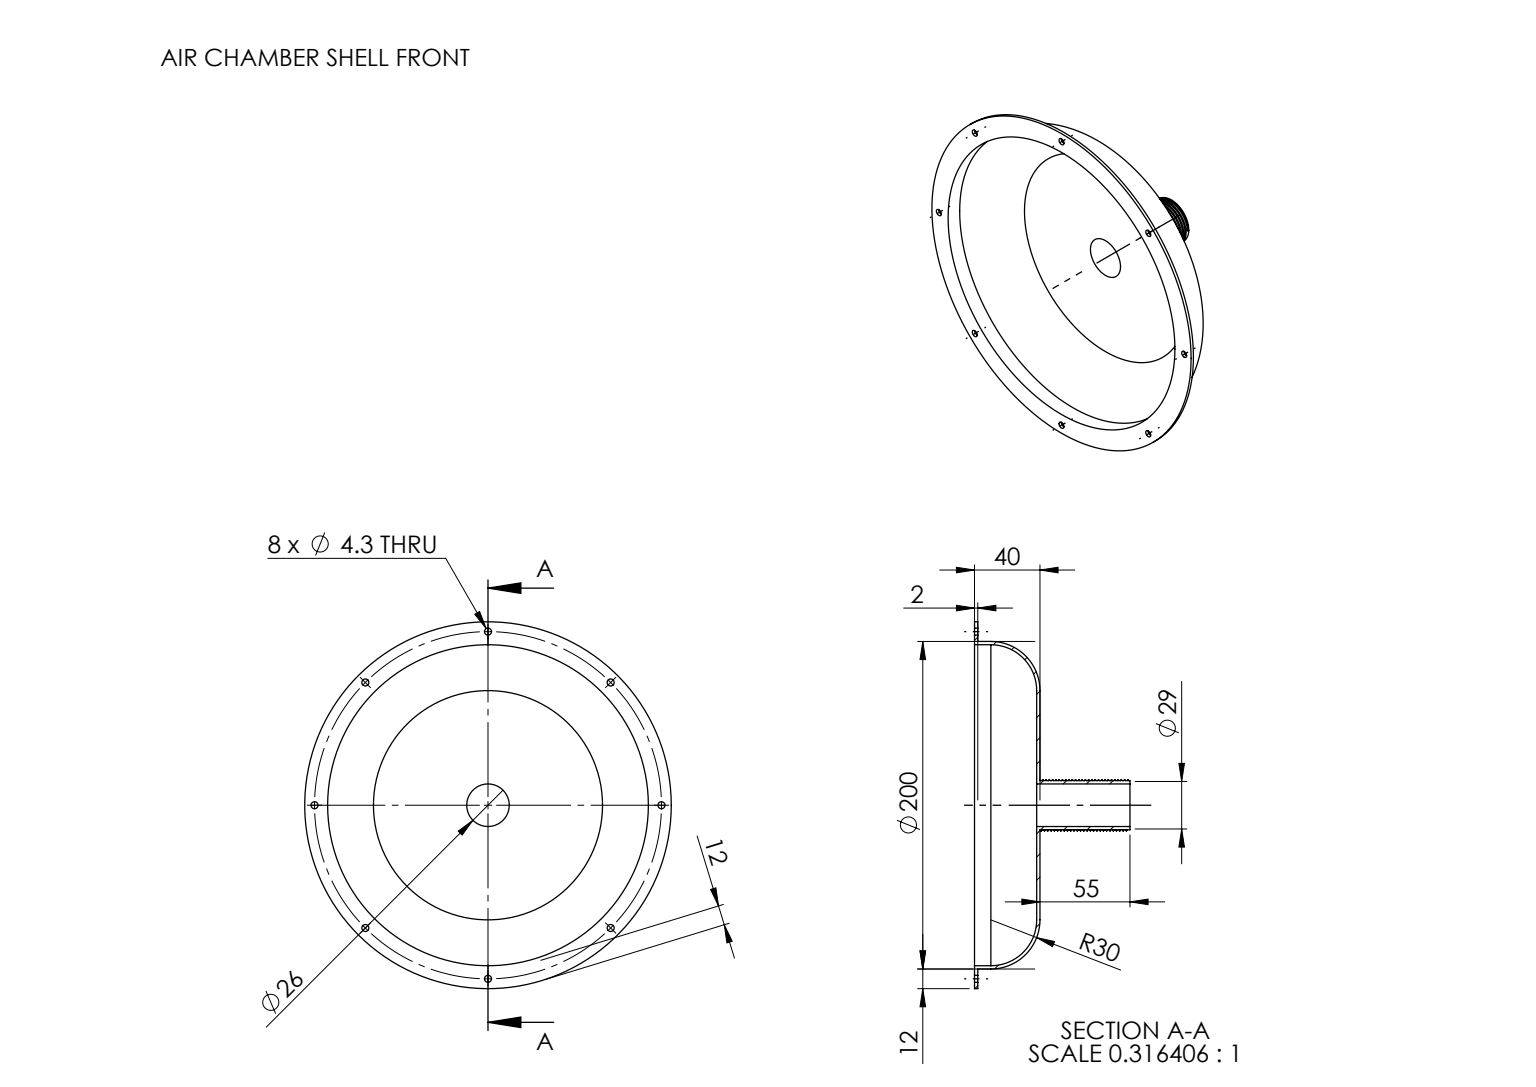
ISO-10303-21;
HEADER;
FILE_DESCRIPTION (('STEP AP214'),
    '1' );
FILE_NAME ('air chamber shell front.step',
    '2026-10-08T07:58:12',
    ( '' ),
    ( '' ),
    'SwSTEP 2.0',
    'SolidWorks 2026',
    '' );
FILE_SCHEMA (( 'AUTOMOTIVE_DESIGN' ));
ENDSEC;

DATA;
#4=DIRECTION ( 'NONE',  ( 0.000000000000000000, 0.000000000000000000, -1.000000000000000000 ) ) ;
#9=CARTESIAN_POINT ( 'NONE',  ( 60.97499999726881015, 140.1801316387863778, -4.815267126137194431 ) ) ;
#11=CARTESIAN_POINT ( 'NONE',  ( 68.68867513459484542, 150.1262045565065364, -15.00000000000012434 ) ) ;
#21=CARTESIAN_POINT ( 'NONE',  ( 33.32499999726881157, 164.1591823560292198, -12.60653300113719766 ) ) ;
#26=CARTESIAN_POINT ( 'NONE',  ( 57.37499999726880873, 155.0000000000000000, -15.58253175000000823 ) ) ;
#30=CARTESIAN_POINT ( 'NONE',  ( 87.72499999726882436, 169.8198683612136222, 4.815267126137181997 ) ) ;
#31=CARTESIAN_POINT ( 'NONE',  ( 41.91132485994280188, 163.8167787843871110, -12.13525491562423397 ) ) ;
#33=CARTESIAN_POINT ( 'NONE',  ( 51.79999999453762882, 146.4771138417591203, -11.73074641843674470 ) ) ;
#39=CARTESIAN_POINT ( 'NONE',  ( 60.11132485994280472, 169.2658477444273331, -4.635254915624224203 ) ) ;
#43=EDGE_CURVE ( 'NONE', #14229, #27576, #23397, .T. ) ;
#46=CARTESIAN_POINT ( 'NONE',  ( 43.71132485994280614, 155.0000000000000000, -15.00000000000002487 ) ) ;
#50=CARTESIAN_POINT ( 'NONE',  ( 42.47499999726881015, 149.9369285172503510, 15.58253174999999580 ) ) ;
#51=ORIENTED_EDGE ( 'NONE', *, *, #2660, .T. ) ;
#52=CARTESIAN_POINT ( 'NONE',  ( 47.92499999726881299, 164.1591823560292198, 12.60653300113718167 ) ) ;
#56=CARTESIAN_POINT ( 'NONE',  ( 50.77499999726880731, 140.1801316387863778, 4.815267126137185549 ) ) ;
#60=CARTESIAN_POINT ( 'NONE',  ( 65.20000000000001705, 167.3344367211045096, 8.961492836873468093 ) ) ;
#67=CARTESIAN_POINT ( 'NONE',  ( 67.92499999726881299, 164.1591823560292198, 12.60653300113718167 ) ) ;
#70=CARTESIAN_POINT ( 'NONE',  ( 37.59999999453762598, 141.2096805137202580, -4.480746418436742040 ) ) ;
#90=CARTESIAN_POINT ( 'NONE',  ( 80.92499999726882720, 145.8408176439707802, -12.60653300113719588 ) ) ;
#91=CARTESIAN_POINT ( 'NONE',  ( 87.50000000000001421, 155.0000000000000000, -6.938893903907228378E-15 ) ) ;
#95=CARTESIAN_POINT ( 'NONE',  ( 50.79999999999999716, 167.3344367211045096, -8.961492836873482304 ) ) ;
#98=CARTESIAN_POINT ( 'NONE',  ( 53.82499999726881157, 168.2552932293087906, 9.630534252274372875 ) ) ;
#102=CARTESIAN_POINT ( 'NONE',  ( 55.42499999726880588, 168.2552932293087906, -9.630534252274387086 ) ) ;
#103=CARTESIAN_POINT ( 'NONE',  ( 67.97499999726881015, 169.8198683612136222, 4.815267126137181997 ) ) ;
#105=CARTESIAN_POINT ( 'NONE',  ( 46.01132485994281041, 167.7597621252805880, -9.270509831248443078 ) ) ;
#108=CARTESIAN_POINT ( 'NONE',  ( 35.38867513459481273, 169.2658477444273331, 4.635254915624208216 ) ) ;
#121=CYLINDRICAL_SURFACE ( 'NONE', #25443, 15.00000000000001776 ) ;
#124=CARTESIAN_POINT ( 'NONE',  ( 70.92499999726881299, 145.8408176439707802, -12.60653300113719588 ) ) ;
#128=CARTESIAN_POINT ( 'NONE',  ( 63.72499999726881015, 169.8198683612136222, 4.815267126137181997 ) ) ;
#137=CARTESIAN_POINT ( 'NONE',  ( 44.78867513459481842, 155.0000000000000000, -15.00000000000002487 ) ) ;
#144=CARTESIAN_POINT ( 'NONE',  ( 40.12499999726880873, 155.0000000000000000, 15.58253174999999402 ) ) ;
#151=CARTESIAN_POINT ( 'NONE',  ( 77.49999999453761745, 139.7537977485451393, -4.138211985947621020E-15 ) ) ;
#155=VECTOR ( 'NONE', #28010, 1000.000000000000000 ) ;
#158=CARTESIAN_POINT ( 'NONE',  ( 48.78867513459482552, 155.0000000000000000, -15.00000000000002487 ) ) ;
#163=CARTESIAN_POINT ( 'NONE',  ( 51.68867513459483831, 159.8737954434934920, 15.00000000000010836 ) ) ;
#170=CARTESIAN_POINT ( 'NONE',  ( 62.97499999726881015, 140.1801316387863778, -4.815267126137194431 ) ) ;
#177=VECTOR ( 'NONE', #7747, 1000.000000000000000 ) ;
#185=CARTESIAN_POINT ( 'NONE',  ( 86.00000000000001421, 139.7537977485451393, -4.138211985947621020E-15 ) ) ;
#186=CARTESIAN_POINT ( 'NONE',  ( 81.68867513459483121, 159.8737954434934920, 15.00000000000010836 ) ) ;
#190=CARTESIAN_POINT ( 'NONE',  ( 59.07499999726880446, 141.7447067706911810, -9.630534252274385310 ) ) ;
#194=CARTESIAN_POINT ( 'NONE',  ( 87.92499999726881299, 164.1591823560292198, 12.60653300113718167 ) ) ;
#197=DIRECTION ( 'NONE',  ( 0.000000000000000000, 0.000000000000000000, -1.000000000000000000 ) ) ;
#198=CARTESIAN_POINT ( 'NONE',  ( 58.39999999453763024, 168.7903194862797420, -4.480746418436745593 ) ) ;
#206=CIRCLE ( 'NONE', #7281, 100.0000000000000284 ) ;
#207=ORIENTED_EDGE ( 'NONE', *, *, #12087, .F. ) ;
#215=CARTESIAN_POINT ( 'NONE',  ( 43.97499999726881015, 169.8198683612136222, 4.815267126137181997 ) ) ;
#216=ORIENTED_EDGE ( 'NONE', *, *, #22229, .T. ) ;
#217=CARTESIAN_POINT ( 'NONE',  ( 53.12499999726881583, 155.0000000000000000, -15.58253175000000823 ) ) ;
#223=CARTESIAN_POINT ( 'NONE',  ( 53.77499999726881441, 169.8198683612136222, -4.815267126137197984 ) ) ;
#229=CARTESIAN_POINT ( 'NONE',  ( 67.70000000000001705, 146.4771138417591203, 11.73074641843673227 ) ) ;
#234=CARTESIAN_POINT ( 'NONE',  ( 37.97499999726881015, 169.8198683612136222, 4.815267126137181997 ) ) ;
#238=CARTESIAN_POINT ( 'NONE',  ( 69.42499999726881299, 168.2552932293087906, -9.630534252274385310 ) ) ;
#241=CARTESIAN_POINT ( 'NONE',  ( 39.59999999453763309, 141.2096805137202580, -4.480746418436742040 ) ) ;
#255=ADVANCED_FACE ( 'NONE', ( #21810 ), #32041, .T. ) ;
#257=CARTESIAN_POINT ( 'NONE',  ( 55.81132485994281467, 159.8737954434936057, -15.00000000000002665 ) ) ;
#260=CARTESIAN_POINT ( 'NONE',  ( 86.72499999726882436, 140.1801316387863778, -4.815267126137194431 ) ) ;
#261=FACE_OUTER_BOUND ( 'NONE', #4301, .T. ) ;
#265=CARTESIAN_POINT ( 'NONE',  ( 49.50000000000000000, 155.0000000000000000, 14.49999999999999467 ) ) ;
#267=CARTESIAN_POINT ( 'NONE',  ( 125.5000000000000000, 229.9533188057749555, 74.95331880577313655 ) ) ;
#268=CARTESIAN_POINT ( 'NONE',  ( 50.62499999726880162, 138.6155565068815463, -3.929120461958505118E-15 ) ) ;
#270=CARTESIAN_POINT ( 'NONE',  ( 61.02499999726880020, 149.9369285172503510, -15.58253175000000823 ) ) ;
#271=CARTESIAN_POINT ( 'NONE',  ( 72.47499999726878173, 149.9369285172503510, 15.58253174999999580 ) ) ;
#275=CARTESIAN_POINT ( 'NONE',  ( 125.5000000000000000, 48.99999999999998579, 2.149999999999971489 ) ) ;
#287=ORIENTED_EDGE ( 'NONE', *, *, #8864, .T. ) ;
#288=CARTESIAN_POINT ( 'NONE',  ( 75.92499999726881299, 164.1591823560292198, 12.60653300113718167 ) ) ;
#291=CARTESIAN_POINT ( 'NONE',  ( 67.82499999726881867, 168.2552932293087906, 9.630534252274372875 ) ) ;
#295=DIRECTION ( 'NONE',  ( 1.000000000000000000, 0.000000000000000000, 0.000000000000000000 ) ) ;
#298=FACE_BOUND ( 'NONE', #1357, .T. ) ;
#305=CARTESIAN_POINT ( 'NONE',  ( 44.22499999726880304, 149.9369285172503510, 15.58253174999999580 ) ) ;
#312=CARTESIAN_POINT ( 'NONE',  ( 80.39999999453763735, 168.7903194862797420, -4.480746418436745593 ) ) ;
#317=VERTEX_POINT ( 'NONE', #1197 ) ;
#324=EDGE_CURVE ( 'NONE', #6936, #7786, #8863, .T. ) ;
#327=CARTESIAN_POINT ( 'NONE',  ( 63.57499999726881867, 164.1591823560292198, -12.60653300113719766 ) ) ;
#337=CARTESIAN_POINT ( 'NONE',  ( 84.47499999726881015, 149.9369285172503510, 15.58253174999999580 ) ) ;
#340=CARTESIAN_POINT ( 'NONE',  ( 38.12499999726880873, 155.0000000000000000, 15.58253174999999402 ) ) ;
#342=LINE ( 'NONE', #30862, #5985 ) ;
#344=EDGE_CURVE ( 'NONE', #21593, #16276, #11595, .T. ) ;
#346=CARTESIAN_POINT ( 'NONE',  ( 58.17499999726881299, 164.1591823560292198, 12.60653300113718167 ) ) ;
#351=EDGE_CURVE ( 'NONE', #31779, #31412, #28685, .T. ) ;
#352=CARTESIAN_POINT ( 'NONE',  ( 78.61132485994281183, 159.8737954434936057, 15.00000000000001421 ) ) ;
#354=CARTESIAN_POINT ( 'NONE',  ( 62.09999999453761887, 159.7113355953771077, -14.50000000000000888 ) ) ;
#357=CARTESIAN_POINT ( 'NONE',  ( 77.31132485994280046, 140.7341522555726669, -4.635254915624220651 ) ) ;
#359=CARTESIAN_POINT ( 'NONE',  ( 71.28867513459483973, 170.7719333635740497, -7.904646289410545231E-15 ) ) ;
#363=EDGE_LOOP ( 'NONE', ( #22893, #12184, #17028, #24574 ) ) ;
#364=CARTESIAN_POINT ( 'NONE',  ( 44.11132485994280472, 169.2658477444273331, -4.635254915624224203 ) ) ;
#370=CARTESIAN_POINT ( 'NONE',  ( 45.47499999726881015, 160.0630714827496206, -15.58253175000000823 ) ) ;
#372=CARTESIAN_POINT ( 'NONE',  ( 51.32499999726881157, 164.1591823560292198, -12.60653300113719766 ) ) ;
#377=CARTESIAN_POINT ( 'NONE',  ( 51.67499999726879878, 168.2552932293087906, -9.630534252274385310 ) ) ;
#378=CARTESIAN_POINT ( 'NONE',  ( 32.50000000000000000, 155.0000000000000000, 15.00000000000001243 ) ) ;
#383=CARTESIAN_POINT ( 'NONE',  ( 75.40000000000000568, 159.7113355953771077, 14.49999999999999289 ) ) ;
#387=CARTESIAN_POINT ( 'NONE',  ( 86.48867513459484258, 142.2402378747194405, -9.270509831248439525 ) ) ;
#388=CARTESIAN_POINT ( 'NONE',  ( 37.37499999726881583, 155.0000000000000000, -15.58253175000000823 ) ) ;
#390=CARTESIAN_POINT ( 'NONE',  ( 71.72499999726881015, 169.8198683612136222, 4.815267126137181997 ) ) ;
#393=CARTESIAN_POINT ( 'NONE',  ( 38.49999999453763166, 170.2462022514548323, -7.872454543227099337E-15 ) ) ;
#398=ORIENTED_EDGE ( 'NONE', *, *, #15560, .F. ) ;
#405=EDGE_CURVE ( 'NONE', #7596, #17895, #14227, .T. ) ;
#411=ADVANCED_FACE ( 'NONE', ( #12099 ), #20103, .F. ) ;
#415=CARTESIAN_POINT ( 'NONE',  ( 34.42499999726880588, 141.7447067706911810, 9.630534252274376428 ) ) ;
#417=CARTESIAN_POINT ( 'NONE',  ( 33.67499999726881299, 168.2552932293087906, -9.630534252274385310 ) ) ;
#420=VECTOR ( 'NONE', #14402, 1000.000000000000000 ) ;
#422=CARTESIAN_POINT ( 'NONE',  ( 45.70000000000000284, 146.4771138417591203, 11.73074641843673227 ) ) ;
#426=CARTESIAN_POINT ( 'NONE',  ( 51.12499999726881583, 155.0000000000000000, -15.58253175000000823 ) ) ;
#430=CARTESIAN_POINT ( 'NONE',  ( 66.72499999726881015, 140.1801316387863778, -4.815267126137194431 ) ) ;
#431=CARTESIAN_POINT ( 'NONE',  ( 78.67499999726879878, 141.7447067706911810, 9.630534252274376428 ) ) ;
#455=( BOUNDED_CURVE ( )  B_SPLINE_CURVE ( 2, ( #7550, #25926, #18262, #23205, #4981, #21145, #13149, #539, #28652, #5312, #17936 ),
 .UNSPECIFIED., .F., .F. ) 
 B_SPLINE_CURVE_WITH_KNOTS ( ( 3, 2, 2, 2, 2, 3 ),
 ( 0.1249999999999998473, 0.1285714285714284200, 0.1321428571428569787, 0.1357142857142855652, 0.1392857142857141239, 0.1428571428571427104 ),
 .UNSPECIFIED. ) 
 CURVE ( )  GEOMETRIC_REPRESENTATION_ITEM ( )  RATIONAL_B_SPLINE_CURVE ( ( 1.000000000000002220, 0.9510565162951514218, 1.000000000000000000, 0.9510565162951534202, 1.000000000000000000, 0.9510565162951534202, 1.000000000000000000, 0.9510565162951534202, 1.000000000000000000, 0.9510565162951545304, 0.9999999999999988898 ) ) 
 REPRESENTATION_ITEM ( '' )  );
#457=CARTESIAN_POINT ( 'NONE',  ( 80.42499999726881299, 141.7447067706911810, 9.630534252274376428 ) ) ;
#460=CARTESIAN_POINT ( 'NONE',  ( 69.02499999726880731, 149.9369285172503510, -15.58253175000000823 ) ) ;
#463=CYLINDRICAL_SURFACE ( 'NONE', #17578, 15.00000000000001776 ) ;
#475=CARTESIAN_POINT ( 'NONE',  ( 60.48867513459483547, 142.2402378747194405, -9.270509831248439525 ) ) ;
#476=CARTESIAN_POINT ( 'NONE',  ( 42.52499999726880731, 140.1801316387863778, 4.815267126137185549 ) ) ;
#484=CARTESIAN_POINT ( 'NONE',  ( 79.79999999453762882, 146.4771138417591203, -11.73074641843674470 ) ) ;
#494=CARTESIAN_POINT ( 'NONE',  ( 77.47499999726879594, 160.0630714827496206, -15.58253175000000823 ) ) ;
#500=FILL_AREA_STYLE_COLOUR ( '', #2004 ) ;
#502=CARTESIAN_POINT ( 'NONE',  ( 63.27499999726880731, 149.9369285172503510, -15.58253175000000823 ) ) ;
#503=AXIS2_PLACEMENT_3D ( 'NONE', #32929, #27646, #1421 ) ;
#507=( BOUNDED_CURVE ( )  B_SPLINE_CURVE ( 2, ( #4951, #13282, #18065, #5118, #18402, #10250, #10735, #28626, #5613 ),
 .UNSPECIFIED., .F., .T. ) 
 B_SPLINE_CURVE_WITH_KNOTS ( ( 3, 2, 2, 2, 3 ),
 ( 0.9464285714285716189, 0.9500000000000000666, 0.9535714285714287364, 0.9571428571428571841, 0.9605034456745119575 ),
 .UNSPECIFIED. ) 
 CURVE ( )  GEOMETRIC_REPRESENTATION_ITEM ( )  RATIONAL_B_SPLINE_CURVE ( ( 0.9999999999999970024, 0.9510565162951564178, 1.000000000000000000, 0.9510565162951534202, 1.000000000000000000, 0.9510565162951534202, 1.000000000000000000, 0.9539459051894326747, 0.9945623735783009067 ) ) 
 REPRESENTATION_ITEM ( '' )  );
#513=CARTESIAN_POINT ( 'NONE',  ( 83.97499999726882436, 169.8198683612136222, 4.815267126137181997 ) ) ;
#516=CARTESIAN_POINT ( 'NONE',  ( 41.42499999726881299, 168.2552932293087906, -9.630534252274385310 ) ) ;
#522=CARTESIAN_POINT ( 'NONE',  ( 57.07499999726879736, 141.7447067706911810, -9.630534252274385310 ) ) ;
#526=CARTESIAN_POINT ( 'NONE',  ( 55.78867513459481842, 155.0000000000000000, 15.00000000000001243 ) ) ;
#528=CARTESIAN_POINT ( 'NONE',  ( 60.59999999453763309, 168.7903194862797420, 4.480746418436729606 ) ) ;
#533=CARTESIAN_POINT ( 'NONE',  ( 71.58867513459482268, 163.8167787843871110, 12.13525491562421621 ) ) ;
#534=VERTEX_POINT ( 'NONE', #12264 ) ;
#537=EDGE_CURVE ( 'NONE', #27429, #2840, #9457, .T. ) ;
#538=CARTESIAN_POINT ( 'NONE',  ( 125.5000000000000000, 229.9533188057739039, -74.95331880577418815 ) ) ;
#539=CARTESIAN_POINT ( 'NONE',  ( 80.08867513459485110, 142.2402378747194405, 9.270509831248432420 ) ) ;
#543=DIRECTION ( 'NONE',  ( -1.000000000000000000, 0.000000000000000000, 0.000000000000000000 ) ) ;
#545=CARTESIAN_POINT ( 'NONE',  ( 45.07499999726879736, 141.7447067706911810, -9.630534252274387086 ) ) ;
#547=CARTESIAN_POINT ( 'NONE',  ( 48.62499999726880873, 138.6155565068815463, -3.929120461958505118E-15 ) ) ;
#549=CARTESIAN_POINT ( 'NONE',  ( 61.68867513459483121, 159.8737954434936057, 15.00000000000001421 ) ) ;
#551=CARTESIAN_POINT ( 'NONE',  ( 56.27499999726880020, 160.0630714827496206, 15.58253174999999402 ) ) ;
#554=CARTESIAN_POINT ( 'NONE',  ( 74.30000000000001137, 146.4771138417591203, -11.73074641843674470 ) ) ;
#556=CARTESIAN_POINT ( 'NONE',  ( 127.5000000000000000, 155.0000000000000000, -6.938893903907228378E-15 ) ) ;
#558=CARTESIAN_POINT ( 'NONE',  ( 33.28867513459482552, 170.7719333635740497, -7.904646289410545231E-15 ) ) ;
#559=CARTESIAN_POINT ( 'NONE',  ( 36.17499999726880588, 164.1591823560292198, 12.60653300113718167 ) ) ;
#561=CARTESIAN_POINT ( 'NONE',  ( 75.12499999726881583, 155.0000000000000000, -15.58253175000000823 ) ) ;
#562=VERTEX_POINT ( 'NONE', #4088 ) ;
#564=CARTESIAN_POINT ( 'NONE',  ( 42.69999999453762030, 167.3344367211045096, 8.961492836873468093 ) ) ;
#565=CARTESIAN_POINT ( 'NONE',  ( 39.81132485994280756, 159.8737954434936057, -15.00000000000005151 ) ) ;
#575=CARTESIAN_POINT ( 'NONE',  ( 73.78867513459483973, 155.0000000000000000, 15.00000000000001243 ) ) ;
#581=FACE_OUTER_BOUND ( 'NONE', #26390, .T. ) ;
#583=CARTESIAN_POINT ( 'NONE',  ( 87.12499999726880162, 155.0000000000000000, -15.58253175000000823 ) ) ;
#584=DIRECTION ( 'NONE',  ( -1.000000000000000000, 0.000000000000000000, 0.000000000000000000 ) ) ;
#587=CARTESIAN_POINT ( 'NONE',  ( 55.79999999999999716, 142.6655632788954620, 8.961492836873471646 ) ) ;
#589=DIRECTION ( 'NONE',  ( 1.000000000000000000, 0.000000000000000000, 0.000000000000000000 ) ) ;
#591=CARTESIAN_POINT ( 'NONE',  ( 60.22499999726881725, 149.9369285172503510, 15.58253174999999580 ) ) ;
#594=CARTESIAN_POINT ( 'NONE',  ( 61.92499999726882010, 164.1591823560292198, 12.60653300113718167 ) ) ;
#595=CARTESIAN_POINT ( 'NONE',  ( 73.97499999726881015, 169.8198683612136222, 4.815267126137181997 ) ) ;
#597=CARTESIAN_POINT ( 'NONE',  ( 32.50000000000000000, 155.0000000000000000, -6.938893903907228378E-15 ) ) ;
#601=ORIENTED_EDGE ( 'NONE', *, *, #25333, .F. ) ;
#608=VERTEX_POINT ( 'NONE', #7674 ) ;
#614=CARTESIAN_POINT ( 'NONE',  ( 79.42499999726881299, 168.2552932293087906, -9.630534252274387086 ) ) ;
#616=CARTESIAN_POINT ( 'NONE',  ( 69.78867513459482552, 155.0000000000000000, 15.00000000000001243 ) ) ;
#620=CARTESIAN_POINT ( 'NONE',  ( 71.82499999726883289, 168.2552932293087906, 9.630534252274372875 ) ) ;
#626=CARTESIAN_POINT ( 'NONE',  ( 34.20000000000000284, 142.6655632788954620, -8.961492836873480528 ) ) ;
#629=EDGE_CURVE ( 'NONE', #11212, #17245, #20101, .T. ) ;
#634=CARTESIAN_POINT ( 'NONE',  ( 45.42499999726880588, 168.2552932293087906, -9.630534252274387086 ) ) ;
#636=CARTESIAN_POINT ( 'NONE',  ( 127.5000000000000000, 155.0000000000000000, -112.0000000000000711 ) ) ;
#643=CARTESIAN_POINT ( 'NONE',  ( 79.89999999453763735, 150.2886644046228639, -14.50000000000000888 ) ) ;
#654=CARTESIAN_POINT ( 'NONE',  ( 74.47499999726881015, 149.9369285172503510, 15.58253174999999580 ) ) ;
#655=CARTESIAN_POINT ( 'NONE',  ( 53.11132485994280472, 140.7341522555726669, 4.635254915624211769 ) ) ;
#656=CARTESIAN_POINT ( 'NONE',  ( 59.58867513459482979, 163.8167787843871110, 12.13525491562421621 ) ) ;
#658=PRESENTATION_STYLE_ASSIGNMENT (( #994 ) ) ;
#660=CARTESIAN_POINT ( 'NONE',  ( 68.17499999726881299, 164.1591823560292198, 12.60653300113718167 ) ) ;
#661=ORIENTED_EDGE ( 'NONE', *, *, #43, .F. ) ;
#664=CARTESIAN_POINT ( 'NONE',  ( 43.58867513459482979, 163.8167787843871110, 12.13525491562421621 ) ) ;
#669=CARTESIAN_POINT ( 'NONE',  ( 87.57499999726880446, 164.1591823560292198, -12.60653300113719766 ) ) ;
#674=CARTESIAN_POINT ( 'NONE',  ( 40.02499999726881441, 160.0630714827496206, 15.58253174999999402 ) ) ;
#675=CARTESIAN_POINT ( 'NONE',  ( 67.78867513459482552, 155.0000000000000000, 15.00000000000001243 ) ) ;
#679=CARTESIAN_POINT ( 'NONE',  ( 55.77499999726881441, 169.8198683612136222, -4.815267126137197984 ) ) ;
#685=CARTESIAN_POINT ( 'NONE',  ( 62.29999999453762172, 167.3344367211045096, -8.961492836873482304 ) ) ;
#695=CARTESIAN_POINT ( 'NONE',  ( 117.5000000000000142, 155.0000000000000000, 100.0000000000000284 ) ) ;
#704=CARTESIAN_POINT ( 'NONE',  ( 44.67499999726881299, 141.7447067706911810, 9.630534252274376428 ) ) ;
#706=CARTESIAN_POINT ( 'NONE',  ( 49.02499999726880731, 149.9369285172503510, -15.58253175000000823 ) ) ;
#708=CARTESIAN_POINT ( 'NONE',  ( 61.58867513459482979, 163.8167787843871110, 12.13525491562421621 ) ) ;
#711=CARTESIAN_POINT ( 'NONE',  ( 55.67499999726879878, 168.2552932293087906, -9.630534252274385310 ) ) ;
#716=CARTESIAN_POINT ( 'NONE',  ( 73.40000000000000568, 159.7113355953771077, 14.49999999999999289 ) ) ;
#717=CARTESIAN_POINT ( 'NONE',  ( 64.98867513459482836, 163.8167787843871110, -12.13525491562423397 ) ) ;
#720=DIRECTION ( 'NONE',  ( 0.000000000000000000, -0.7071067811865506814, -0.7071067811865442421 ) ) ;
#721=CARTESIAN_POINT ( 'NONE',  ( 35.77499999726881441, 169.8198683612136222, -4.815267126137197984 ) ) ;
#725=CARTESIAN_POINT ( 'NONE',  ( 79.92499999726881299, 164.1591823560292198, 12.60653300113718167 ) ) ;
#729=CARTESIAN_POINT ( 'NONE',  ( 42.29999999453763593, 167.3344367211045096, -8.961492836873482304 ) ) ;
#741=AXIS2_PLACEMENT_3D ( 'NONE', #7083, #30078, #6742 ) ;
#744=EDGE_CURVE ( 'NONE', #14095, #15702, #8660, .T. ) ;
#750=CARTESIAN_POINT ( 'NONE',  ( 36.87499999726881583, 138.6155565068815463, -3.929120461958505118E-15 ) ) ;
#754=CARTESIAN_POINT ( 'NONE',  ( 53.19999999999998863, 167.3344367211045096, 8.961492836873468093 ) ) ;
#757=EDGE_CURVE ( 'NONE', #31949, #12310, #32158, .T. ) ;
#758=CARTESIAN_POINT ( 'NONE',  ( 55.22499999726880304, 160.0630714827496206, -15.58253175000000823 ) ) ;
#760=CARTESIAN_POINT ( 'NONE',  ( 37.51132485994280330, 146.1832212156128890, -12.13525491562423042 ) ) ;
#761=CARTESIAN_POINT ( 'NONE',  ( 62.72499999726881015, 140.1801316387863778, -4.815267126137194431 ) ) ;
#762=CARTESIAN_POINT ( 'NONE',  ( 76.87499999726881583, 138.6155565068815463, -3.929120461958505118E-15 ) ) ;
#772=CIRCLE ( 'NONE', #14370, 2.149999999999994138 ) ;
#785=CARTESIAN_POINT ( 'NONE',  ( 76.12499999726881583, 155.0000000000000000, 15.58253174999999402 ) ) ;
#786=ORIENTED_EDGE ( 'NONE', *, *, #16132, .F. ) ;
#789=MANIFOLD_SOLID_BREP ( 'CirPattern1', #11241 ) ;
#792=CARTESIAN_POINT ( 'NONE',  ( 70.02499999726879309, 160.0630714827496206, 15.58253174999999402 ) ) ;
#796=CARTESIAN_POINT ( 'NONE',  ( 33.59999999999998721, 150.2886644046228639, 14.49999999999999645 ) ) ;
#802=CARTESIAN_POINT ( 'NONE',  ( 125.5000000000000000, 228.4330392262228600, -76.47359838532526055 ) ) ;
#804=CARTESIAN_POINT ( 'NONE',  ( 45.02499999726881441, 149.9369285172503510, -15.58253175000000823 ) ) ;
#811=CARTESIAN_POINT ( 'NONE',  ( 87.99999999453763166, 155.0000000000000000, -14.50000000000000711 ) ) ;
#819=ORIENTED_EDGE ( 'NONE', *, *, #16423, .F. ) ;
#821=ORIENTED_EDGE ( 'NONE', *, *, #24714, .F. ) ;
#822=EDGE_CURVE ( 'NONE', #562, #11454, #3119, .T. ) ;
#823=CARTESIAN_POINT ( 'NONE',  ( 75.67499999726881299, 168.2552932293087906, -9.630534252274387086 ) ) ;
#825=CARTESIAN_POINT ( 'NONE',  ( 58.78867513459481842, 155.0000000000000000, -15.00000000000002487 ) ) ;
#829=CARTESIAN_POINT ( 'NONE',  ( 70.97499999726881015, 140.1801316387863778, -4.815267126137194431 ) ) ;
#836=CARTESIAN_POINT ( 'NONE',  ( 83.78867513459482552, 155.0000000000000000, 15.00000000000001243 ) ) ;
#838=CARTESIAN_POINT ( 'NONE',  ( 85.07499999726880446, 141.7447067706911810, -9.630534252274385310 ) ) ;
#841=CARTESIAN_POINT ( 'NONE',  ( 39.42499999726881299, 168.2552932293087906, -9.630534252274385310 ) ) ;
#842=CARTESIAN_POINT ( 'NONE',  ( 36.68867513459482410, 150.1262045565068206, -15.00000000000030909 ) ) ;
#843=DIRECTION ( 'NONE',  ( 0.000000000000000000, 0.7071067811865442421, -0.7071067811865506814 ) ) ;
#845=CARTESIAN_POINT ( 'NONE',  ( 33.37499999726880873, 155.0000000000000000, -15.58253175000000823 ) ) ;
#846=CARTESIAN_POINT ( 'NONE',  ( 63.07499999726881867, 141.7447067706911810, -9.630534252274385310 ) ) ;
#853=CARTESIAN_POINT ( 'NONE',  ( 63.29999999453762882, 142.6655632788954620, 8.961492836873471646 ) ) ;
#856=CARTESIAN_POINT ( 'NONE',  ( 77.01132485994283172, 142.2402378747194405, 9.270509831248432420 ) ) ;
#859=CARTESIAN_POINT ( 'NONE',  ( 72.01132485994281751, 167.7597621252805880, -9.270509831248443078 ) ) ;
#865=DIRECTION ( 'NONE',  ( 1.000000000000000000, 0.000000000000000000, 0.000000000000000000 ) ) ;
#870=CARTESIAN_POINT ( 'NONE',  ( 51.47499999726881725, 160.0630714827496206, -15.58253175000000823 ) ) ;
#872=CARTESIAN_POINT ( 'NONE',  ( 60.02499999726880020, 160.0630714827496206, 15.58253174999999402 ) ) ;
#875=DIRECTION ( 'NONE',  ( 0.000000000000000000, 0.000000000000000000, -1.000000000000000000 ) ) ;
#877=CARTESIAN_POINT ( 'NONE',  ( 59.17499999726881299, 145.8408176439707802, -12.60653300113719588 ) ) ;
#882=CARTESIAN_POINT ( 'NONE',  ( 74.09999999999999432, 141.2096805137202580, -4.480746418436742040 ) ) ;
#886=CARTESIAN_POINT ( 'NONE',  ( 40.77499999726881441, 140.1801316387863778, 4.815267126137185549 ) ) ;
#888=CARTESIAN_POINT ( 'NONE',  ( 75.32499999726881867, 164.1591823560292198, -12.60653300113719766 ) ) ;
#891=CARTESIAN_POINT ( 'NONE',  ( 41.99999999453763166, 155.0000000000000000, -14.50000000000000711 ) ) ;
#893=CARTESIAN_POINT ( 'NONE',  ( 40.71132485994280614, 155.0000000000000000, 15.00000000000001243 ) ) ;
#904=CARTESIAN_POINT ( 'NONE',  ( 127.5000000000000000, 155.0000000000000000, -6.938893903907228378E-15 ) ) ;
#911=CARTESIAN_POINT ( 'NONE',  ( 37.02499999726880020, 149.9369285172503510, -15.58253175000000823 ) ) ;
#913=CARTESIAN_POINT ( 'NONE',  ( 88.02499999726880731, 160.0630714827496206, 15.58253174999999402 ) ) ;
#914=DIRECTION ( 'NONE',  ( 0.000000000000000000, 1.000000000000000000, -6.454785026890489601E-15 ) ) ;
#917=CARTESIAN_POINT ( 'NONE',  ( 55.10000000000000142, 168.7903194862797420, 4.480746418436729606 ) ) ;
#921=CARTESIAN_POINT ( 'NONE',  ( 55.82499999726880446, 168.2552932293087906, 9.630534252274372875 ) ) ;
#926=CARTESIAN_POINT ( 'NONE',  ( 65.12499999726881583, 155.0000000000000000, -15.58253175000000823 ) ) ;
#927=CARTESIAN_POINT ( 'NONE',  ( 73.47499999726878173, 160.0630714827496206, -15.58253175000000823 ) ) ;
#939=ORIENTED_EDGE ( 'NONE', *, *, #757, .F. ) ;
#940=CARTESIAN_POINT ( 'NONE',  ( 63.21132485994281325, 139.2280666364260071, -4.041636747397287284E-15 ) ) ;
#941=ORIENTED_EDGE ( 'NONE', *, *, #22042, .T. ) ;
#947=CARTESIAN_POINT ( 'NONE',  ( 74.82499999726881867, 141.7447067706911810, -9.630534252274387086 ) ) ;
#952=CARTESIAN_POINT ( 'NONE',  ( 67.22499999726879594, 160.0630714827496206, -15.58253175000000823 ) ) ;
#957=CARTESIAN_POINT ( 'NONE',  ( 35.20000000000000284, 167.3344367211045096, 8.961492836873468093 ) ) ;
#965=CARTESIAN_POINT ( 'NONE',  ( 44.42499999726881299, 141.7447067706911810, 9.630534252274376428 ) ) ;
#972=CIRCLE ( 'NONE', #14031, 13.00000000000001776 ) ;
#975=CARTESIAN_POINT ( 'NONE',  ( 85.69999999453762030, 142.6655632788954620, -8.961492836873480528 ) ) ;
#985=CARTESIAN_POINT ( 'NONE',  ( 70.47499999726881015, 149.9369285172503510, 15.58253174999999580 ) ) ;
#988=ADVANCED_FACE ( 'NONE', ( #4564 ), #7120, .F. ) ;
#989=CARTESIAN_POINT ( 'NONE',  ( 80.17499999726881299, 164.1591823560292198, 12.60653300113718167 ) ) ;
#994=SURFACE_STYLE_USAGE ( .BOTH. , #19219 ) ;
#997=CARTESIAN_POINT ( 'NONE',  ( 70.77499999726880731, 140.1801316387863778, 4.815267126137185549 ) ) ;
#1007=CARTESIAN_POINT ( 'NONE',  ( 84.67499999726881299, 141.7447067706911810, 9.630534252274376428 ) ) ;
#1010=CARTESIAN_POINT ( 'NONE',  ( 35.52499999726880731, 169.8198683612136222, -4.815267126137197984 ) ) ;
#1011=CARTESIAN_POINT ( 'NONE',  ( 81.18867513459481700, 169.2658477444273331, -4.635254915624224203 ) ) ;
#1015=EDGE_CURVE ( 'NONE', #20912, #20942, #22442, .T. ) ;
#1023=CARTESIAN_POINT ( 'NONE',  ( 66.99999999453761745, 155.0000000000000000, 14.49999999999999467 ) ) ;
#1031=CARTESIAN_POINT ( 'NONE',  ( 45.01132485994281751, 142.2402378747194405, 9.270509831248432420 ) ) ;
#1043=CARTESIAN_POINT ( 'NONE',  ( 48.77499999726880731, 140.1801316387863778, 4.815267126137185549 ) ) ;
#1045=CARTESIAN_POINT ( 'NONE',  ( 54.42499999726881299, 141.7447067706911810, 9.630534252274376428 ) ) ;
#1051=CARTESIAN_POINT ( 'NONE',  ( 59.27499999726882152, 149.9369285172503510, -15.58253175000000823 ) ) ;
#1057=CARTESIAN_POINT ( 'NONE',  ( 73.59999999999999432, 150.2886644046228639, 14.49999999999999645 ) ) ;
#1058=CARTESIAN_POINT ( 'NONE',  ( 64.88867513459483405, 159.8737954434937478, -14.99999999999993072 ) ) ;
#1059=DIRECTION ( 'NONE',  ( 0.000000000000000000, 0.000000000000000000, -1.000000000000000000 ) ) ;
#1061=CARTESIAN_POINT ( 'NONE',  ( 125.5000000000000000, 261.0000000000000000, -2.149999999999985256 ) ) ;
#1062=CARTESIAN_POINT ( 'NONE',  ( 45.27499999726880020, 149.9369285172503510, -15.58253175000000823 ) ) ;
#1065=CARTESIAN_POINT ( 'NONE',  ( 75.22499999726879594, 160.0630714827496206, -15.58253175000000823 ) ) ;
#1066=ORIENTED_EDGE ( 'NONE', *, *, #8262, .F. ) ;
#1068=CARTESIAN_POINT ( 'NONE',  ( 46.69999999453762740, 167.3344367211045096, 8.961492836873468093 ) ) ;
#1086=CARTESIAN_POINT ( 'NONE',  ( 37.12499999726881583, 155.0000000000000000, -15.58253175000000823 ) ) ;
#1087=( BOUNDED_CURVE ( )  B_SPLINE_CURVE ( 2, ( #26892, #27390, #29787, #3549, #18445, #26273, #6096, #6453, #1339, #13942, #32335 ),
 .UNSPECIFIED., .F., .F. ) 
 B_SPLINE_CURVE_WITH_KNOTS ( ( 3, 2, 2, 2, 2, 3 ),
 ( 0.6249999999999996669, 0.6285714285714282257, 0.6321428571428568954, 0.6357142857142854542, 0.6392857142857141239, 0.6428571428571426827 ),
 .UNSPECIFIED. ) 
 CURVE ( )  GEOMETRIC_REPRESENTATION_ITEM ( )  RATIONAL_B_SPLINE_CURVE ( ( 1.000000000000004663, 0.9510565162951488682, 1.000000000000000000, 0.9510565162951534202, 1.000000000000000000, 0.9510565162951534202, 1.000000000000000000, 0.9510565162951534202, 1.000000000000000000, 0.9510565162951549745, 0.9999999999999984457 ) ) 
 REPRESENTATION_ITEM ( '' )  );
#1089=CARTESIAN_POINT ( 'NONE',  ( 42.87499999726881583, 138.6155565068815463, -3.929120461958505118E-15 ) ) ;
#1092=CARTESIAN_POINT ( 'NONE',  ( 56.59999999999999432, 159.7113355953771077, -14.50000000000000888 ) ) ;
#1096=CARTESIAN_POINT ( 'NONE',  ( 54.71132485994280614, 155.0000000000000000, 15.00000000000001243 ) ) ;
#1098=CARTESIAN_POINT ( 'NONE',  ( 58.02499999726880731, 160.0630714827496206, 15.58253174999999402 ) ) ;
#1101=CARTESIAN_POINT ( 'NONE',  ( 67.62499999726881583, 171.3844434931184253, -7.942151717890134290E-15 ) ) ;
#1102=CARTESIAN_POINT ( 'NONE',  ( 73.57499999726880446, 164.1591823560292198, -12.60653300113719766 ) ) ;
#1114=ORIENTED_EDGE ( 'NONE', *, *, #11237, .F. ) ;
#1121=CARTESIAN_POINT ( 'NONE',  ( 86.82499999726879025, 141.7447067706911810, -9.630534252274387086 ) ) ;
#1123=CARTESIAN_POINT ( 'NONE',  ( 68.78867513459482552, 155.0000000000000000, -15.00000000000002487 ) ) ;
#1124=CARTESIAN_POINT ( 'NONE',  ( 76.72499999726881015, 140.1801316387863778, -4.815267126137194431 ) ) ;
#1126=CARTESIAN_POINT ( 'NONE',  ( 74.88867513459483405, 159.8737954434939184, -14.99999999999981704 ) ) ;
#1127=FACE_OUTER_BOUND ( 'NONE', #9365, .T. ) ;
#1134=CARTESIAN_POINT ( 'NONE',  ( 117.5000000000000142, 155.0000000000000000, 98.00000000000000000 ) ) ;
#1135=CARTESIAN_POINT ( 'NONE',  ( 50.22499999726881015, 149.9369285172503510, 15.58253174999999580 ) ) ;
#1143=CARTESIAN_POINT ( 'NONE',  ( 83.79999999453762882, 146.4771138417591203, -11.73074641843674470 ) ) ;
#1152=CARTESIAN_POINT ( 'NONE',  ( 73.67499999726878457, 168.2552932293087906, -9.630534252274385310 ) ) ;
#1154=ORIENTED_EDGE ( 'NONE', *, *, #19289, .T. ) ;
#1155=CARTESIAN_POINT ( 'NONE',  ( 85.87499999726881583, 171.3844434931184253, -7.942151717890134290E-15 ) ) ;
#1160=CARTESIAN_POINT ( 'NONE',  ( 69.67499999726879878, 168.2552932293087906, -9.630534252274387086 ) ) ;
#1162=CARTESIAN_POINT ( 'NONE',  ( 41.28867513459482552, 170.7719333635740497, -7.904646289410545231E-15 ) ) ;
#1164=DIRECTION ( 'NONE',  ( 0.000000000000000000, 0.000000000000000000, -1.000000000000000000 ) ) ;
#1168=CARTESIAN_POINT ( 'NONE',  ( 88.17499999726881299, 164.1591823560292198, 12.60653300113718167 ) ) ;
#1171=CARTESIAN_POINT ( 'NONE',  ( 46.02499999726880731, 160.0630714827496206, 15.58253174999999402 ) ) ;
#1182=CARTESIAN_POINT ( 'NONE',  ( 68.99999999453763166, 155.0000000000000000, 14.49999999999999467 ) ) ;
#1189=ADVANCED_FACE ( 'NONE', ( #30983 ), #30977, .F. ) ;
#1191=ORIENTED_EDGE ( 'NONE', *, *, #15216, .F. ) ;
#1197=CARTESIAN_POINT ( 'NONE',  ( 127.5000000000000000, 78.52640161467446944, -73.43303922622258995 ) ) ;
#1199=CARTESIAN_POINT ( 'NONE',  ( 50.07499999726881157, 168.2552932293087906, 9.630534252274372875 ) ) ;
#1201=CARTESIAN_POINT ( 'NONE',  ( 54.52499999726881441, 140.1801316387863778, 4.815267126137185549 ) ) ;
#1210=CARTESIAN_POINT ( 'NONE',  ( 62.67499999726879878, 141.7447067706911810, 9.630534252274376428 ) ) ;
#1214=CARTESIAN_POINT ( 'NONE',  ( 81.30000000000001137, 163.5228861582408797, 11.73074641843673049 ) ) ;
#1215=CARTESIAN_POINT ( 'NONE',  ( 39.98867513459482126, 146.1832212156128890, 12.13525491562421976 ) ) ;
#1219=CARTESIAN_POINT ( 'NONE',  ( 47.57499999726881867, 164.1591823560292198, -12.60653300113719766 ) ) ;
#1222=CARTESIAN_POINT ( 'NONE',  ( 79.32499999726881867, 164.1591823560292198, -12.60653300113719766 ) ) ;
#1227=CARTESIAN_POINT ( 'NONE',  ( 48.59999999453763309, 168.7903194862797420, 4.480746418436729606 ) ) ;
#1229=DIRECTION ( 'NONE',  ( 0.000000000000000000, 0.000000000000000000, 1.000000000000000000 ) ) ;
#1231=ORIENTED_EDGE ( 'NONE', *, *, #33099, .T. ) ;
#1239=EDGE_CURVE ( 'NONE', #23379, #18472, #26181, .T. ) ;
#1241=CARTESIAN_POINT ( 'NONE',  ( 51.51132485994281041, 146.1832212156128890, -12.13525491562423042 ) ) ;
#1245=DIRECTION ( 'NONE',  ( 1.000000000000000000, 0.000000000000000000, 0.000000000000000000 ) ) ;
#1248=ORIENTED_EDGE ( 'NONE', *, *, #24308, .T. ) ;
#1249=CARTESIAN_POINT ( 'NONE',  ( 41.12499999726880873, 155.0000000000000000, -15.58253175000000823 ) ) ;
#1254=CARTESIAN_POINT ( 'NONE',  ( 41.77499999726881441, 169.8198683612136222, -4.815267126137197984 ) ) ;
#1259=CARTESIAN_POINT ( 'NONE',  ( 53.10000000000000142, 168.7903194862797420, 4.480746418436729606 ) ) ;
#1260=CARTESIAN_POINT ( 'NONE',  ( 63.38867513459482694, 169.2658477444273331, 4.635254915624208216 ) ) ;
#1266=CARTESIAN_POINT ( 'NONE',  ( 59.62499999726882294, 171.3844434931184253, -7.942151717890132712E-15 ) ) ;
#1269=CARTESIAN_POINT ( 'NONE',  ( 43.21132485994281325, 139.2280666364260071, -4.041636747397287284E-15 ) ) ;
#1270=CARTESIAN_POINT ( 'NONE',  ( 81.57499999726880446, 164.1591823560292198, -12.60653300113719766 ) ) ;
#1274=ORIENTED_EDGE ( 'NONE', *, *, #15983, .F. ) ;
#1276=CIRCLE ( 'NONE', #741, 2.149999999999985256 ) ;
#1293=CARTESIAN_POINT ( 'NONE',  ( 82.52499999726880731, 140.1801316387863778, 4.815267126137185549 ) ) ;
#1294=ORIENTED_EDGE ( 'NONE', *, *, #3214, .F. ) ;
#1295=CARTESIAN_POINT ( 'NONE',  ( 68.91132485994280898, 146.1832212156128890, 12.13525491562421976 ) ) ;
#1297=CARTESIAN_POINT ( 'NONE',  ( 79.42499999726881299, 168.2552932293087906, -9.630534252274385310 ) ) ;
#1303=CARTESIAN_POINT ( 'NONE',  ( 33.80000000000000426, 142.6655632788954620, 8.961492836873471646 ) ) ;
#1307=CARTESIAN_POINT ( 'NONE',  ( 73.61132485994279762, 150.1262045565062806, -14.99999999999993072 ) ) ;
#1309=DIRECTION ( 'NONE',  ( 0.000000000000000000, 0.000000000000000000, -1.000000000000000000 ) ) ;
#1310=CARTESIAN_POINT ( 'NONE',  ( 51.02499999726880731, 149.9369285172503510, -15.58253175000000823 ) ) ;
#1318=CARTESIAN_POINT ( 'NONE',  ( 83.29999999453764303, 142.6655632788954620, 8.961492836873471646 ) ) ;
#1323=ORIENTED_EDGE ( 'NONE', *, *, #11989, .F. ) ;
#1326=CARTESIAN_POINT ( 'NONE',  ( 72.47499999726878173, 149.9369285172503510, 15.58253174999999580 ) ) ;
#1328=VERTEX_POINT ( 'NONE', #26846 ) ;
#1329=CARTESIAN_POINT ( 'NONE',  ( 82.47499999726879594, 149.9369285172503510, 15.58253174999999580 ) ) ;
#1336=CARTESIAN_POINT ( 'NONE',  ( 71.27499999726882152, 149.9369285172503510, -15.58253175000000823 ) ) ;
#1339=CARTESIAN_POINT ( 'NONE',  ( 51.98867513459482126, 146.1832212156128890, 12.13525491562421976 ) ) ;
#1344=CARTESIAN_POINT ( 'NONE',  ( 37.91132485994280898, 163.8167787843871110, -12.13525491562423397 ) ) ;
#1346=CARTESIAN_POINT ( 'NONE',  ( 42.82499999726879736, 141.7447067706911810, -9.630534252274385310 ) ) ;
#1347=DIRECTION ( 'NONE',  ( 0.000000000000000000, 0.000000000000000000, -1.000000000000000000 ) ) ;
#1348=CARTESIAN_POINT ( 'NONE',  ( 34.02499999726880731, 160.0630714827496206, 15.58253174999999224 ) ) ;
#1356=CARTESIAN_POINT ( 'NONE',  ( 69.99999999453763166, 155.0000000000000000, -14.50000000000000711 ) ) ;
#1357=EDGE_LOOP ( 'NONE', ( #5317, #13106 ) ) ;
#1362=CARTESIAN_POINT ( 'NONE',  ( 45.51132485994280330, 146.1832212156128890, -12.13525491562423042 ) ) ;
#1370=CARTESIAN_POINT ( 'NONE',  ( 55.71132485994280614, 155.0000000000000000, -15.00000000000002487 ) ) ;
#1373=CARTESIAN_POINT ( 'NONE',  ( 50.87499999726881583, 138.6155565068815747, -3.929120461958505118E-15 ) ) ;
#1377=CYLINDRICAL_SURFACE ( 'NONE', #8631, 15.00000000000001776 ) ;
#1379=CARTESIAN_POINT ( 'NONE',  ( 56.77499999726881441, 140.1801316387863778, 4.815267126137185549 ) ) ;
#1385=CARTESIAN_POINT ( 'NONE',  ( 80.60000000000000853, 159.7113355953771077, -14.50000000000000888 ) ) ;
#1390=CARTESIAN_POINT ( 'NONE',  ( 43.37499999726881583, 155.0000000000000000, -15.58253175000000823 ) ) ;
#1392=CARTESIAN_POINT ( 'NONE',  ( 85.42499999726879878, 168.2552932293087906, -9.630534252274385310 ) ) ;
#1396=CARTESIAN_POINT ( 'NONE',  ( 48.09999999453763309, 159.7113355953771077, -14.50000000000000888 ) ) ;
#1397=( BOUNDED_CURVE ( )  B_SPLINE_CURVE ( 2, ( #526, #26411, #26243, #10593, #8684, #8199, #10918, #11242, #5782, #16178, #31365 ),
 .UNSPECIFIED., .F., .T. ) 
 B_SPLINE_CURVE_WITH_KNOTS ( ( 3, 2, 2, 2, 2, 3 ),
 ( 0.5714285714285713969, 0.5749999999999999556, 0.5785714285714284033, 0.5821428571428569620, 0.5857142857142854098, 0.5892857142857139685 ),
 .UNSPECIFIED. ) 
 CURVE ( )  GEOMETRIC_REPRESENTATION_ITEM ( )  RATIONAL_B_SPLINE_CURVE ( ( 1.000000000000000000, 0.9510565162951534202, 1.000000000000000000, 0.9510565162951534202, 1.000000000000000000, 0.9510565162951534202, 1.000000000000000000, 0.9510565162951534202, 1.000000000000000000, 0.9510565162951564178, 0.9999999999999970024 ) ) 
 REPRESENTATION_ITEM ( '' )  );
#1400=CARTESIAN_POINT ( 'NONE',  ( 117.5000000000000142, 155.0000000000000000, -6.938893903907228378E-15 ) ) ;
#1408=CARTESIAN_POINT ( 'NONE',  ( 50.78867513459482552, 155.0000000000000000, -15.00000000000002487 ) ) ;
#1416=CARTESIAN_POINT ( 'NONE',  ( 38.62499999726880873, 138.6155565068815463, -3.929120461958505118E-15 ) ) ;
#1420=CARTESIAN_POINT ( 'NONE',  ( 42.57499999726881157, 145.8408176439707802, 12.60653300113718345 ) ) ;
#1421=DIRECTION ( 'NONE',  ( 0.000000000000000000, 0.000000000000000000, -1.000000000000000000 ) ) ;
#1424=CARTESIAN_POINT ( 'NONE',  ( 64.00000000000000000, 139.7537977485451393, -4.138211985947621020E-15 ) ) ;
#1429=CARTESIAN_POINT ( 'NONE',  ( 66.22499999726879594, 149.9369285172503510, 15.58253174999999580 ) ) ;
#1433=CARTESIAN_POINT ( 'NONE',  ( 80.97499999726881015, 140.1801316387863778, -4.815267126137194431 ) ) ;
#1436=CARTESIAN_POINT ( 'NONE',  ( 71.98867513459481415, 146.1832212156128890, 12.13525491562421976 ) ) ;
#1437=CARTESIAN_POINT ( 'NONE',  ( 52.78867513459482552, 155.0000000000000000, -15.00000000000002487 ) ) ;
#1445=EDGE_CURVE ( 'NONE', #562, #19762, #2143, .T. ) ;
#1449=CARTESIAN_POINT ( 'NONE',  ( 63.61132485994281893, 150.1262045565062806, -14.99999999999993072 ) ) ;
#1454=CARTESIAN_POINT ( 'NONE',  ( 85.32499999726880446, 164.1591823560292198, -12.60653300113719766 ) ) ;
#1457=CARTESIAN_POINT ( 'NONE',  ( 79.32499999726881867, 164.1591823560292198, -12.60653300113719766 ) ) ;
#1462=CARTESIAN_POINT ( 'NONE',  ( 42.10000000000000142, 141.2096805137202580, -4.480746418436742040 ) ) ;
#1464=EDGE_CURVE ( 'NONE', #7737, #13563, #32457, .T. ) ;
#1465=EDGE_CURVE ( 'NONE', #1492, #15895, #8561, .T. ) ;
#1468=CARTESIAN_POINT ( 'NONE',  ( 78.68867513459480278, 150.1262045565062522, -14.99999999999990763 ) ) ;
#1469=LINE ( 'NONE', #27359, #5012 ) ;
#1470=CARTESIAN_POINT ( 'NONE',  ( 53.62499999726881583, 171.3844434931184253, -7.942151717890134290E-15 ) ) ;
#1471=CARTESIAN_POINT ( 'NONE',  ( 65.27499999726880731, 149.9369285172503510, -15.58253175000000823 ) ) ;
#1480=CARTESIAN_POINT ( 'NONE',  ( 83.59999999453762598, 141.2096805137202580, -4.480746418436742040 ) ) ;
#1490=CARTESIAN_POINT ( 'NONE',  ( 68.57499999726881867, 145.8408176439707802, 12.60653300113718345 ) ) ;
#1492=VERTEX_POINT ( 'NONE', #16788 ) ;
#1494=CARTESIAN_POINT ( 'NONE',  ( 84.87499999726881583, 138.6155565068815747, -3.929120461958505118E-15 ) ) ;
#1502=DIRECTION ( 'NONE',  ( 1.000000000000000000, 0.000000000000000000, 0.000000000000000000 ) ) ;
#1507=CARTESIAN_POINT ( 'NONE',  ( 71.41132485994282320, 142.2402378747194405, -9.270509831248439525 ) ) ;
#1512=CARTESIAN_POINT ( 'NONE',  ( 44.42499999726881299, 141.7447067706911810, 9.630534252274376428 ) ) ;
#1513=CARTESIAN_POINT ( 'NONE',  ( 87.50000000000001421, 155.6617420473934885, -15.38934888333735884 ) ) ;
#1523=CARTESIAN_POINT ( 'NONE',  ( 69.19999999453763451, 146.4771138417591203, 11.73074641843673227 ) ) ;
#1524=ORIENTED_EDGE ( 'NONE', *, *, #31571, .T. ) ;
#1534=CARTESIAN_POINT ( 'NONE',  ( 42.48867513459482836, 142.2402378747194405, -9.270509831248439525 ) ) ;
#1538=CARTESIAN_POINT ( 'NONE',  ( 55.31132485994280756, 140.7341522555726669, -4.635254915624220651 ) ) ;
#1540=CARTESIAN_POINT ( 'NONE',  ( 50.47499999726881015, 149.9369285172503510, 15.58253174999999580 ) ) ;
#1541=AXIS2_PLACEMENT_3D ( 'NONE', #27704, #4366, #11701 ) ;
#1545=DIRECTION ( 'NONE',  ( 0.000000000000000000, 0.000000000000000000, -1.000000000000000000 ) ) ;
#1547=CARTESIAN_POINT ( 'NONE',  ( 58.57499999726881157, 145.8408176439707802, 12.60653300113718345 ) ) ;
#1552=CARTESIAN_POINT ( 'NONE',  ( 78.10000000000000853, 141.2096805137202580, -4.480746418436742040 ) ) ;
#1558=CARTESIAN_POINT ( 'NONE',  ( 41.87499999726880162, 171.3844434931184253, -7.942151717890132712E-15 ) ) ;
#1561=CARTESIAN_POINT ( 'NONE',  ( 84.22499999726879594, 149.9369285172503510, 15.58253174999999580 ) ) ;
#1565=CARTESIAN_POINT ( 'NONE',  ( 46.39999999453763024, 168.7903194862797420, -4.480746418436745593 ) ) ;
#1570=CARTESIAN_POINT ( 'NONE',  ( 66.71132485994280614, 155.0000000000000000, 15.00000000000001243 ) ) ;
#1571=ORIENTED_EDGE ( 'NONE', *, *, #15447, .F. ) ;
#1577=EDGE_LOOP ( 'NONE', ( #29940, #16353, #31307, #23424 ) ) ;
#1580=DIRECTION ( 'NONE',  ( 0.000000000000000000, 0.000000000000000000, -1.000000000000000000 ) ) ;
#1584=CARTESIAN_POINT ( 'NONE',  ( 35.62499999726880873, 171.3844434931184253, -7.942151717890132712E-15 ) ) ;
#1589=CARTESIAN_POINT ( 'NONE',  ( 40.07499999726879736, 168.2552932293087906, 9.630534252274372875 ) ) ;
#1593=CARTESIAN_POINT ( 'NONE',  ( 60.90000000000000568, 168.7903194862797420, -4.480746418436745593 ) ) ;
#1594=( BOUNDED_CURVE ( )  B_SPLINE_CURVE ( 2, ( #20468, #30870, #7534, #2414, #12799, #23191, #10264, #20642, #31039, #352, #13622 ),
 .UNSPECIFIED., .F., .T. ) 
 B_SPLINE_CURVE_WITH_KNOTS ( ( 3, 2, 2, 2, 2, 3 ),
 ( 0.7857142857142856984, 0.7892857142857142572, 0.7928571428571428159, 0.7964285714285713746, 0.8000000000000000444, 0.8035714285714286031 ),
 .UNSPECIFIED. ) 
 CURVE ( )  GEOMETRIC_REPRESENTATION_ITEM ( )  RATIONAL_B_SPLINE_CURVE ( ( 1.000000000000000000, 0.9510565162951534202, 1.000000000000000000, 0.9510565162951534202, 1.000000000000000000, 0.9510565162951534202, 1.000000000000000000, 0.9510565162951534202, 1.000000000000000000, 0.9510565162951534202, 1.000000000000000000 ) ) 
 REPRESENTATION_ITEM ( '' )  );
#1599=CARTESIAN_POINT ( 'NONE',  ( 62.02499999726880020, 160.0630714827496206, 15.58253174999999402 ) ) ;
#1603=CARTESIAN_POINT ( 'NONE',  ( 79.77499999726880731, 169.8198683612136222, -4.815267126137197984 ) ) ;
#1606=LINE ( 'NONE', #11667, #20843 ) ;
#1615=EDGE_CURVE ( 'NONE', #31412, #31779, #972, .T. ) ;
#1620=ORIENTED_EDGE ( 'NONE', *, *, #3918, .T. ) ;
#1621=CARTESIAN_POINT ( 'NONE',  ( 82.92499999726882720, 145.8408176439707802, -12.60653300113719588 ) ) ;
#1623=CARTESIAN_POINT ( 'NONE',  ( 69.78867513459482552, 155.0000000000000000, 15.00000000000001243 ) ) ;
#1624=CARTESIAN_POINT ( 'NONE',  ( 77.42499999726882720, 168.2552932293087906, -9.630534252274385310 ) ) ;
#1625=EDGE_CURVE ( 'NONE', #16276, #8938, #29825, .T. ) ;
#1628=CARTESIAN_POINT ( 'NONE',  ( 74.98867513459481415, 163.8167787843871110, -12.13525491562423397 ) ) ;
#1629=CARTESIAN_POINT ( 'NONE',  ( 41.59999999999999432, 150.2886644046228639, 14.49999999999999645 ) ) ;
#1633=CARTESIAN_POINT ( 'NONE',  ( 78.78867513459481131, 155.0000000000000000, -15.00000000000002487 ) ) ;
#1635=CARTESIAN_POINT ( 'NONE',  ( 53.22499999726879594, 160.0630714827496206, -15.58253175000000823 ) ) ;
#1636=CARTESIAN_POINT ( 'NONE',  ( 63.47499999726881725, 160.0630714827496206, -15.58253175000000823 ) ) ;
#1651=CARTESIAN_POINT ( 'NONE',  ( 71.77499999726882152, 169.8198683612136222, -4.815267126137197984 ) ) ;
#1655=EDGE_CURVE ( 'NONE', #30153, #24793, #17888, .T. ) ;
#1656=CARTESIAN_POINT ( 'NONE',  ( 86.07499999726880446, 168.2552932293087906, 9.630534252274372875 ) ) ;
#1657=CARTESIAN_POINT ( 'NONE',  ( 32.50000000000000000, 155.0000000000000000, -6.938893903907228378E-15 ) ) ;
#1676=CARTESIAN_POINT ( 'NONE',  ( 43.72499999726881015, 169.8198683612136222, 4.815267126137181997 ) ) ;
#1677=CYLINDRICAL_SURFACE ( 'NONE', #23078, 15.00000000000001776 ) ;
#1683=CARTESIAN_POINT ( 'NONE',  ( 75.88867513459484826, 150.1262045565061385, 14.99999999999982947 ) ) ;
#1687=CARTESIAN_POINT ( 'NONE',  ( 68.19999999453763451, 163.5228861582408797, -11.73074641843674470 ) ) ;
#1698=CARTESIAN_POINT ( 'NONE',  ( 87.49999999999995737, 167.3752416915453125, -9.523985490255702402 ) ) ;
#1702=CARTESIAN_POINT ( 'NONE',  ( 127.5000000000000000, 155.0000000000000000, -6.938893903907228378E-15 ) ) ;
#1704=CARTESIAN_POINT ( 'NONE',  ( 58.27499999726880731, 160.0630714827496206, 15.58253174999999224 ) ) ;
#1710=CARTESIAN_POINT ( 'NONE',  ( 67.57499999726881867, 164.1591823560292198, -12.60653300113719766 ) ) ;
#1715=CARTESIAN_POINT ( 'NONE',  ( 82.00000000000001421, 139.7537977485451393, -4.138211985947621020E-15 ) ) ;
#1720=CARTESIAN_POINT ( 'NONE',  ( 44.97499999726881015, 140.1801316387863778, -4.815267126137194431 ) ) ;
#1722=CARTESIAN_POINT ( 'NONE',  ( 83.02499999726879309, 149.9369285172503510, -15.58253175000000823 ) ) ;
#1723=DIRECTION ( 'NONE',  ( -1.000000000000000000, -0.000000000000000000, -0.000000000000000000 ) ) ;
#1725=CARTESIAN_POINT ( 'NONE',  ( 45.09999999453763309, 150.2886644046228639, 14.49999999999999645 ) ) ;
#1730=CARTESIAN_POINT ( 'NONE',  ( 73.71132485994280614, 155.0000000000000000, -15.00000000000002487 ) ) ;
#1743=CARTESIAN_POINT ( 'NONE',  ( 37.47499999726880304, 160.0630714827496206, -15.58253175000000823 ) ) ;
#1744=ORIENTED_EDGE ( 'NONE', *, *, #31666, .F. ) ;
#1745=CARTESIAN_POINT ( 'NONE',  ( 45.02499999726880731, 149.9369285172503510, -15.58253175000000823 ) ) ;
#1746=CARTESIAN_POINT ( 'NONE',  ( 38.88867513459482694, 159.8737954434936057, -15.00000000000002665 ) ) ;
#1749=CARTESIAN_POINT ( 'NONE',  ( 42.77499999726880731, 140.1801316387863778, 4.815267126137185549 ) ) ;
#1755=CARTESIAN_POINT ( 'NONE',  ( 62.39999999999999858, 150.2886644046228639, -14.50000000000000888 ) ) ;
#1762=CARTESIAN_POINT ( 'NONE',  ( 61.92499999726882010, 164.1591823560292198, 12.60653300113718167 ) ) ;
#1765=CARTESIAN_POINT ( 'NONE',  ( 42.71132485994280614, 155.0000000000000000, 15.00000000000001243 ) ) ;
#1767=CARTESIAN_POINT ( 'NONE',  ( 80.27499999726879309, 160.0630714827496206, 15.58253174999999402 ) ) ;
#1784=CARTESIAN_POINT ( 'NONE',  ( 81.32499999726880446, 164.1591823560292198, -12.60653300113719766 ) ) ;
#1789=CARTESIAN_POINT ( 'NONE',  ( 75.92499999726881299, 164.1591823560292198, 12.60653300113718167 ) ) ;
#1790=CARTESIAN_POINT ( 'NONE',  ( 53.78867513459483263, 155.0000000000000000, 15.00000000000001243 ) ) ;
#1795=CARTESIAN_POINT ( 'NONE',  ( 43.80000000000001137, 142.6655632788954620, 8.961492836873471646 ) ) ;
#1803=CARTESIAN_POINT ( 'NONE',  ( 49.32499999726881157, 164.1591823560292198, -12.60653300113719766 ) ) ;
#1804=CARTESIAN_POINT ( 'NONE',  ( 62.87499999726881583, 138.6155565068815463, -3.929120461958505118E-15 ) ) ;
#1806=CARTESIAN_POINT ( 'NONE',  ( 40.71132485994280614, 155.0000000000000000, 15.00000000000001243 ) ) ;
#1813=AXIS2_PLACEMENT_3D ( 'NONE', #4996, #18112, #8223 ) ;
#1815=CARTESIAN_POINT ( 'NONE',  ( 83.51132485994280330, 146.1832212156128890, -12.13525491562423042 ) ) ;
#1824=CARTESIAN_POINT ( 'NONE',  ( 80.87499999726881583, 138.6155565068815463, -3.929120461958505118E-15 ) ) ;
#1827=ORIENTED_EDGE ( 'NONE', *, *, #20796, .F. ) ;
#1828=CARTESIAN_POINT ( 'NONE',  ( 84.67499999726881299, 141.7447067706911810, 9.630534252274376428 ) ) ;
#1833=CARTESIAN_POINT ( 'NONE',  ( 55.12499999726881583, 155.0000000000000000, -15.58253175000000823 ) ) ;
#1834=CARTESIAN_POINT ( 'NONE',  ( 87.50000000000001421, 155.0000000000000000, -6.938893903907228378E-15 ) ) ;
#1835=ADVANCED_FACE ( 'NONE', ( #28027 ), #9738, .T. ) ;
#1837=ORIENTED_EDGE ( 'NONE', *, *, #29441, .F. ) ;
#1838=DIRECTION ( 'NONE',  ( 1.000000000000000000, 0.000000000000000000, 0.000000000000000000 ) ) ;
#1848=CARTESIAN_POINT ( 'NONE',  ( 45.52499999726881441, 169.8198683612136222, -4.815267126137197984 ) ) ;
#1858=CARTESIAN_POINT ( 'NONE',  ( 85.18867513459483121, 169.2658477444273331, -4.635254915624224203 ) ) ;
#1861=CARTESIAN_POINT ( 'NONE',  ( 72.49999999453761745, 170.2462022514548323, -7.872454543227099337E-15 ) ) ;
#1868=ORIENTED_EDGE ( 'NONE', *, *, #27409, .F. ) ;
#1870=ORIENTED_EDGE ( 'NONE', *, *, #28229, .F. ) ;
#1872=ADVANCED_FACE ( 'NONE', ( #26935 ), #1377, .T. ) ;
#1874=CYLINDRICAL_SURFACE ( 'NONE', #16753, 15.00000000000001776 ) ;
#1881=CARTESIAN_POINT ( 'NONE',  ( 53.57499999726881157, 164.1591823560292198, -12.60653300113719766 ) ) ;
#1884=LINE ( 'NONE', #12269, #30881 ) ;
#1888=CARTESIAN_POINT ( 'NONE',  ( 66.47499999726882436, 149.9369285172503510, 15.58253174999999580 ) ) ;
#1890=DIRECTION ( 'NONE',  ( 0.000000000000000000, -0.7071067811865442421, 0.7071067811865506814 ) ) ;
#1893=CARTESIAN_POINT ( 'NONE',  ( 80.90000000000000568, 168.7903194862797420, -4.480746418436745593 ) ) ;
#1898=CARTESIAN_POINT ( 'NONE',  ( 48.97499999726881725, 140.1801316387863778, -4.815267126137194431 ) ) ;
#1902=CARTESIAN_POINT ( 'NONE',  ( 81.02499999726880731, 149.9369285172503510, -15.58253175000000823 ) ) ;
#1905=CARTESIAN_POINT ( 'NONE',  ( 51.69999999453762030, 142.6655632788954620, -8.961492836873480528 ) ) ;
#1923=CARTESIAN_POINT ( 'NONE',  ( 36.37499999726881583, 155.0000000000000000, 15.58253174999999402 ) ) ;
#1925=CARTESIAN_POINT ( 'NONE',  ( 44.82499999726880446, 141.7447067706911810, -9.630534252274385310 ) ) ;
#1929=CARTESIAN_POINT ( 'NONE',  ( 46.07499999726881157, 168.2552932293087906, 9.630534252274372875 ) ) ;
#1933=CARTESIAN_POINT ( 'NONE',  ( 58.00000000000000711, 139.7537977485451393, -4.138211985947621020E-15 ) ) ;
#1935=CARTESIAN_POINT ( 'NONE',  ( 64.51132485994280330, 163.8167787843871110, 12.13525491562421621 ) ) ;
#1940=CARTESIAN_POINT ( 'NONE',  ( 64.52499999726882152, 140.1801316387863778, 4.815267126137185549 ) ) ;
#1942=ORIENTED_EDGE ( 'NONE', *, *, #405, .T. ) ;
#1944=CARTESIAN_POINT ( 'NONE',  ( 85.27499999726879309, 149.9369285172503510, -15.58253175000000823 ) ) ;
#1947=( BOUNDED_CURVE ( )  B_SPLINE_CURVE ( 2, ( #1623, #11852, #32626, #14569, #8783, #11349, #4013, #12013, #21730, #19682, #1123 ),
 .UNSPECIFIED., .F., .T. ) 
 B_SPLINE_CURVE_WITH_KNOTS ( ( 3, 2, 2, 2, 2, 3 ),
 ( 0.3214285714285712303, 0.3249999999999997891, 0.3285714285714283478, 0.3321428571428569620, 0.3357142857142855208, 0.3392857142857140795 ),
 .UNSPECIFIED. ) 
 CURVE ( )  GEOMETRIC_REPRESENTATION_ITEM ( )  RATIONAL_B_SPLINE_CURVE ( ( 1.000000000000002220, 0.9510565162951510887, 1.000000000000000000, 0.9510565162951534202, 1.000000000000000000, 0.9510565162951534202, 1.000000000000000000, 0.9510565162951534202, 1.000000000000000000, 0.9510565162951549745, 0.9999999999999984457 ) ) 
 REPRESENTATION_ITEM ( '' )  );
#1959=CARTESIAN_POINT ( 'NONE',  ( 69.81132485994281467, 159.8737954434934920, -15.00000000000012434 ) ) ;
#1965=CARTESIAN_POINT ( 'NONE',  ( 73.27499999726882152, 149.9369285172503510, -15.58253175000000823 ) ) ;
#1966=CARTESIAN_POINT ( 'NONE',  ( 81.22499999726882436, 160.0630714827496206, -15.58253175000000823 ) ) ;
#1971=CARTESIAN_POINT ( 'NONE',  ( 41.20000000000000284, 167.3344367211045096, 8.961492836873468093 ) ) ;
#1977=CARTESIAN_POINT ( 'NONE',  ( 58.92499999726881299, 145.8408176439707802, -12.60653300113719588 ) ) ;
#1978=CARTESIAN_POINT ( 'NONE',  ( 64.67499999726878457, 141.7447067706911810, 9.630534252274376428 ) ) ;
#1981=PLANE ( 'NONE',  #9716 ) ;
#1989=CARTESIAN_POINT ( 'NONE',  ( 82.91132485994279477, 146.1832212156128890, 12.13525491562421976 ) ) ;
#1997=CARTESIAN_POINT ( 'NONE',  ( 76.77499999726880731, 140.1801316387863778, 4.815267126137185549 ) ) ;
#2002=CARTESIAN_POINT ( 'NONE',  ( 71.52499999726882152, 169.8198683612136222, -4.815267126137197984 ) ) ;
#2004=COLOUR_RGB ( '', 0.31764706, 0.68627451, 0.89019608) ;
#2005=LINE ( 'NONE', #27383, #32872 ) ;
#2006=CARTESIAN_POINT ( 'NONE',  ( 56.42499999726881299, 141.7447067706911810, 9.630534252274376428 ) ) ;
#2009=VERTEX_POINT ( 'NONE', #3424 ) ;
#2016=FACE_OUTER_BOUND ( 'NONE', #11926, .T. ) ;
#2032=CARTESIAN_POINT ( 'NONE',  ( 85.28867513459485394, 170.7719333635740497, -7.904646289410545231E-15 ) ) ;
#2035=CARTESIAN_POINT ( 'NONE',  ( 76.29999999453761461, 167.3344367211045096, -8.961492836873482304 ) ) ;
#2036=ORIENTED_EDGE ( 'NONE', *, *, #29715, .T. ) ;
#2042=AXIS2_PLACEMENT_3D ( 'NONE', #21703, #6196, #16414 ) ;
#2043=ORIENTED_EDGE ( 'NONE', *, *, #15447, .T. ) ;
#2044=ORIENTED_EDGE ( 'NONE', *, *, #6265, .F. ) ;
#2046=CARTESIAN_POINT ( 'NONE',  ( 51.78867513459482552, 155.0000000000000000, 15.00000000000001243 ) ) ;
#2051=CARTESIAN_POINT ( 'NONE',  ( 55.01132485994281041, 142.2402378747194405, 9.270509831248432420 ) ) ;
#2053=CARTESIAN_POINT ( 'NONE',  ( 53.47499999726881015, 160.0630714827496206, -15.58253175000000823 ) ) ;
#2057=VECTOR ( 'NONE', #8457, 1000.000000000000000 ) ;
#2060=CARTESIAN_POINT ( 'NONE',  ( 68.47499999726878173, 149.9369285172503510, 15.58253174999999580 ) ) ;
#2066=CARTESIAN_POINT ( 'NONE',  ( 86.10000000000000853, 141.2096805137202580, -4.480746418436742040 ) ) ;
#2070=CARTESIAN_POINT ( 'NONE',  ( 53.07499999726880446, 141.7447067706911810, -9.630534252274385310 ) ) ;
#2073=CARTESIAN_POINT ( 'NONE',  ( 82.32499999726880446, 145.8408176439707802, 12.60653300113718345 ) ) ;
#2076=CARTESIAN_POINT ( 'NONE',  ( 54.79999999453763593, 163.5228861582408797, 11.73074641843673049 ) ) ;
#2098=CARTESIAN_POINT ( 'NONE',  ( 39.77499999726881441, 169.8198683612136222, -4.815267126137197984 ) ) ;
#2099=ORIENTED_EDGE ( 'NONE', *, *, #22368, .F. ) ;
#2100=CARTESIAN_POINT ( 'NONE',  ( 42.12499999726881583, 155.0000000000000000, 15.58253174999999402 ) ) ;
#2105=CARTESIAN_POINT ( 'NONE',  ( 44.87499999726880873, 138.6155565068815463, -3.929120461958505118E-15 ) ) ;
#2111=CARTESIAN_POINT ( 'NONE',  ( 61.79999999999999716, 142.6655632788954620, 8.961492836873471646 ) ) ;
#2120=CARTESIAN_POINT ( 'NONE',  ( 61.32499999726881157, 164.1591823560292198, -12.60653300113719766 ) ) ;
#2124=CARTESIAN_POINT ( 'NONE',  ( 34.99999999453763166, 155.0000000000000000, 14.49999999999999467 ) ) ;
#2133=CARTESIAN_POINT ( 'NONE',  ( 66.28867513459483973, 139.2280666364260071, -4.041636747397287284E-15 ) ) ;
#2135=FACE_OUTER_BOUND ( 'NONE', #29476, .T. ) ;
#2136=EDGE_LOOP ( 'NONE', ( #33216, #22533, #24327, #939 ) ) ;
#2137=CARTESIAN_POINT ( 'NONE',  ( 70.11132485994281183, 169.2658477444273331, -4.635254915624224203 ) ) ;
#2140=DIRECTION ( 'NONE',  ( 0.000000000000000000, 0.000000000000000000, -1.000000000000000000 ) ) ;
#2143=B_SPLINE_CURVE_WITH_KNOTS ( 'NONE', 3,
 ( #16956, #32297, #27351, #14236, #12193, #4017, #22073, #14739, #14411, #27520, #17134, #12018, #30080, #27852, #9629, #20026 ),
 .UNSPECIFIED., .F., .F.,
 ( 4, 2, 2, 2, 2, 2, 2, 4 ),
 ( 0.01344638572600751272, 0.01751370969988639420, 0.01954737168682584708, 0.02158103367376530690, 0.02361469566070476672, 0.02564835764764422307, 0.02768201963458367942, 0.02971568162152313924 ),
 .UNSPECIFIED. ) ;
#2144=CARTESIAN_POINT ( 'NONE',  ( 79.92499999726881299, 164.1591823560292198, 12.60653300113718167 ) ) ;
#2149=CARTESIAN_POINT ( 'NONE',  ( 41.39999999999999147, 159.7113355953771077, 14.49999999999999289 ) ) ;
#2155=CARTESIAN_POINT ( 'NONE',  ( 58.22499999726881015, 149.9369285172503510, 15.58253174999999580 ) ) ;
#2156=CARTESIAN_POINT ( 'NONE',  ( 67.87499999726881583, 171.3844434931184253, -7.942151717890132712E-15 ) ) ;
#2158=DIRECTION ( 'NONE',  ( 1.000000000000000000, 0.000000000000000000, 0.000000000000000000 ) ) ;
#2165=CARTESIAN_POINT ( 'NONE',  ( 74.18867513459481700, 140.7341522555726669, 4.635254915624211769 ) ) ;
#2169=ORIENTED_EDGE ( 'NONE', *, *, #27707, .F. ) ;
#2171=ORIENTED_EDGE ( 'NONE', *, *, #10125, .T. ) ;
#2172=CARTESIAN_POINT ( 'NONE',  ( 79.97499999726881015, 169.8198683612136222, 4.815267126137181997 ) ) ;
#2176=CARTESIAN_POINT ( 'NONE',  ( 70.62499999726881583, 138.6155565068815747, -3.929120461958505118E-15 ) ) ;
#2179=CARTESIAN_POINT ( 'NONE',  ( 65.72499999726881015, 169.8198683612136222, 4.815267126137181997 ) ) ;
#2184=DIRECTION ( 'NONE',  ( 1.000000000000000000, 0.000000000000000000, 0.000000000000000000 ) ) ;
#2196=CARTESIAN_POINT ( 'NONE',  ( 37.42499999726881299, 168.2552932293087906, -9.630534252274387086 ) ) ;
#2204=CARTESIAN_POINT ( 'NONE',  ( 73.09999999453764019, 150.2886644046228639, 14.49999999999999645 ) ) ;
#2205=ORIENTED_EDGE ( 'NONE', *, *, #7919, .F. ) ;
#2218=CARTESIAN_POINT ( 'NONE',  ( 81.71132485994280614, 155.0000000000000000, -15.00000000000002487 ) ) ;
#2220=CARTESIAN_POINT ( 'NONE',  ( 56.27499999726880731, 160.0630714827496206, 15.58253174999999224 ) ) ;
#2224=SURFACE_STYLE_FILL_AREA ( #17551 ) ;
#2227=CARTESIAN_POINT ( 'NONE',  ( 66.67499999726881299, 141.7447067706911810, 9.630534252274376428 ) ) ;
#2233=CARTESIAN_POINT ( 'NONE',  ( 34.02499999726880731, 160.0630714827496206, 15.58253174999999402 ) ) ;
#2237=EDGE_CURVE ( 'NONE', #28404, #29398, #25221, .T. ) ;
#2239=CARTESIAN_POINT ( 'NONE',  ( 53.27499999726880731, 149.9369285172503510, -15.58253175000000823 ) ) ;
#2241=DIRECTION ( 'NONE',  ( 1.000000000000000000, 0.000000000000000000, 0.000000000000000000 ) ) ;
#2242=EDGE_CURVE ( 'NONE', #25792, #19681, #24675, .T. ) ;
#2245=CARTESIAN_POINT ( 'NONE',  ( 52.09999999453762598, 159.7113355953771077, -14.50000000000000888 ) ) ;
#2259=ORIENTED_EDGE ( 'NONE', *, *, #16821, .F. ) ;
#2263=CARTESIAN_POINT ( 'NONE',  ( 38.17499999726881299, 164.1591823560292198, 12.60653300113718167 ) ) ;
#2265=CARTESIAN_POINT ( 'NONE',  ( 44.12499999726881583, 155.0000000000000000, 15.58253174999999402 ) ) ;
#2269=CARTESIAN_POINT ( 'NONE',  ( 47.47499999726881015, 160.0630714827496206, -15.58253175000000823 ) ) ;
#2273=CARTESIAN_POINT ( 'NONE',  ( 68.00000000000001421, 139.7537977485451393, -4.138211985947621020E-15 ) ) ;
#2278=CARTESIAN_POINT ( 'NONE',  ( 33.37499999726880873, 155.0000000000000000, -15.58253175000000823 ) ) ;
#2280=CARTESIAN_POINT ( 'NONE',  ( 72.52499999726882152, 140.1801316387863778, 4.815267126137185549 ) ) ;
#2282=ORIENTED_EDGE ( 'NONE', *, *, #24533, .F. ) ;
#2285=CARTESIAN_POINT ( 'NONE',  ( 35.29999999453763593, 142.6655632788954620, 8.961492836873471646 ) ) ;
#2298=DIRECTION ( 'NONE',  ( 0.000000000000000000, 0.000000000000000000, -1.000000000000000000 ) ) ;
#2300=CARTESIAN_POINT ( 'NONE',  ( 69.91132485994280898, 163.8167787843871110, -12.13525491562423397 ) ) ;
#2303=ORIENTED_EDGE ( 'NONE', *, *, #1655, .T. ) ;
#2305=ORIENTED_EDGE ( 'NONE', *, *, #7539, .F. ) ;
#2306=CARTESIAN_POINT ( 'NONE',  ( 81.41132485994280898, 142.2402378747194405, -9.270509831248439525 ) ) ;
#2308=CARTESIAN_POINT ( 'NONE',  ( 81.52499999726880731, 169.8198683612136222, -4.815267126137197984 ) ) ;
#2309=PLANE ( 'NONE',  #25202 ) ;
#2314=CARTESIAN_POINT ( 'NONE',  ( 48.79999999999999716, 167.3344367211045096, -8.961492836873482304 ) ) ;
#2316=CARTESIAN_POINT ( 'NONE',  ( 38.71132485994280614, 155.0000000000000000, 15.00000000000001243 ) ) ;
#2320=CARTESIAN_POINT ( 'NONE',  ( 58.02499999726880731, 160.0630714827496206, 15.58253174999999224 ) ) ;
#2321=CARTESIAN_POINT ( 'NONE',  ( 69.87499999726880162, 171.3844434931184253, -7.942151717890132712E-15 ) ) ;
#2323=FACE_BOUND ( 'NONE', #12251, .T. ) ;
#2342=CARTESIAN_POINT ( 'NONE',  ( 78.27499999726880731, 160.0630714827496206, 15.58253174999999402 ) ) ;
#2345=CARTESIAN_POINT ( 'NONE',  ( 71.72499999726881015, 169.8198683612136222, 4.815267126137181997 ) ) ;
#2348=CARTESIAN_POINT ( 'NONE',  ( 66.52499999726880731, 140.1801316387863778, 4.815267126137185549 ) ) ;
#2354=DIRECTION ( 'NONE',  ( -1.000000000000000000, 0.000000000000000000, -0.000000000000000000 ) ) ;
#2362=CARTESIAN_POINT ( 'NONE',  ( 46.78867513459482552, 155.0000000000000000, -15.00000000000002487 ) ) ;
#2363=CIRCLE ( 'NONE', #24112, 2.149999999999985256 ) ;
#2365=CARTESIAN_POINT ( 'NONE',  ( 41.02499999726880731, 149.9369285172503510, -15.58253175000000823 ) ) ;
#2375=CARTESIAN_POINT ( 'NONE',  ( 75.09999999453762598, 150.2886644046228639, 14.49999999999999645 ) ) ;
#2386=CARTESIAN_POINT ( 'NONE',  ( 32.50000000000000000, 155.0000000000000000, -6.938893903907228378E-15 ) ) ;
#2388=ORIENTED_EDGE ( 'NONE', *, *, #18646, .F. ) ;
#2394=AXIS2_PLACEMENT_3D ( 'NONE', #2422, #10096, #23196 ) ;
#2395=CARTESIAN_POINT ( 'NONE',  ( 57.67499999726880588, 168.2552932293087906, -9.630534252274387086 ) ) ;
#2398=SURFACE_SIDE_STYLE ('',( #2224 ) ) ;
#2403=DIRECTION ( 'NONE',  ( 1.000000000000000000, 0.000000000000000000, 0.000000000000000000 ) ) ;
#2404=AXIS2_PLACEMENT_3D ( 'NONE', #8872, #11941, #4266 ) ;
#2406=CARTESIAN_POINT ( 'NONE',  ( 33.62499999726881583, 171.3844434931184253, -7.942151717890132712E-15 ) ) ;
#2411=CARTESIAN_POINT ( 'NONE',  ( 49.17499999726881299, 145.8408176439707802, -12.60653300113719588 ) ) ;
#2413=CARTESIAN_POINT ( 'NONE',  ( 86.62499999726883004, 138.6155565068815463, -3.929120461958505118E-15 ) ) ;
#2414=CARTESIAN_POINT ( 'NONE',  ( 78.01132485994284593, 167.7597621252805880, -9.270509831248443078 ) ) ;
#2417=CARTESIAN_POINT ( 'NONE',  ( 52.79999999453763593, 163.5228861582408797, 11.73074641843673049 ) ) ;
#2422=CARTESIAN_POINT ( 'NONE',  ( 127.5000000000000000, 155.0000000000000000, -6.938893903907228378E-15 ) ) ;
#2424=CARTESIAN_POINT ( 'NONE',  ( 32.50000000000000000, 155.0000000000000000, 15.00000000000001243 ) ) ;
#2432=DIRECTION ( 'NONE',  ( 1.000000000000000000, 0.000000000000000000, 0.000000000000000000 ) ) ;
#2433=CARTESIAN_POINT ( 'NONE',  ( 79.57499999726881867, 164.1591823560292198, -12.60653300113719766 ) ) ;
#2437=CARTESIAN_POINT ( 'NONE',  ( 34.67499999726880588, 141.7447067706911810, 9.630534252274376428 ) ) ;
#2438=ORIENTED_EDGE ( 'NONE', *, *, #17837, .T. ) ;
#2439=CARTESIAN_POINT ( 'NONE',  ( 41.62499999726880162, 171.3844434931184253, -7.942151717890132712E-15 ) ) ;
#2440=CARTESIAN_POINT ( 'NONE',  ( 66.78867513459482552, 155.0000000000000000, -15.00000000000002487 ) ) ;
#2441=EDGE_CURVE ( 'NONE', #28404, #5476, #4849, .T. ) ;
#2445=CARTESIAN_POINT ( 'NONE',  ( 47.37499999726880873, 155.0000000000000000, -15.58253175000000823 ) ) ;
#2446=CARTESIAN_POINT ( 'NONE',  ( 89.50000000000001421, 155.0000000000000000, -6.938893903907228378E-15 ) ) ;
#2449=CARTESIAN_POINT ( 'NONE',  ( 70.40000000000000568, 150.2886644046228639, -14.50000000000000888 ) ) ;
#2456=CARTESIAN_POINT ( 'NONE',  ( 67.52499999726880731, 169.8198683612136222, -4.815267126137197984 ) ) ;
#2459=CARTESIAN_POINT ( 'NONE',  ( 37.39999999453763024, 141.2096805137202580, 4.480746418436733158 ) ) ;
#2475=CARTESIAN_POINT ( 'NONE',  ( 34.41132485994280898, 167.7597621252805880, 9.270509831248428867 ) ) ;
#2480=CARTESIAN_POINT ( 'NONE',  ( 85.82499999726879025, 168.2552932293087906, 9.630534252274372875 ) ) ;
#2485=CARTESIAN_POINT ( 'NONE',  ( 47.70000000000000284, 146.4771138417591203, 11.73074641843673227 ) ) ;
#2488=ADVANCED_FACE ( 'NONE', ( #2892 ), #10731, .T. ) ;
#2489=CARTESIAN_POINT ( 'NONE',  ( 53.92499999726881299, 164.1591823560292198, 12.60653300113718167 ) ) ;
#2492=CARTESIAN_POINT ( 'NONE',  ( 55.52499999726881441, 169.8198683612136222, -4.815267126137197984 ) ) ;
#2493=CARTESIAN_POINT ( 'NONE',  ( 71.17499999726881299, 145.8408176439707802, -12.60653300113719588 ) ) ;
#2500=CARTESIAN_POINT ( 'NONE',  ( 32.50000000000000000, 155.0000000000000000, 15.00000000000001243 ) ) ;
#2505=ORIENTED_EDGE ( 'NONE', *, *, #6759, .F. ) ;
#2508=EDGE_LOOP ( 'NONE', ( #32994, #9884, #9445, #29988 ) ) ;
#2509=CARTESIAN_POINT ( 'NONE',  ( 76.47499999726881015, 149.9369285172503510, 15.58253174999999580 ) ) ;
#2511=EDGE_LOOP ( 'NONE', ( #2793, #21886, #22794, #18548 ) ) ;
#2512=CARTESIAN_POINT ( 'NONE',  ( 73.32499999726880446, 164.1591823560292198, -12.60653300113719766 ) ) ;
#2514=CARTESIAN_POINT ( 'NONE',  ( 125.5000000000000000, 155.0000000000010800, 106.0000000000000142 ) ) ;
#2515=CARTESIAN_POINT ( 'NONE',  ( 65.12499999726881583, 155.0000000000000000, -15.58253175000000823 ) ) ;
#2527=CARTESIAN_POINT ( 'NONE',  ( 45.68867513459483121, 159.8737954434933499, 15.00000000000019895 ) ) ;
#2533=CARTESIAN_POINT ( 'NONE',  ( 45.88867513459483405, 150.1262045565061385, 14.99999999999982947 ) ) ;
#2535=CARTESIAN_POINT ( 'NONE',  ( 37.82499999726881157, 168.2552932293087906, 9.630534252274372875 ) ) ;
#2544=CARTESIAN_POINT ( 'NONE',  ( 71.49999999453763166, 139.7537977485451393, -4.138211985947621020E-15 ) ) ;
#2550=ORIENTED_EDGE ( 'NONE', *, *, #8975, .F. ) ;
#2553=ORIENTED_EDGE ( 'NONE', *, *, #21809, .T. ) ;
#2557=CARTESIAN_POINT ( 'NONE',  ( 55.98867513459482126, 146.1832212156128890, 12.13525491562421976 ) ) ;
#2558=ORIENTED_EDGE ( 'NONE', *, *, #13893, .F. ) ;
#2562=CARTESIAN_POINT ( 'NONE',  ( 60.47499999726880304, 149.9369285172503510, 15.58253174999999580 ) ) ;
#2563=EDGE_LOOP ( 'NONE', ( #6399, #7677, #30970, #31090 ) ) ;
#2576=CARTESIAN_POINT ( 'NONE',  ( 35.02499999726880020, 149.9369285172503510, -15.58253175000000823 ) ) ;
#2580=CARTESIAN_POINT ( 'NONE',  ( 48.08867513459482268, 142.2402378747194405, 9.270509831248432420 ) ) ;
#2581=CARTESIAN_POINT ( 'NONE',  ( 49.77499999726880731, 169.8198683612136222, -4.815267126137197984 ) ) ;
#2584=CARTESIAN_POINT ( 'NONE',  ( 34.71132485994281325, 155.0000000000000000, 15.00000000000001243 ) ) ;
#2586=CARTESIAN_POINT ( 'NONE',  ( 65.61132485994279762, 150.1262045565062806, -14.99999999999993072 ) ) ;
#2587=CARTESIAN_POINT ( 'NONE',  ( 54.09999999453763309, 159.7113355953771077, -14.50000000000000888 ) ) ;
#2590=CARTESIAN_POINT ( 'NONE',  ( 47.71132485994280614, 155.0000000000000000, -15.00000000000002487 ) ) ;
#2592=CARTESIAN_POINT ( 'NONE',  ( 59.81132485994281467, 159.8737954434935489, -15.00000000000007638 ) ) ;
#2600=AXIS2_PLACEMENT_3D ( 'NONE', #18352, #25681, #4726 ) ;
#2605=CARTESIAN_POINT ( 'NONE',  ( 45.37499999726880873, 155.0000000000000000, -15.58253175000000823 ) ) ;
#2608=CARTESIAN_POINT ( 'NONE',  ( 47.82499999726881867, 168.2552932293087906, 9.630534252274372875 ) ) ;
#2609=DIRECTION ( 'NONE',  ( 0.000000000000000000, 0.000000000000000000, 1.000000000000000000 ) ) ;
#2612=CARTESIAN_POINT ( 'NONE',  ( 46.87499999726880873, 138.6155565068815463, -3.929120461958505118E-15 ) ) ;
#2615=DIRECTION ( 'NONE',  ( 1.000000000000000000, 0.000000000000000000, 0.000000000000000000 ) ) ;
#2616=CARTESIAN_POINT ( 'NONE',  ( 70.60000000000000853, 159.7113355953771077, -14.50000000000000888 ) ) ;
#2618=CARTESIAN_POINT ( 'NONE',  ( 37.78867513459481842, 155.0000000000000000, 15.00000000000001243 ) ) ;
#2625=CIRCLE ( 'NONE', #23284, 2.149999999999985256 ) ;
#2626=CARTESIAN_POINT ( 'NONE',  ( 69.02499999726880731, 149.9369285172503510, -15.58253175000000823 ) ) ;
#2629=CARTESIAN_POINT ( 'NONE',  ( 58.71132485994280614, 155.0000000000000000, 15.00000000000001243 ) ) ;
#2630=CARTESIAN_POINT ( 'NONE',  ( 86.67499999726878457, 141.7447067706911810, 9.630534252274376428 ) ) ;
#2634=ORIENTED_EDGE ( 'NONE', *, *, #11989, .T. ) ;
#2641=DIRECTION ( 'NONE',  ( -1.000000000000000000, -0.000000000000000000, 0.000000000000000000 ) ) ;
#2648=CARTESIAN_POINT ( 'NONE',  ( 55.91132485994280898, 163.8167787843871110, -12.13525491562423397 ) ) ;
#2650=CARTESIAN_POINT ( 'NONE',  ( 34.22499999726881015, 149.9369285172503510, 15.58253174999999580 ) ) ;
#2651=CARTESIAN_POINT ( 'NONE',  ( 82.32499999726880446, 145.8408176439707802, 12.60653300113718345 ) ) ;
#2657=CARTESIAN_POINT ( 'NONE',  ( 46.70000000000000284, 163.5228861582408797, -11.73074641843674470 ) ) ;
#2660=EDGE_CURVE ( 'NONE', #23167, #9113, #12785, .T. ) ;
#2661=CARTESIAN_POINT ( 'NONE',  ( 54.32499999726880446, 145.8408176439707802, 12.60653300113718345 ) ) ;
#2664=CARTESIAN_POINT ( 'NONE',  ( 56.52499999726881441, 140.1801316387863778, 4.815267126137185549 ) ) ;
#2665=CARTESIAN_POINT ( 'NONE',  ( 71.07499999726880446, 141.7447067706911810, -9.630534252274385310 ) ) ;
#2671=CARTESIAN_POINT ( 'NONE',  ( 85.38867513459483405, 169.2658477444273331, 4.635254915624208216 ) ) ;
#2689=ADVANCED_FACE ( 'NONE', ( #10408 ), #31346, .T. ) ;
#2690=CARTESIAN_POINT ( 'NONE',  ( 74.52499999726880731, 140.1801316387863778, 4.815267126137185549 ) ) ;
#2695=CARTESIAN_POINT ( 'NONE',  ( 62.22499999726881725, 149.9369285172503510, 15.58253174999999580 ) ) ;
#2701=CARTESIAN_POINT ( 'NONE',  ( 42.71132485994280614, 155.0000000000000000, 15.00000000000001243 ) ) ;
#2708=CARTESIAN_POINT ( 'NONE',  ( 87.17499999726881299, 145.8408176439707802, -12.60653300113719588 ) ) ;
#2710=CARTESIAN_POINT ( 'NONE',  ( 36.52499999726881441, 140.1801316387863778, 4.815267126137185549 ) ) ;
#2711=( BOUNDED_CURVE ( )  B_SPLINE_CURVE ( 2, ( #10898, #32162, #21275, #19055, #3548, #18730, #24503, #31671, #26391, #26547, #13941 ),
 .UNSPECIFIED., .F., .T. ) 
 B_SPLINE_CURVE_WITH_KNOTS ( ( 3, 2, 2, 2, 2, 3 ),
 ( 0.03571428571428574700, 0.03928571428571431962, 0.04285714285714289917, 0.04642857142857147179, 0.05000000000000005135, 0.05357142857142861703 ),
 .UNSPECIFIED. ) 
 CURVE ( )  GEOMETRIC_REPRESENTATION_ITEM ( )  RATIONAL_B_SPLINE_CURVE ( ( 0.9999999999999995559, 0.9510565162951538642, 1.000000000000000000, 0.9510565162951534202, 1.000000000000000000, 0.9510565162951534202, 1.000000000000000000, 0.9510565162951534202, 1.000000000000000000, 0.9510565162951527540, 1.000000000000000666 ) ) 
 REPRESENTATION_ITEM ( '' )  );
#2718=CARTESIAN_POINT ( 'NONE',  ( 80.89999999453763735, 159.7113355953771077, 14.49999999999999289 ) ) ;
#2722=EDGE_CURVE ( 'NONE', #6290, #15366, #17716, .T. ) ;
#2724=ADVANCED_FACE ( 'NONE', ( #3723 ), #21946, .T. ) ;
#2725=CARTESIAN_POINT ( 'NONE',  ( 48.98867513459481415, 163.8167787843871110, -12.13525491562423397 ) ) ;
#2726=VERTEX_POINT ( 'NONE', #13943 ) ;
#2732=DIRECTION ( 'NONE',  ( 1.000000000000000000, 0.000000000000000000, 0.000000000000000000 ) ) ;
#2738=CARTESIAN_POINT ( 'NONE',  ( 63.67499999726880588, 168.2552932293087906, -9.630534252274387086 ) ) ;
#2750=CARTESIAN_POINT ( 'NONE',  ( 83.70000000000000284, 146.4771138417591203, 11.73074641843673227 ) ) ;
#2751=DIRECTION ( 'NONE',  ( 1.000000000000000000, 0.000000000000000000, 0.000000000000000000 ) ) ;
#2754=CARTESIAN_POINT ( 'NONE',  ( 58.57499999726881157, 145.8408176439707802, 12.60653300113718345 ) ) ;
#2756=CARTESIAN_POINT ( 'NONE',  ( 87.82499999726881867, 168.2552932293087906, 9.630534252274372875 ) ) ;
#2759=CARTESIAN_POINT ( 'NONE',  ( 62.89999999453763024, 159.7113355953771077, 14.49999999999999289 ) ) ;
#2762=CARTESIAN_POINT ( 'NONE',  ( 37.78867513459481842, 155.0000000000000000, 15.00000000000001243 ) ) ;
#2765=CARTESIAN_POINT ( 'NONE',  ( 59.91132485994281609, 163.8167787843871110, -12.13525491562423397 ) ) ;
#2768=ORIENTED_EDGE ( 'NONE', *, *, #19308, .F. ) ;
#2775=CARTESIAN_POINT ( 'NONE',  ( 41.67499999726881299, 168.2552932293087906, -9.630534252274387086 ) ) ;
#2777=CARTESIAN_POINT ( 'NONE',  ( 52.92499999726881299, 145.8408176439707802, -12.60653300113719588 ) ) ;
#2781=CARTESIAN_POINT ( 'NONE',  ( 54.17499999726881299, 164.1591823560292198, 12.60653300113718167 ) ) ;
#2782=CARTESIAN_POINT ( 'NONE',  ( 78.81132485994281467, 150.1262045565064227, 15.00000000000001599 ) ) ;
#2785=CARTESIAN_POINT ( 'NONE',  ( 67.00000000000001421, 170.2462022514548323, -7.872454543227099337E-15 ) ) ;
#2789=CARTESIAN_POINT ( 'NONE',  ( 56.88867513459482694, 159.8737954434937478, -14.99999999999993072 ) ) ;
#2790=CARTESIAN_POINT ( 'NONE',  ( 38.67499999726879878, 141.7447067706911810, 9.630534252274376428 ) ) ;
#2792=CARTESIAN_POINT ( 'NONE',  ( 69.62499999726883004, 171.3844434931184253, -7.942151717890132712E-15 ) ) ;
#2793=ORIENTED_EDGE ( 'NONE', *, *, #5823, .T. ) ;
#2795=CARTESIAN_POINT ( 'NONE',  ( 36.69999999453762740, 167.3344367211045096, 8.961492836873468093 ) ) ;
#2805=CARTESIAN_POINT ( 'NONE',  ( 74.41132485994282320, 167.7597621252805880, 9.270509831248428867 ) ) ;
#2812=DIRECTION ( 'NONE',  ( -1.000000000000000000, -0.000000000000000000, -0.000000000000000000 ) ) ;
#2813=CARTESIAN_POINT ( 'NONE',  ( 33.47499999726881015, 160.0630714827496206, -15.58253175000000823 ) ) ;
#2817=CARTESIAN_POINT ( 'NONE',  ( 49.00000000000000711, 170.2462022514548323, -7.872454543227099337E-15 ) ) ;
#2820=CARTESIAN_POINT ( 'NONE',  ( 51.62499999726880873, 171.3844434931184253, -7.942151717890132712E-15 ) ) ;
#2823=CARTESIAN_POINT ( 'NONE',  ( 61.52499999726881441, 169.8198683612136222, -4.815267126137197984 ) ) ;
#2824=CARTESIAN_POINT ( 'NONE',  ( 70.07499999726881867, 168.2552932293087906, 9.630534252274372875 ) ) ;
#2838=CARTESIAN_POINT ( 'NONE',  ( 32.50000000000000000, 155.0000000000000000, -6.938893903907228378E-15 ) ) ;
#2840=VERTEX_POINT ( 'NONE', #24677 ) ;
#2843=CARTESIAN_POINT ( 'NONE',  ( 77.62499999726880162, 171.3844434931184253, -7.942151717890134290E-15 ) ) ;
#2848=CARTESIAN_POINT ( 'NONE',  ( 70.92499999726881299, 145.8408176439707802, -12.60653300113719588 ) ) ;
#2857=CARTESIAN_POINT ( 'NONE',  ( 125.5000000000000000, 229.9533188057749555, 74.95331880577313655 ) ) ;
#2862=CARTESIAN_POINT ( 'NONE',  ( 46.58867513459481557, 146.1832212156128890, -12.13525491562423042 ) ) ;
#2864=CARTESIAN_POINT ( 'NONE',  ( 38.42499999726880588, 141.7447067706911810, 9.630534252274376428 ) ) ;
#2871=CARTESIAN_POINT ( 'NONE',  ( 82.29999999453764303, 167.3344367211045096, -8.961492836873482304 ) ) ;
#2872=AXIS2_PLACEMENT_3D ( 'NONE', #19834, #9787, #4333 ) ;
#2876=AXIS2_PLACEMENT_3D ( 'NONE', #9612, #9277, #19670 ) ;
#2888=CARTESIAN_POINT ( 'NONE',  ( 65.27499999726880731, 149.9369285172503510, -15.58253175000000823 ) ) ;
#2892=FACE_OUTER_BOUND ( 'NONE', #5791, .T. ) ;
#2896=CARTESIAN_POINT ( 'NONE',  ( 32.50000000000000000, 155.0000000000000000, -6.938893903907228378E-15 ) ) ;
#2899=FACE_OUTER_BOUND ( 'NONE', #26462, .T. ) ;
#2903=CARTESIAN_POINT ( 'NONE',  ( 41.32499999726881157, 164.1591823560292198, -12.60653300113719766 ) ) ;
#2908=CARTESIAN_POINT ( 'NONE',  ( 55.57499999726881157, 164.1591823560292198, -12.60653300113719766 ) ) ;
#2912=CARTESIAN_POINT ( 'NONE',  ( 35.41132485994280898, 142.2402378747194405, -9.270509831248439525 ) ) ;
#2916=CARTESIAN_POINT ( 'NONE',  ( 58.29999999453762172, 167.3344367211045096, -8.961492836873482304 ) ) ;
#2923=CARTESIAN_POINT ( 'NONE',  ( 59.11132485994280472, 140.7341522555726669, 4.635254915624211769 ) ) ;
#2931=ORIENTED_EDGE ( 'NONE', *, *, #25842, .T. ) ;
#2934=CARTESIAN_POINT ( 'NONE',  ( 45.67499999726881299, 168.2552932293087906, -9.630534252274387086 ) ) ;
#2936=CARTESIAN_POINT ( 'NONE',  ( 50.32499999726881157, 145.8408176439707802, 12.60653300113718345 ) ) ;
#2941=CARTESIAN_POINT ( 'NONE',  ( 51.57499999726881157, 164.1591823560292198, -12.60653300113719766 ) ) ;
#2944=CARTESIAN_POINT ( 'NONE',  ( 44.48867513459482126, 142.2402378747194405, -9.270509831248439525 ) ) ;
#2945=EDGE_CURVE ( 'NONE', #21593, #29444, #28334, .T. ) ;
#2948=CARTESIAN_POINT ( 'NONE',  ( 72.39999999999999147, 150.2886644046228639, -14.50000000000000888 ) ) ;
#2952=CARTESIAN_POINT ( 'NONE',  ( 86.58867513459482268, 146.1832212156128890, -12.13525491562423042 ) ) ;
#2954=CARTESIAN_POINT ( 'NONE',  ( 35.47499999726880304, 160.0630714827496206, -15.58253175000000823 ) ) ;
#2957=CARTESIAN_POINT ( 'NONE',  ( 70.72499999726881015, 140.1801316387863778, -4.815267126137194431 ) ) ;
#2960=CARTESIAN_POINT ( 'NONE',  ( 43.99999999453763166, 155.0000000000000000, -14.50000000000000711 ) ) ;
#2972=VECTOR ( 'NONE', #3685, 1000.000000000000000 ) ;
#2973=ORIENTED_EDGE ( 'NONE', *, *, #2722, .T. ) ;
#2978=CARTESIAN_POINT ( 'NONE',  ( 33.82499999726880446, 168.2552932293087906, 9.630534252274372875 ) ) ;
#2979=CARTESIAN_POINT ( 'NONE',  ( 35.87499999726881583, 171.3844434931184253, -7.942151717890132712E-15 ) ) ;
#2982=CARTESIAN_POINT ( 'NONE',  ( 45.90000000000000568, 141.2096805137202580, 4.480746418436733158 ) ) ;
#2984=CARTESIAN_POINT ( 'NONE',  ( 84.61132485994284025, 159.8737954434934920, 15.00000000000010836 ) ) ;
#2985=CARTESIAN_POINT ( 'NONE',  ( 49.82499999726881157, 168.2552932293087906, 9.630534252274372875 ) ) ;
#2988=CARTESIAN_POINT ( 'NONE',  ( 63.42499999726880588, 168.2552932293087906, -9.630534252274387086 ) ) ;
#2989=CARTESIAN_POINT ( 'NONE',  ( 74.87499999726880162, 138.6155565068815463, -3.929120461958505118E-15 ) ) ;
#2994=CARTESIAN_POINT ( 'NONE',  ( 54.28867513459483973, 139.2280666364260071, -4.041636747397287284E-15 ) ) ;
#2995=ORIENTED_EDGE ( 'NONE', *, *, #16665, .F. ) ;
#2999=CARTESIAN_POINT ( 'NONE',  ( 34.38867513459481273, 140.7341522555726669, -4.635254915624220651 ) ) ;
#3004=EDGE_LOOP ( 'NONE', ( #12042, #25746, #10651, #21637 ) ) ;
#3009=CARTESIAN_POINT ( 'NONE',  ( 80.02499999726880731, 160.0630714827496206, 15.58253174999999224 ) ) ;
#3011=CARTESIAN_POINT ( 'NONE',  ( 66.92499999726881299, 145.8408176439707802, -12.60653300113719588 ) ) ;
#3022=CARTESIAN_POINT ( 'NONE',  ( 46.68867513459483121, 150.1262045565065364, -15.00000000000012434 ) ) ;
#3024=CARTESIAN_POINT ( 'NONE',  ( 47.12499999726880873, 155.0000000000000000, -15.58253175000000823 ) ) ;
#3026=DIRECTION ( 'NONE',  ( 1.000000000000000000, 0.000000000000000000, 0.000000000000000000 ) ) ;
#3032=CARTESIAN_POINT ( 'NONE',  ( 80.29999999453761461, 167.3344367211045096, -8.961492836873482304 ) ) ;
#3037=CARTESIAN_POINT ( 'NONE',  ( 49.78867513459482552, 155.0000000000000000, 15.00000000000001243 ) ) ;
#3043=CARTESIAN_POINT ( 'NONE',  ( 74.37499999726881583, 155.0000000000000000, 15.58253174999999402 ) ) ;
#3044=CARTESIAN_POINT ( 'NONE',  ( 87.44295828238632851, 168.4482970619196465, 7.151417191984575261 ) ) ;
#3045=CARTESIAN_POINT ( 'NONE',  ( 58.88867513459481984, 159.8737954434936057, -15.00000000000002665 ) ) ;
#3048=CARTESIAN_POINT ( 'NONE',  ( 65.77499999726880731, 169.8198683612136222, -4.815267126137197984 ) ) ;
#3050=CARTESIAN_POINT ( 'NONE',  ( 32.50000000000000000, 155.0000000000000000, -15.00000000000002487 ) ) ;
#3053=EDGE_CURVE ( 'NONE', #17895, #28642, #26860, .T. ) ;
#3055=CARTESIAN_POINT ( 'NONE',  ( 80.41132485994282320, 167.7597621252805880, 9.270509831248428867 ) ) ;
#3057=CARTESIAN_POINT ( 'NONE',  ( 86.87499999726880162, 138.6155565068815463, -3.929120461958505118E-15 ) ) ;
#3060=CARTESIAN_POINT ( 'NONE',  ( 37.52499999726881441, 169.8198683612136222, -4.815267126137197984 ) ) ;
#3061=CARTESIAN_POINT ( 'NONE',  ( 81.08867513459485110, 167.7597621252805880, -9.270509831248443078 ) ) ;
#3065=CARTESIAN_POINT ( 'NONE',  ( 58.67499999726882010, 141.7447067706911810, 9.630534252274376428 ) ) ;
#3073=CARTESIAN_POINT ( 'NONE',  ( 65.71132485994280614, 155.0000000000000000, -15.00000000000002487 ) ) ;
#3074=CARTESIAN_POINT ( 'NONE',  ( 59.59999999453763309, 141.2096805137202580, -4.480746418436742040 ) ) ;
#3075=ORIENTED_EDGE ( 'NONE', *, *, #3497, .T. ) ;
#3079=CARTESIAN_POINT ( 'NONE',  ( 71.81132485994281467, 159.8737954434934920, -15.00000000000012434 ) ) ;
#3086=CARTESIAN_POINT ( 'NONE',  ( 43.91132485994281609, 163.8167787843871110, -12.13525491562423397 ) ) ;
#3091=CARTESIAN_POINT ( 'NONE',  ( 46.67499999726881299, 141.7447067706911810, 9.630534252274376428 ) ) ;
#3092=VERTEX_POINT ( 'NONE', #17508 ) ;
#3093=CARTESIAN_POINT ( 'NONE',  ( 48.42499999726881299, 141.7447067706911810, 9.630534252274376428 ) ) ;
#3095=CARTESIAN_POINT ( 'NONE',  ( 61.78867513459482552, 155.0000000000000000, 15.00000000000001243 ) ) ;
#3099=CARTESIAN_POINT ( 'NONE',  ( 53.97499999726881015, 169.8198683612136222, 4.815267126137181997 ) ) ;
#3101=CARTESIAN_POINT ( 'NONE',  ( 81.71132485994280614, 155.0000000000000000, -15.00000000000002487 ) ) ;
#3103=CARTESIAN_POINT ( 'NONE',  ( 76.30000000000001137, 146.4771138417591203, -11.73074641843674470 ) ) ;
#3104=CARTESIAN_POINT ( 'NONE',  ( 40.38867513459481984, 140.7341522555726669, -4.635254915624220651 ) ) ;
#3105=CARTESIAN_POINT ( 'NONE',  ( 32.50000000000000000, 155.0000000000000000, -6.938893903907228378E-15 ) ) ;
#3107=CARTESIAN_POINT ( 'NONE',  ( 86.38867513459483405, 140.7341522555726669, -4.635254915624220651 ) ) ;
#3108=CARTESIAN_POINT ( 'NONE',  ( 41.07499999726881157, 141.7447067706911810, -9.630534252274385310 ) ) ;
#3110=CARTESIAN_POINT ( 'NONE',  ( 80.02499999726882152, 160.0630714827496206, 15.58253174999999402 ) ) ;
#3113=CARTESIAN_POINT ( 'NONE',  ( 39.19999999453763451, 146.4771138417591203, 11.73074641843673227 ) ) ;
#3119=CIRCLE ( 'NONE', #22153, 15.00000000000001776 ) ;
#3122=CARTESIAN_POINT ( 'NONE',  ( 32.50000000000000000, 155.0000000000000000, -6.938893903907228378E-15 ) ) ;
#3138=VECTOR ( 'NONE', #1838, 1000.000000000000000 ) ;
#3140=CARTESIAN_POINT ( 'NONE',  ( 33.57499999726881157, 164.1591823560292198, -12.60653300113719766 ) ) ;
#3143=CARTESIAN_POINT ( 'NONE',  ( 52.50000000000000711, 155.0000000000000000, -14.50000000000000711 ) ) ;
#3147=CARTESIAN_POINT ( 'NONE',  ( 52.62499999726880162, 138.6155565068815463, -3.929120461958505118E-15 ) ) ;
#3151=CARTESIAN_POINT ( 'NONE',  ( 65.52499999726880731, 169.8198683612136222, -4.815267126137197984 ) ) ;
#3152=CARTESIAN_POINT ( 'NONE',  ( 75.57499999726881867, 164.1591823560292198, -12.60653300113719766 ) ) ;
#3156=CARTESIAN_POINT ( 'NONE',  ( 83.78867513459482552, 155.0000000000000000, 15.00000000000001243 ) ) ;
#3171=ORIENTED_EDGE ( 'NONE', *, *, #30012, .F. ) ;
#3173=CARTESIAN_POINT ( 'NONE',  ( 78.32499999726881867, 145.8408176439707802, 12.60653300113718345 ) ) ;
#3174=CARTESIAN_POINT ( 'NONE',  ( 33.68749999590321664, 155.0000000000000000, -15.04126587500000767 ) ) ;
#3177=CARTESIAN_POINT ( 'NONE',  ( 69.22499999726881015, 160.0630714827496206, -15.58253175000000823 ) ) ;
#3180=CARTESIAN_POINT ( 'NONE',  ( 38.60000000000000853, 159.7113355953771077, -14.50000000000000888 ) ) ;
#3184=CARTESIAN_POINT ( 'NONE',  ( 125.5000000000000000, 229.9533188057739039, -74.95331880577418815 ) ) ;
#3187=AXIS2_PLACEMENT_3D ( 'NONE', #9813, #33313, #23093 ) ;
#3192=CARTESIAN_POINT ( 'NONE',  ( 44.32499999726881157, 145.8408176439707802, 12.60653300113718345 ) ) ;
#3200=CARTESIAN_POINT ( 'NONE',  ( 78.19999999453763451, 163.5228861582408797, -11.73074641843674470 ) ) ;
#3209=CARTESIAN_POINT ( 'NONE',  ( 79.07499999726881867, 141.7447067706911810, -9.630534252274387086 ) ) ;
#3210=CARTESIAN_POINT ( 'NONE',  ( 52.81132485994281467, 150.1262045565065364, 15.00000000000011191 ) ) ;
#3214=EDGE_CURVE ( 'NONE', #18911, #30462, #12231, .T. ) ;
#3216=CARTESIAN_POINT ( 'NONE',  ( 66.77499999726880731, 140.1801316387863778, 4.815267126137185549 ) ) ;
#3224=CARTESIAN_POINT ( 'NONE',  ( 82.07499999726880446, 168.2552932293087906, 9.630534252274372875 ) ) ;
#3226=CARTESIAN_POINT ( 'NONE',  ( 36.52499999726881441, 140.1801316387863778, 4.815267126137185549 ) ) ;
#3232=CARTESIAN_POINT ( 'NONE',  ( 56.57499999726881157, 145.8408176439707802, 12.60653300113718345 ) ) ;
#3238=CARTESIAN_POINT ( 'NONE',  ( 60.19999999453762740, 163.5228861582408797, -11.73074641843674470 ) ) ;
#3241=CARTESIAN_POINT ( 'NONE',  ( 36.78867513459482552, 155.0000000000000000, -15.00000000000002487 ) ) ;
#3254=CARTESIAN_POINT ( 'NONE',  ( 40.77499999726881441, 140.1801316387863778, 4.815267126137185549 ) ) ;
#3255=VERTEX_POINT ( 'NONE', #10033 ) ;
#3256=CARTESIAN_POINT ( 'NONE',  ( 49.92499999726881299, 164.1591823560292198, 12.60653300113718167 ) ) ;
#3261=CARTESIAN_POINT ( 'NONE',  ( 55.07499999726879736, 141.7447067706911810, -9.630534252274385310 ) ) ;
#3266=CARTESIAN_POINT ( 'NONE',  ( 76.50000000000001421, 155.0000000000000000, -14.50000000000000711 ) ) ;
#3268=DIRECTION ( 'NONE',  ( 1.000000000000000000, 0.000000000000000000, 0.000000000000000000 ) ) ;
#3271=CARTESIAN_POINT ( 'NONE',  ( 38.57499999726881157, 145.8408176439707802, 12.60653300113718345 ) ) ;
#3273=CARTESIAN_POINT ( 'NONE',  ( 77.22499999726881015, 160.0630714827496206, -15.58253175000000823 ) ) ;
#3276=CARTESIAN_POINT ( 'NONE',  ( 40.19999999453763451, 163.5228861582408797, -11.73074641843674470 ) ) ;
#3282=VERTEX_POINT ( 'NONE', #28418 ) ;
#3287=ADVANCED_FACE ( 'NONE', ( #15293 ), #30809, .T. ) ;
#3298=CARTESIAN_POINT ( 'NONE',  ( 37.27499999726880020, 149.9369285172503510, -15.58253175000000823 ) ) ;
#3302=CARTESIAN_POINT ( 'NONE',  ( 53.90000000000000568, 141.2096805137202580, 4.480746418436733158 ) ) ;
#3306=CARTESIAN_POINT ( 'NONE',  ( 54.82499999726879736, 141.7447067706911810, -9.630534252274385310 ) ) ;
#3310=CARTESIAN_POINT ( 'NONE',  ( 65.42499999726881299, 168.2552932293087906, -9.630534252274387086 ) ) ;
#3311=CARTESIAN_POINT ( 'NONE',  ( 76.37499999726881583, 155.0000000000000000, 15.58253174999999402 ) ) ;
#3326=ORIENTED_EDGE ( 'NONE', *, *, #17837, .F. ) ;
#3332=CARTESIAN_POINT ( 'NONE',  ( 76.02499999726880731, 160.0630714827496206, 15.58253174999999224 ) ) ;
#3337=CARTESIAN_POINT ( 'NONE',  ( 68.02499999726882152, 160.0630714827496206, 15.58253174999999402 ) ) ;
#3341=CARTESIAN_POINT ( 'NONE',  ( 36.00000000000000711, 139.7537977485451393, -4.138211985947621020E-15 ) ) ;
#3345=EDGE_CURVE ( 'NONE', #27265, #28748, #10942, .T. ) ;
#3350=CARTESIAN_POINT ( 'NONE',  ( 43.52499999726881441, 169.8198683612136222, -4.815267126137197984 ) ) ;
#3352=LINE ( 'NONE', #24476, #16227 ) ;
#3359=CARTESIAN_POINT ( 'NONE',  ( 77.19999999453763451, 146.4771138417591203, 11.73074641843673227 ) ) ;
#3367=ORIENTED_EDGE ( 'NONE', *, *, #21211, .T. ) ;
#3369=ORIENTED_EDGE ( 'NONE', *, *, #9298, .F. ) ;
#3370=CARTESIAN_POINT ( 'NONE',  ( 76.77499999726880731, 140.1801316387863778, 4.815267126137185549 ) ) ;
#3371=DIRECTION ( 'NONE',  ( 0.000000000000000000, 0.000000000000000000, -1.000000000000000000 ) ) ;
#3376=CARTESIAN_POINT ( 'NONE',  ( 66.87499999726880162, 138.6155565068815747, -3.929120461958505118E-15 ) ) ;
#3380=CARTESIAN_POINT ( 'NONE',  ( 32.50000000000000000, 155.0000000000000000, -6.938893903907228378E-15 ) ) ;
#3385=CARTESIAN_POINT ( 'NONE',  ( 86.47499999726879594, 149.9369285172503510, 15.58253174999999580 ) ) ;
#3389=CARTESIAN_POINT ( 'NONE',  ( 38.72499999726881015, 140.1801316387863778, -4.815267126137194431 ) ) ;
#3390=CARTESIAN_POINT ( 'NONE',  ( 80.98867513459481415, 163.8167787843871110, -12.13525491562423397 ) ) ;
#3394=CARTESIAN_POINT ( 'NONE',  ( 61.87499999726881583, 171.3844434931184253, -7.942151717890132712E-15 ) ) ;
#3401=CARTESIAN_POINT ( 'NONE',  ( 61.39999999453763024, 141.2096805137202580, 4.480746418436733158 ) ) ;
#3404=CARTESIAN_POINT ( 'NONE',  ( 76.91132485994280898, 146.1832212156128890, 12.13525491562421976 ) ) ;
#3406=CARTESIAN_POINT ( 'NONE',  ( 72.11132485994281183, 169.2658477444273331, -4.635254915624224203 ) ) ;
#3409=ORIENTED_EDGE ( 'NONE', *, *, #14549, .F. ) ;
#3418=CIRCLE ( 'NONE', #12698, 2.149999999999985256 ) ;
#3419=CARTESIAN_POINT ( 'NONE',  ( 47.87499999726880162, 171.3844434931184253, -7.942151717890134290E-15 ) ) ;
#3421=CARTESIAN_POINT ( 'NONE',  ( 58.22499999726881015, 149.9369285172503510, 15.58253174999999580 ) ) ;
#3424=CARTESIAN_POINT ( 'NONE',  ( 77.71132485994280614, 155.0000000000000000, -15.00000000000002487 ) ) ;
#3426=CARTESIAN_POINT ( 'NONE',  ( 57.07499999726879736, 141.7447067706911810, -9.630534252274385310 ) ) ;
#3428=CARTESIAN_POINT ( 'NONE',  ( 47.58867513459481557, 163.8167787843871110, 12.13525491562421621 ) ) ;
#3431=CARTESIAN_POINT ( 'NONE',  ( 71.50000000000001421, 155.0000000000000000, 14.49999999999999467 ) ) ;
#3432=CARTESIAN_POINT ( 'NONE',  ( 64.78867513459482552, 155.0000000000000000, -15.00000000000002487 ) ) ;
#3435=CARTESIAN_POINT ( 'NONE',  ( 33.58867513459482268, 163.8167787843871110, 12.13525491562421621 ) ) ;
#3436=CARTESIAN_POINT ( 'NONE',  ( 37.77499999726881441, 169.8198683612136222, -4.815267126137197984 ) ) ;
#3438=CARTESIAN_POINT ( 'NONE',  ( 78.32499999726881867, 145.8408176439707802, 12.60653300113718345 ) ) ;
#3441=CARTESIAN_POINT ( 'NONE',  ( 39.99999999453762456, 155.0000000000000000, -14.50000000000000711 ) ) ;
#3448=ORIENTED_EDGE ( 'NONE', *, *, #24308, .F. ) ;
#3455=CARTESIAN_POINT ( 'NONE',  ( 50.08867513459482268, 142.2402378747194405, 9.270509831248432420 ) ) ;
#3460=CARTESIAN_POINT ( 'NONE',  ( 33.47499999726881015, 160.0630714827496206, -15.58253175000000823 ) ) ;
#3461=VERTEX_POINT ( 'NONE', #30987 ) ;
#3462=CARTESIAN_POINT ( 'NONE',  ( 37.82499999726881157, 168.2552932293087906, 9.630534252274372875 ) ) ;
#3466=CARTESIAN_POINT ( 'NONE',  ( 35.97499999726881015, 169.8198683612136222, 4.815267126137181997 ) ) ;
#3471=CARTESIAN_POINT ( 'NONE',  ( 52.80000000000000426, 167.3344367211045096, -8.961492836873482304 ) ) ;
#3475=CARTESIAN_POINT ( 'NONE',  ( 56.12499999726880873, 155.0000000000000000, 15.58253174999999402 ) ) ;
#3480=CARTESIAN_POINT ( 'NONE',  ( 64.52499999726882152, 140.1801316387863778, 4.815267126137185549 ) ) ;
#3481=CARTESIAN_POINT ( 'NONE',  ( 77.17499999726881299, 145.8408176439707802, -12.60653300113719588 ) ) ;
#3485=CARTESIAN_POINT ( 'NONE',  ( 83.88867513459483405, 150.1262045565062238, 14.99999999999988454 ) ) ;
#3486=VERTEX_POINT ( 'NONE', #18026 ) ;
#3497=EDGE_CURVE ( 'NONE', #8044, #608, #15529, .T. ) ;
#3498=CARTESIAN_POINT ( 'NONE',  ( 39.11132485994280472, 140.7341522555726669, 4.635254915624211769 ) ) ;
#3503=CARTESIAN_POINT ( 'NONE',  ( 79.02499999726879309, 149.9369285172503510, -15.58253175000000823 ) ) ;
#3504=ORIENTED_EDGE ( 'NONE', *, *, #3552, .F. ) ;
#3506=CARTESIAN_POINT ( 'NONE',  ( 70.72499999726881015, 140.1801316387863778, -4.815267126137194431 ) ) ;
#3510=CARTESIAN_POINT ( 'NONE',  ( 57.71132485994280614, 155.0000000000000000, -15.00000000000002487 ) ) ;
#3511=CARTESIAN_POINT ( 'NONE',  ( 33.30000000000000426, 163.5228861582408797, 11.73074641843673049 ) ) ;
#3518=CARTESIAN_POINT ( 'NONE',  ( 59.98867513459482836, 146.1832212156128890, 12.13525491562421976 ) ) ;
#3519=CARTESIAN_POINT ( 'NONE',  ( 41.52499999726881441, 169.8198683612136222, -4.815267126137197984 ) ) ;
#3526=CARTESIAN_POINT ( 'NONE',  ( 84.89999999453762314, 159.7113355953771077, 14.49999999999999289 ) ) ;
#3536=ADVANCED_FACE ( 'NONE', ( #2016 ), #12405, .T. ) ;
#3538=CARTESIAN_POINT ( 'NONE',  ( 79.87499999726880162, 171.3844434931184253, -7.942151717890134290E-15 ) ) ;
#3540=DIRECTION ( 'NONE',  ( 0.000000000000000000, -0.7071067811865475727, -0.7071067811865475727 ) ) ;
#3546=CARTESIAN_POINT ( 'NONE',  ( 67.17499999726881299, 145.8408176439707802, -12.60653300113719588 ) ) ;
#3548=CARTESIAN_POINT ( 'NONE',  ( 36.11132485994280472, 169.2658477444273331, -4.635254915624224203 ) ) ;
#3549=CARTESIAN_POINT ( 'NONE',  ( 52.48867513459483547, 142.2402378747194405, -9.270509831248439525 ) ) ;
#3550=CARTESIAN_POINT ( 'NONE',  ( 43.28867513459483263, 170.7719333635740497, -7.904646289410545231E-15 ) ) ;
#3552=EDGE_CURVE ( 'NONE', #20942, #5021, #26704, .T. ) ;
#3554=CARTESIAN_POINT ( 'NONE',  ( 83.08867513459485110, 167.7597621252805880, -9.270509831248443078 ) ) ;
#3557=CARTESIAN_POINT ( 'NONE',  ( 82.87499999726878741, 138.6155565068815463, -3.929120461958505118E-15 ) ) ;
#3560=CARTESIAN_POINT ( 'NONE',  ( 35.72499999726881015, 169.8198683612136222, 4.815267126137181997 ) ) ;
#3565=CARTESIAN_POINT ( 'NONE',  ( 61.37499999726880873, 155.0000000000000000, -15.58253175000000823 ) ) ;
#3572=CARTESIAN_POINT ( 'NONE',  ( 65.59999999453764019, 141.2096805137202580, -4.480746418436742040 ) ) ;
#3582=DIRECTION ( 'NONE',  ( 1.000000000000000000, 0.000000000000000000, 0.000000000000000000 ) ) ;
#3588=CARTESIAN_POINT ( 'NONE',  ( 50.27499999726880731, 160.0630714827496206, 15.58253174999999224 ) ) ;
#3590=CARTESIAN_POINT ( 'NONE',  ( 55.32499999726881157, 164.1591823560292198, -12.60653300113719766 ) ) ;
#3595=CARTESIAN_POINT ( 'NONE',  ( 56.97499999726881015, 140.1801316387863778, -4.815267126137194431 ) ) ;
#3600=CARTESIAN_POINT ( 'NONE',  ( 72.20000000000001705, 142.6655632788954620, -8.961492836873480528 ) ) ;
#3601=CARTESIAN_POINT ( 'NONE',  ( 62.41132485994282320, 167.7597621252805880, 9.270509831248428867 ) ) ;
#3602=DIRECTION ( 'NONE',  ( 0.000000000000000000, 0.000000000000000000, -1.000000000000000000 ) ) ;
#3604=CARTESIAN_POINT ( 'NONE',  ( 32.88867513459483405, 159.8737954434936057, -15.00000000000002665 ) ) ;
#3605=CARTESIAN_POINT ( 'NONE',  ( 44.57499999726881157, 145.8408176439707802, 12.60653300113718345 ) ) ;
#3608=CARTESIAN_POINT ( 'NONE',  ( 79.12499999726881583, 155.0000000000000000, -15.58253175000000823 ) ) ;
#3610=CARTESIAN_POINT ( 'NONE',  ( 38.71132485994280614, 155.0000000000000000, 15.00000000000001243 ) ) ;
#3611=CARTESIAN_POINT ( 'NONE',  ( 41.29999999453762172, 142.6655632788954620, 8.961492836873471646 ) ) ;
#3615=VERTEX_POINT ( 'NONE', #24599 ) ;
#3623=CARTESIAN_POINT ( 'NONE',  ( 78.88867513459481984, 159.8737954434934636, -15.00000000000014566 ) ) ;
#3628=AXIS2_PLACEMENT_3D ( 'NONE', #25975, #2812, #31427 ) ;
#3629=EDGE_LOOP ( 'NONE', ( #398, #22472, #28449, #10571 ) ) ;
#3630=CARTESIAN_POINT ( 'NONE',  ( 40.22499999726880304, 149.9369285172503510, 15.58253174999999580 ) ) ;
#3632=CARTESIAN_POINT ( 'NONE',  ( 40.97499999726881725, 140.1801316387863778, -4.815267126137194431 ) ) ;
#3636=CARTESIAN_POINT ( 'NONE',  ( 56.39999999999999858, 150.2886644046228639, -14.50000000000000888 ) ) ;
#3642=CARTESIAN_POINT ( 'NONE',  ( 57.42499999726880588, 168.2552932293087906, -9.630534252274385310 ) ) ;
#3645=CARTESIAN_POINT ( 'NONE',  ( 37.71132485994279904, 155.0000000000000000, -15.00000000000002487 ) ) ;
#3646=CARTESIAN_POINT ( 'NONE',  ( 67.22499999726879594, 160.0630714827496206, -15.58253175000000823 ) ) ;
#3647=CARTESIAN_POINT ( 'NONE',  ( 78.47499999726881015, 149.9369285172503510, 15.58253174999999580 ) ) ;
#3666=VERTEX_POINT ( 'NONE', #19484 ) ;
#3668=CARTESIAN_POINT ( 'NONE',  ( 84.02499999726880731, 160.0630714827496206, 15.58253174999999224 ) ) ;
#3672=CARTESIAN_POINT ( 'NONE',  ( 78.42499999726882720, 141.7447067706911810, 9.630534252274376428 ) ) ;
#3677=CARTESIAN_POINT ( 'NONE',  ( 35.59999999999998721, 150.2886644046228639, 14.49999999999999645 ) ) ;
#3685=DIRECTION ( 'NONE',  ( 1.000000000000000000, 0.000000000000000000, 0.000000000000000000 ) ) ;
#3686=CARTESIAN_POINT ( 'NONE',  ( 48.72499999726881725, 140.1801316387863778, -4.815267126137194431 ) ) ;
#3688=LINE ( 'NONE', #31967, #11346 ) ;
#3707=CARTESIAN_POINT ( 'NONE',  ( 73.47499999726878173, 160.0630714827496206, -15.58253175000000823 ) ) ;
#3711=CARTESIAN_POINT ( 'NONE',  ( 83.27499999726880731, 149.9369285172503510, -15.58253175000000823 ) ) ;
#3712=FACE_OUTER_BOUND ( 'NONE', #22728, .T. ) ;
#3718=CARTESIAN_POINT ( 'NONE',  ( 68.27499999726879309, 160.0630714827496206, 15.58253174999999224 ) ) ;
#3719=VERTEX_POINT ( 'NONE', #23798 ) ;
#3720=CARTESIAN_POINT ( 'NONE',  ( 41.48867513459482836, 167.7597621252805880, 9.270509831248428867 ) ) ;
#3723=FACE_OUTER_BOUND ( 'NONE', #11345, .T. ) ;
#3727=CARTESIAN_POINT ( 'NONE',  ( 84.27499999726879309, 160.0630714827496206, 15.58253174999999402 ) ) ;
#3730=CARTESIAN_POINT ( 'NONE',  ( 42.32499999726881157, 145.8408176439707802, 12.60653300113718345 ) ) ;
#3731=CARTESIAN_POINT ( 'NONE',  ( 36.18867513459482410, 140.7341522555726669, 4.635254915624211769 ) ) ;
#3735=EDGE_CURVE ( 'NONE', #23334, #3461, #16406, .T. ) ;
#3743=CARTESIAN_POINT ( 'NONE',  ( 66.89999999453763735, 159.7113355953771077, 14.49999999999999289 ) ) ;
#3748=EDGE_CURVE ( 'NONE', #6526, #30462, #26178, .T. ) ;
#3749=CARTESIAN_POINT ( 'NONE',  ( 73.78867513459483973, 155.0000000000000000, 15.00000000000001243 ) ) ;
#3755=ADVANCED_FACE ( 'NONE', ( #21863, #5412, #3980, #32256, #298, #28753, #27155, #26188, #23639, #21076 ), #8146, .F. ) ;
#3758=CARTESIAN_POINT ( 'NONE',  ( 49.71132485994280614, 155.0000000000000000, -15.00000000000002487 ) ) ;
#3764=CARTESIAN_POINT ( 'NONE',  ( 49.37499999726880873, 155.0000000000000000, -15.58253175000000823 ) ) ;
#3766=CARTESIAN_POINT ( 'NONE',  ( 56.22499999726881015, 149.9369285172503510, 15.58253174999999580 ) ) ;
#3773=CARTESIAN_POINT ( 'NONE',  ( 60.57499999726881157, 145.8408176439707802, 12.60653300113718345 ) ) ;
#3775=CARTESIAN_POINT ( 'NONE',  ( 73.48867513459482836, 167.7597621252805880, 9.270509831248428867 ) ) ;
#3777=CARTESIAN_POINT ( 'NONE',  ( 82.69999999999998863, 163.5228861582408797, -11.73074641843674470 ) ) ;
#3782=CARTESIAN_POINT ( 'NONE',  ( 46.57499999726881157, 145.8408176439707802, 12.60653300113718345 ) ) ;
#3785=CARTESIAN_POINT ( 'NONE',  ( 75.72499999726881015, 169.8198683612136222, 4.815267126137181997 ) ) ;
#3787=CARTESIAN_POINT ( 'NONE',  ( 51.91132485994280898, 163.8167787843871110, -12.13525491562423397 ) ) ;
#3788=CARTESIAN_POINT ( 'NONE',  ( 49.19999999453762740, 146.4771138417591203, 11.73074641843673227 ) ) ;
#3789=( BOUNDED_CURVE ( )  B_SPLINE_CURVE ( 2, ( #28884, #23443, #10670, #6975, #108, #18500, #7322, #12419, #4749, #22813, #17362 ),
 .UNSPECIFIED., .F., .F. ) 
 B_SPLINE_CURVE_WITH_KNOTS ( ( 3, 2, 2, 2, 2, 3 ),
 ( 0.9285714285714283811, 0.9321428571428569398, 0.9357142857142856096, 0.9392857142857141683, 0.9428571428571427271, 0.9464285714285712858 ),
 .UNSPECIFIED. ) 
 CURVE ( )  GEOMETRIC_REPRESENTATION_ITEM ( )  RATIONAL_B_SPLINE_CURVE ( ( 1.000000000000001554, 0.9510565162951518658, 1.000000000000000000, 0.9510565162951534202, 1.000000000000000000, 0.9510565162951534202, 1.000000000000000000, 0.9510565162951534202, 1.000000000000000000, 0.9510565162951549745, 0.9999999999999984457 ) ) 
 REPRESENTATION_ITEM ( '' )  );
#3799=DIRECTION ( 'NONE',  ( 0.000000000000000000, 0.000000000000000000, 1.000000000000000000 ) ) ;
#3804=DIRECTION ( 'NONE',  ( 1.000000000000000000, 0.000000000000000000, 0.000000000000000000 ) ) ;
#3806=CARTESIAN_POINT ( 'NONE',  ( 40.92499999726881299, 145.8408176439707802, -12.60653300113719588 ) ) ;
#3808=CARTESIAN_POINT ( 'NONE',  ( 43.27499999726880020, 149.9369285172503510, -15.58253175000000823 ) ) ;
#3811=CARTESIAN_POINT ( 'NONE',  ( 57.30000000000000426, 163.5228861582408797, 11.73074641843673049 ) ) ;
#3815=CARTESIAN_POINT ( 'NONE',  ( 59.22499999726879594, 160.0630714827496206, -15.58253175000000823 ) ) ;
#3819=CARTESIAN_POINT ( 'NONE',  ( 82.27499999726880731, 160.0630714827496206, 15.58253174999999402 ) ) ;
#3834=VERTEX_POINT ( 'NONE', #30389 ) ;
#3837=ORIENTED_EDGE ( 'NONE', *, *, #3748, .T. ) ;
#3839=CARTESIAN_POINT ( 'NONE',  ( 84.72499999726882436, 140.1801316387863778, -4.815267126137194431 ) ) ;
#3840=ORIENTED_EDGE ( 'NONE', *, *, #17060, .T. ) ;
#3842=CARTESIAN_POINT ( 'NONE',  ( 75.72499999726881015, 169.8198683612136222, 4.815267126137181997 ) ) ;
#3845=AXIS2_PLACEMENT_3D ( 'NONE', #20780, #31179, #18234 ) ;
#3846=CARTESIAN_POINT ( 'NONE',  ( 33.40000000000000568, 159.7113355953771077, 14.49999999999999289 ) ) ;
#3853=CARTESIAN_POINT ( 'NONE',  ( 50.82499999726880446, 141.7447067706911810, -9.630534252274387086 ) ) ;
#3855=CARTESIAN_POINT ( 'NONE',  ( 41.31132485994280756, 140.7341522555726669, -4.635254915624220651 ) ) ;
#3860=CARTESIAN_POINT ( 'NONE',  ( 88.89999999453763735, 159.7113355953771077, 14.49999999999999289 ) ) ;
#3870=CARTESIAN_POINT ( 'NONE',  ( 74.57499999726881867, 145.8408176439707802, 12.60653300113718345 ) ) ;
#3873=CARTESIAN_POINT ( 'NONE',  ( 80.67499999726882720, 141.7447067706911810, 9.630534252274376428 ) ) ;
#3879=CARTESIAN_POINT ( 'NONE',  ( 68.07499999726881867, 168.2552932293087906, 9.630534252274372875 ) ) ;
#3882=EDGE_CURVE ( 'NONE', #33037, #25104, #13144, .T. ) ;
#3889=CARTESIAN_POINT ( 'NONE',  ( 46.32499999726881157, 145.8408176439707802, 12.60653300113718345 ) ) ;
#3891=CARTESIAN_POINT ( 'NONE',  ( 33.52499999726880731, 169.8198683612136222, -4.815267126137197984 ) ) ;
#3893=LINE ( 'NONE', #22628, #30394 ) ;
#3901=CARTESIAN_POINT ( 'NONE',  ( 69.89999999453762314, 150.2886644046228639, -14.50000000000000888 ) ) ;
#3912=CARTESIAN_POINT ( 'NONE',  ( 41.98867513459482126, 146.1832212156128890, 12.13525491562421976 ) ) ;
#3917=( BOUNDED_CURVE ( )  B_SPLINE_CURVE ( 2, ( #16547, #21826, #26942, #31883, #8392, #27116, #8550, #3601, #16882, #13655, #11447 ),
 .UNSPECIFIED., .F., .T. ) 
 B_SPLINE_CURVE_WITH_KNOTS ( ( 3, 2, 2, 2, 2, 3 ),
 ( 0.5000000000000000000, 0.5035714285714285587, 0.5071428571428571175, 0.5107142857142856762, 0.5142857142857142350, 0.5178571428571429047 ),
 .UNSPECIFIED. ) 
 CURVE ( )  GEOMETRIC_REPRESENTATION_ITEM ( )  RATIONAL_B_SPLINE_CURVE ( ( 1.000000000000000000, 0.9510565162951534202, 1.000000000000000000, 0.9510565162951534202, 1.000000000000000000, 0.9510565162951534202, 1.000000000000000000, 0.9510565162951534202, 1.000000000000000000, 0.9510565162951534202, 1.000000000000000000 ) ) 
 REPRESENTATION_ITEM ( '' )  );
#3918=EDGE_CURVE ( 'NONE', #29444, #8938, #22718, .T. ) ;
#3919=CARTESIAN_POINT ( 'NONE',  ( 125.5000000000000000, 48.99999999999998579, -2.149999999999999023 ) ) ;
#3921=CARTESIAN_POINT ( 'NONE',  ( 52.87499999726880162, 138.6155565068815747, -3.929120461958505118E-15 ) ) ;
#3922=ORIENTED_EDGE ( 'NONE', *, *, #405, .F. ) ;
#3924=CARTESIAN_POINT ( 'NONE',  ( 67.31132485994281467, 140.7341522555726669, -4.635254915624220651 ) ) ;
#3930=CARTESIAN_POINT ( 'NONE',  ( 59.37499999726881583, 155.0000000000000000, -15.58253175000000823 ) ) ;
#3935=CARTESIAN_POINT ( 'NONE',  ( 83.40000000000000568, 159.7113355953771077, 14.49999999999999289 ) ) ;
#3939=CYLINDRICAL_SURFACE ( 'NONE', #8080, 2.149999999999994138 ) ;
#3940=CARTESIAN_POINT ( 'NONE',  ( 45.97499999726881015, 169.8198683612136222, 4.815267126137181997 ) ) ;
#3942=CARTESIAN_POINT ( 'NONE',  ( 85.32499999726880446, 164.1591823560292198, -12.60653300113719766 ) ) ;
#3946=DIRECTION ( 'NONE',  ( 1.000000000000000000, 0.000000000000000000, 0.000000000000000000 ) ) ;
#3947=CARTESIAN_POINT ( 'NONE',  ( 47.49999999453763166, 139.7537977485451393, -4.138211985947621020E-15 ) ) ;
#3960=CARTESIAN_POINT ( 'NONE',  ( 50.91132485994280188, 146.1832212156128890, 12.13525491562421976 ) ) ;
#3969=CARTESIAN_POINT ( 'NONE',  ( 36.42499999726879878, 141.7447067706911810, 9.630534252274376428 ) ) ;
#3970=CARTESIAN_POINT ( 'NONE',  ( 39.38867513459481984, 169.2658477444273331, 4.635254915624208216 ) ) ;
#3973=CARTESIAN_POINT ( 'NONE',  ( 39.37499999726880873, 155.0000000000000000, -15.58253175000000823 ) ) ;
#3976=EDGE_CURVE ( 'NONE', #5752, #5188, #32933, .T. ) ;
#3978=CARTESIAN_POINT ( 'NONE',  ( 61.30000000000000426, 163.5228861582408797, 11.73074641843673049 ) ) ;
#3979=( BOUNDED_CURVE ( )  B_SPLINE_CURVE ( 2, ( #26987, #29386, #16425, #5705, #16093, #26821, #26487, #19156, #32103, #3485, #3156 ),
 .UNSPECIFIED., .F., .F. ) 
 B_SPLINE_CURVE_WITH_KNOTS ( ( 3, 2, 2, 2, 2, 3 ),
 ( 0.05357142857142836723, 0.05714285714285691903, 0.06071428571428558185, 0.06428571428571414059, 0.06785714285714269933, 0.07142857142857124420 ),
 .UNSPECIFIED. ) 
 CURVE ( )  GEOMETRIC_REPRESENTATION_ITEM ( )  RATIONAL_B_SPLINE_CURVE ( ( 1.000000000000001776, 0.9510565162951518658, 1.000000000000000000, 0.9510565162951534202, 1.000000000000000000, 0.9510565162951534202, 1.000000000000000000, 0.9510565162951534202, 1.000000000000000000, 0.9510565162951555296, 0.9999999999999978906 ) ) 
 REPRESENTATION_ITEM ( '' )  );
#3980=FACE_BOUND ( 'NONE', #32570, .T. ) ;
#3985=VECTOR ( 'NONE', #12306, 1000.000000000000000 ) ;
#3986=CARTESIAN_POINT ( 'NONE',  ( 63.52499999726880731, 169.8198683612136222, -4.815267126137197984 ) ) ;
#3990=CARTESIAN_POINT ( 'NONE',  ( 84.87499999726881583, 138.6155565068815463, -3.929120461958505118E-15 ) ) ;
#3992=CARTESIAN_POINT ( 'NONE',  ( 72.08867513459482268, 142.2402378747194405, 9.270509831248432420 ) ) ;
#3993=CARTESIAN_POINT ( 'NONE',  ( 52.98867513459482126, 163.8167787843871110, -12.13525491562423397 ) ) ;
#4003=CARTESIAN_POINT ( 'NONE',  ( 39.41132485994281609, 142.2402378747194405, -9.270509831248439525 ) ) ;
#4010=AXIS2_PLACEMENT_3D ( 'NONE', #22014, #22687, #29681 ) ;
#4011=CARTESIAN_POINT ( 'NONE',  ( 85.92499999726881299, 164.1591823560292198, 12.60653300113718167 ) ) ;
#4013=CARTESIAN_POINT ( 'NONE',  ( 69.18867513459483121, 169.2658477444273331, -4.635254915624224203 ) ) ;
#4014=CARTESIAN_POINT ( 'NONE',  ( 73.82499999726879025, 168.2552932293087906, 9.630534252274372875 ) ) ;
#4017=CARTESIAN_POINT ( 'NONE',  ( 87.50000000000005684, 169.8972688042864831, 3.304339362361343291 ) ) ;
#4020=CARTESIAN_POINT ( 'NONE',  ( 39.39999999999999858, 159.7113355953771077, 14.49999999999999289 ) ) ;
#4023=DIRECTION ( 'NONE',  ( 1.000000000000000000, 0.000000000000000000, 0.000000000000000000 ) ) ;
#4026=CARTESIAN_POINT ( 'NONE',  ( 51.12499999726881583, 155.0000000000000000, -15.58253175000000823 ) ) ;
#4029=CARTESIAN_POINT ( 'NONE',  ( 40.81132485994281467, 150.1262045565064511, 15.00000000000004086 ) ) ;
#4035=CARTESIAN_POINT ( 'NONE',  ( 86.39999999453762314, 168.7903194862797420, -4.480746418436745593 ) ) ;
#4043=CARTESIAN_POINT ( 'NONE',  ( 72.27499999726879309, 160.0630714827496206, 15.58253174999999402 ) ) ;
#4046=CARTESIAN_POINT ( 'NONE',  ( 83.77499999726880731, 169.8198683612136222, -4.815267126137197984 ) ) ;
#4048=DIRECTION ( 'NONE',  ( -1.000000000000000000, 0.000000000000000000, 0.000000000000000000 ) ) ;
#4052=ORIENTED_EDGE ( 'NONE', *, *, #1445, .F. ) ;
#4060=CARTESIAN_POINT ( 'NONE',  ( 38.41132485994281609, 167.7597621252805880, 9.270509831248428867 ) ) ;
#4064=CARTESIAN_POINT ( 'NONE',  ( 45.22499999726881015, 160.0630714827496206, -15.58253175000000823 ) ) ;
#4065=DIRECTION ( 'NONE',  ( 1.000000000000000000, 0.000000000000000000, 0.000000000000000000 ) ) ;
#4068=CARTESIAN_POINT ( 'NONE',  ( 81.78867513459482552, 155.0000000000000000, 15.00000000000001243 ) ) ;
#4071=CARTESIAN_POINT ( 'NONE',  ( 75.98867513459481415, 146.1832212156128890, 12.13525491562421976 ) ) ;
#4075=CARTESIAN_POINT ( 'NONE',  ( 66.09999999453764019, 159.7113355953771077, -14.50000000000000888 ) ) ;
#4088=CARTESIAN_POINT ( 'NONE',  ( 87.50000000000001421, 166.8192717339189812, 9.236060614774261879 ) ) ;
#4090=CARTESIAN_POINT ( 'NONE',  ( 48.27499999726880731, 160.0630714827496206, 15.58253174999999224 ) ) ;
#4096=CARTESIAN_POINT ( 'NONE',  ( 57.37499999726880873, 155.0000000000000000, -15.58253175000000823 ) ) ;
#4098=FACE_OUTER_BOUND ( 'NONE', #14475, .T. ) ;
#4102=CARTESIAN_POINT ( 'NONE',  ( 77.30000000000001137, 163.5228861582408797, 11.73074641843673049 ) ) ;
#4106=CARTESIAN_POINT ( 'NONE',  ( 42.57499999726881157, 145.8408176439707802, 12.60653300113718345 ) ) ;
#4108=CARTESIAN_POINT ( 'NONE',  ( 83.72499999726882436, 169.8198683612136222, 4.815267126137181997 ) ) ;
#4112=CARTESIAN_POINT ( 'NONE',  ( 50.19999999453762740, 163.5228861582408797, -11.73074641843674470 ) ) ;
#4122=( BOUNDED_CURVE ( )  B_SPLINE_CURVE ( 2, ( #22651, #33038, #22484, #32366, #9709, #27931, #24710, #30493, #20098, #19420, #14811 ),
 .UNSPECIFIED., .F., .F. ) 
 B_SPLINE_CURVE_WITH_KNOTS ( ( 3, 2, 2, 2, 2, 3 ),
 ( 0.5178571428571427937, 0.5214285714285713524, 0.5249999999999999112, 0.5285714285714285809, 0.5321428571428571397, 0.5357142857142856984 ),
 .UNSPECIFIED. ) 
 CURVE ( )  GEOMETRIC_REPRESENTATION_ITEM ( )  RATIONAL_B_SPLINE_CURVE ( ( 1.000000000000000000, 0.9510565162951534202, 1.000000000000000000, 0.9510565162951534202, 1.000000000000000000, 0.9510565162951534202, 1.000000000000000000, 0.9510565162951534202, 1.000000000000000000, 0.9510565162951518658, 1.000000000000001554 ) ) 
 REPRESENTATION_ITEM ( '' )  );
#4133=CARTESIAN_POINT ( 'NONE',  ( 34.82499999726881157, 141.7447067706911810, -9.630534252274385310 ) ) ;
#4137=CARTESIAN_POINT ( 'NONE',  ( 39.97499999726881015, 169.8198683612136222, 4.815267126137181997 ) ) ;
#4141=CARTESIAN_POINT ( 'NONE',  ( 64.20000000000000284, 142.6655632788954620, -8.961492836873480528 ) ) ;
#4146=CARTESIAN_POINT ( 'NONE',  ( 64.72499999726881015, 140.1801316387863778, -4.815267126137194431 ) ) ;
#4150=CARTESIAN_POINT ( 'NONE',  ( 84.37499999726881583, 155.0000000000000000, 15.58253174999999402 ) ) ;
#4172=CARTESIAN_POINT ( 'NONE',  ( 83.32499999726880446, 164.1591823560292198, -12.60653300113719766 ) ) ;
#4174=CARTESIAN_POINT ( 'NONE',  ( 69.71132485994280614, 155.0000000000000000, -15.00000000000002487 ) ) ;
#4175=CARTESIAN_POINT ( 'NONE',  ( 76.02499999726880731, 160.0630714827496206, 15.58253174999999402 ) ) ;
#4181=CARTESIAN_POINT ( 'NONE',  ( 39.80000000000000426, 142.6655632788954620, 8.961492836873471646 ) ) ;
#4187=CARTESIAN_POINT ( 'NONE',  ( 52.02499999726880731, 160.0630714827496206, 15.58253174999999224 ) ) ;
#4188=CARTESIAN_POINT ( 'NONE',  ( 66.37499999726881583, 155.0000000000000000, 15.58253174999999402 ) ) ;
#4190=CARTESIAN_POINT ( 'NONE',  ( 32.50000000000000000, 155.0000000000000000, -6.938893903907228378E-15 ) ) ;
#4196=CARTESIAN_POINT ( 'NONE',  ( 87.59999999453762598, 141.2096805137202580, -4.480746418436742040 ) ) ;
#4204=AXIS2_PLACEMENT_3D ( 'NONE', #17502, #24834, #4388 ) ;
#4207=CARTESIAN_POINT ( 'NONE',  ( 70.57499999726881867, 145.8408176439707802, 12.60653300113718345 ) ) ;
#4210=CARTESIAN_POINT ( 'NONE',  ( 85.07499999726883289, 141.7447067706911810, -9.630534252274387086 ) ) ;
#4211=DIRECTION ( 'NONE',  ( 0.000000000000000000, 0.000000000000000000, -1.000000000000000000 ) ) ;
#4215=ORIENTED_EDGE ( 'NONE', *, *, #3882, .F. ) ;
#4224=FACE_OUTER_BOUND ( 'NONE', #13593, .T. ) ;
#4229=CARTESIAN_POINT ( 'NONE',  ( 41.82499999726881157, 168.2552932293087906, 9.630534252274372875 ) ) ;
#4231=CARTESIAN_POINT ( 'NONE',  ( 34.42499999726880588, 141.7447067706911810, 9.630534252274376428 ) ) ;
#4237=CARTESIAN_POINT ( 'NONE',  ( 76.18867513459481700, 140.7341522555726669, 4.635254915624211769 ) ) ;
#4241=CARTESIAN_POINT ( 'NONE',  ( 69.49999999453763166, 139.7537977485451393, -4.138211985947621020E-15 ) ) ;
#4246=CARTESIAN_POINT ( 'NONE',  ( 45.61132485994281183, 150.1262045565064795, -15.00000000000007638 ) ) ;
#4255=CARTESIAN_POINT ( 'NONE',  ( 64.71132485994279193, 155.0000000000000000, 15.00000000000001243 ) ) ;
#4261=CARTESIAN_POINT ( 'NONE',  ( 58.47499999726881725, 149.9369285172503510, 15.58253174999999580 ) ) ;
#4266=DIRECTION ( 'NONE',  ( 1.000000000000000000, 0.000000000000000000, 0.000000000000000000 ) ) ;
#4269=CARTESIAN_POINT ( 'NONE',  ( 64.47499999726881015, 149.9369285172503510, 15.58253174999999580 ) ) ;
#4274=CARTESIAN_POINT ( 'NONE',  ( 79.90000000000000568, 141.2096805137202580, 4.480746418436733158 ) ) ;
#4279=VECTOR ( 'NONE', #30085, 1000.000000000000000 ) ;
#4281=CARTESIAN_POINT ( 'NONE',  ( 46.67499999726880588, 141.7447067706911810, 9.630534252274376428 ) ) ;
#4284=CARTESIAN_POINT ( 'NONE',  ( 82.42499999726882720, 141.7447067706911810, 9.630534252274376428 ) ) ;
#4288=CARTESIAN_POINT ( 'NONE',  ( 45.89999999453762314, 150.2886644046228639, -14.50000000000000888 ) ) ;
#4299=ADVANCED_FACE ( 'NONE', ( #11280 ), #11613, .F. ) ;
#4301=EDGE_LOOP ( 'NONE', ( #17124, #24743 ) ) ;
#4305=CYLINDRICAL_SURFACE ( 'NONE', #18679, 15.00000000000001776 ) ;
#4307=CARTESIAN_POINT ( 'NONE',  ( 39.07499999726881157, 141.7447067706911810, -9.630534252274387086 ) ) ;
#4308=ORIENTED_EDGE ( 'NONE', *, *, #25161, .T. ) ;
#4309=CARTESIAN_POINT ( 'NONE',  ( 47.22499999726881015, 160.0630714827496206, -15.58253175000000823 ) ) ;
#4314=CARTESIAN_POINT ( 'NONE',  ( 38.37499999726880873, 155.0000000000000000, 15.58253174999999402 ) ) ;
#4318=CARTESIAN_POINT ( 'NONE',  ( 59.19999999999999574, 167.3344367211045096, 8.961492836873468093 ) ) ;
#4319=CARTESIAN_POINT ( 'NONE',  ( 64.31132485994281467, 169.2658477444273331, 4.635254915624208216 ) ) ;
#4325=CARTESIAN_POINT ( 'NONE',  ( 64.92499999726881299, 145.8408176439707802, -12.60653300113719588 ) ) ;
#4329=CARTESIAN_POINT ( 'NONE',  ( 82.37499999726881583, 155.0000000000000000, 15.58253174999999402 ) ) ;
#4333=DIRECTION ( 'NONE',  ( 0.000000000000000000, 0.000000000000000000, -1.000000000000000000 ) ) ;
#4344=ORIENTED_EDGE ( 'NONE', *, *, #11903, .T. ) ;
#4348=CARTESIAN_POINT ( 'NONE',  ( 82.42499999726882720, 141.7447067706911810, 9.630534252274376428 ) ) ;
#4351=CARTESIAN_POINT ( 'NONE',  ( 73.62499999726883004, 171.3844434931184253, -7.942151717890132712E-15 ) ) ;
#4356=CARTESIAN_POINT ( 'NONE',  ( 41.09999999999999432, 168.7903194862797420, 4.480746418436729606 ) ) ;
#4358=ADVANCED_FACE ( 'NONE', ( #14166 ), #26943, .T. ) ;
#4360=CARTESIAN_POINT ( 'NONE',  ( 125.5000000000000000, 228.4330392262239116, 76.47359838532422316 ) ) ;
#4363=CARTESIAN_POINT ( 'NONE',  ( 50.72499999726881725, 140.1801316387863778, -4.815267126137194431 ) ) ;
#4364=CARTESIAN_POINT ( 'NONE',  ( 61.47499999726879594, 160.0630714827496206, -15.58253175000000823 ) ) ;
#4366=DIRECTION ( 'NONE',  ( 1.000000000000000000, 0.000000000000000000, 0.000000000000000000 ) ) ;
#4367=ADVANCED_FACE ( 'NONE', ( #13830 ), #14233, .F. ) ;
#4374=CARTESIAN_POINT ( 'NONE',  ( 74.48867513459482836, 142.2402378747194405, -9.270509831248439525 ) ) ;
#4381=CARTESIAN_POINT ( 'NONE',  ( 72.77499999726882152, 140.1801316387863778, 4.815267126137185549 ) ) ;
#4384=CARTESIAN_POINT ( 'NONE',  ( 83.07499999726880446, 141.7447067706911810, -9.630534252274387086 ) ) ;
#4387=CARTESIAN_POINT ( 'NONE',  ( 54.82499999726879736, 141.7447067706911810, -9.630534252274385310 ) ) ;
#4388=DIRECTION ( 'NONE',  ( 0.000000000000000000, 1.000000000000000000, -6.454785026890489601E-15 ) ) ;
#4389=ADVANCED_FACE ( 'NONE', ( #21497 ), #8551, .T. ) ;
#4403=CARTESIAN_POINT ( 'NONE',  ( 46.92499999726881299, 145.8408176439707802, -12.60653300113719588 ) ) ;
#4415=CARTESIAN_POINT ( 'NONE',  ( 75.79999999453762882, 146.4771138417591203, -11.73074641843674470 ) ) ;
#4420=FACE_OUTER_BOUND ( 'NONE', #15159, .T. ) ;
#4421=ORIENTED_EDGE ( 'NONE', *, *, #14399, .F. ) ;
#4428=CARTESIAN_POINT ( 'NONE',  ( 85.01132485994281751, 142.2402378747194405, 9.270509831248432420 ) ) ;
#4430=CARTESIAN_POINT ( 'NONE',  ( 57.27499999726882152, 149.9369285172503510, -15.58253175000000823 ) ) ;
#4437=CARTESIAN_POINT ( 'NONE',  ( 66.27499999726880731, 160.0630714827496206, 15.58253174999999402 ) ) ;
#4439=CARTESIAN_POINT ( 'NONE',  ( 32.50000000000000000, 155.0000000000000000, -6.938893903907228378E-15 ) ) ;
#4443=CARTESIAN_POINT ( 'NONE',  ( 80.50000000000000000, 155.0000000000000000, -14.50000000000000711 ) ) ;
#4447=CARTESIAN_POINT ( 'NONE',  ( 82.78867513459482552, 155.0000000000000000, -15.00000000000002487 ) ) ;
#4448=CARTESIAN_POINT ( 'NONE',  ( 51.77499999726881441, 169.8198683612136222, -4.815267126137197984 ) ) ;
#4450=CARTESIAN_POINT ( 'NONE',  ( 84.02499999726882152, 160.0630714827496206, 15.58253174999999402 ) ) ;
#4453=CARTESIAN_POINT ( 'NONE',  ( 52.29999999453762882, 167.3344367211045096, -8.961492836873482304 ) ) ;
#4468=VECTOR ( 'NONE', #5652, 1000.000000000000000 ) ;
#4472=CARTESIAN_POINT ( 'NONE',  ( 34.47499999726881015, 149.9369285172503510, 15.58253174999999580 ) ) ;
#4474=CARTESIAN_POINT ( 'NONE',  ( 46.92499999726881299, 145.8408176439707802, -12.60653300113719588 ) ) ;
#4475=CARTESIAN_POINT ( 'NONE',  ( 32.50000000000000000, 155.0000000000000000, -15.00000000000002487 ) ) ;
#4478=CARTESIAN_POINT ( 'NONE',  ( 50.07499999726881157, 168.2552932293087906, 9.630534252274372875 ) ) ;
#4483=CARTESIAN_POINT ( 'NONE',  ( 58.70000000000000284, 163.5228861582408797, -11.73074641843674470 ) ) ;
#4491=CARTESIAN_POINT ( 'NONE',  ( 61.72499999726881015, 169.8198683612136222, 4.815267126137181997 ) ) ;
#4496=CARTESIAN_POINT ( 'NONE',  ( 81.37499999726881583, 155.0000000000000000, -15.58253175000000823 ) ) ;
#4498=VECTOR ( 'NONE', #22056, 1000.000000000000000 ) ;
#4504=DIRECTION ( 'NONE',  ( 1.000000000000000000, 0.000000000000000000, 0.000000000000000000 ) ) ;
#4513=VERTEX_POINT ( 'NONE', #26768 ) ;
#4520=CARTESIAN_POINT ( 'NONE',  ( 72.97499999726881015, 140.1801316387863778, -4.815267126137194431 ) ) ;
#4521=CARTESIAN_POINT ( 'NONE',  ( 80.22499999726881015, 149.9369285172503510, 15.58253174999999580 ) ) ;
#4524=CARTESIAN_POINT ( 'NONE',  ( 75.68867513459480278, 159.8737954434933499, 15.00000000000019895 ) ) ;
#4526=CARTESIAN_POINT ( 'NONE',  ( 43.89999999999999858, 141.2096805137202580, 4.480746418436733158 ) ) ;
#4532=CARTESIAN_POINT ( 'NONE',  ( 55.92499999726881299, 164.1591823560292198, 12.60653300113718167 ) ) ;
#4533=CARTESIAN_POINT ( 'NONE',  ( 62.37499999726880873, 155.0000000000000000, 15.58253174999999402 ) ) ;
#4546=CARTESIAN_POINT ( 'NONE',  ( 67.91132485994280898, 163.8167787843871110, -12.13525491562423397 ) ) ;
#4555=CARTESIAN_POINT ( 'NONE',  ( 75.37499999726881583, 155.0000000000000000, -15.58253175000000823 ) ) ;
#4559=CARTESIAN_POINT ( 'NONE',  ( 72.52499999726882152, 140.1801316387863778, 4.815267126137185549 ) ) ;
#4563=CARTESIAN_POINT ( 'NONE',  ( 54.92499999726881299, 145.8408176439707802, -12.60653300113719588 ) ) ;
#4564=FACE_OUTER_BOUND ( 'NONE', #32871, .T. ) ;
#4590=CARTESIAN_POINT ( 'NONE',  ( 73.99999999453763166, 155.0000000000000000, -14.50000000000000711 ) ) ;
#4596=EDGE_CURVE ( 'NONE', #14298, #4983, #22508, .T. ) ;
#4597=CARTESIAN_POINT ( 'NONE',  ( 75.31132485994281467, 140.7341522555726669, -4.635254915624220651 ) ) ;
#4600=ORIENTED_EDGE ( 'NONE', *, *, #3552, .T. ) ;
#4610=CARTESIAN_POINT ( 'NONE',  ( 55.37499999726881583, 155.0000000000000000, -15.58253175000000823 ) ) ;
#4611=ORIENTED_EDGE ( 'NONE', *, *, #9801, .T. ) ;
#4617=CARTESIAN_POINT ( 'NONE',  ( 63.47499999726881725, 160.0630714827496206, -15.58253175000000823 ) ) ;
#4622=CARTESIAN_POINT ( 'NONE',  ( 86.29999999999999716, 146.4771138417591203, -11.73074641843674470 ) ) ;
#4623=LINE ( 'NONE', #12281, #19794 ) ;
#4627=CARTESIAN_POINT ( 'NONE',  ( 52.87499999726880162, 138.6155565068815463, -3.929120461958505118E-15 ) ) ;
#4629=CARTESIAN_POINT ( 'NONE',  ( 84.32499999726880446, 145.8408176439707802, 12.60653300113718345 ) ) ;
#4630=CARTESIAN_POINT ( 'NONE',  ( 42.61132485994281893, 159.8737954434936341, 14.99999999999998934 ) ) ;
#4632=CARTESIAN_POINT ( 'NONE',  ( 52.19999999453762740, 163.5228861582408797, -11.73074641843674470 ) ) ;
#4648=CARTESIAN_POINT ( 'NONE',  ( 39.47499999726881015, 160.0630714827496206, -15.58253175000000823 ) ) ;
#4650=CARTESIAN_POINT ( 'NONE',  ( 46.32499999726881157, 145.8408176439707802, 12.60653300113718345 ) ) ;
#4654=CARTESIAN_POINT ( 'NONE',  ( 44.37499999726881583, 155.0000000000000000, 15.58253174999999402 ) ) ;
#4655=CARTESIAN_POINT ( 'NONE',  ( 79.31132485994280046, 140.7341522555726669, -4.635254915624220651 ) ) ;
#4659=CARTESIAN_POINT ( 'NONE',  ( 62.19999999999999574, 142.6655632788954620, -8.961492836873480528 ) ) ;
#4666=CARTESIAN_POINT ( 'NONE',  ( 62.32499999726881867, 145.8408176439707802, 12.60653300113718345 ) ) ;
#4668=ORIENTED_EDGE ( 'NONE', *, *, #26852, .F. ) ;
#4670=CARTESIAN_POINT ( 'NONE',  ( 87.67499999726882720, 168.2552932293087906, -9.630534252274385310 ) ) ;
#4672=CARTESIAN_POINT ( 'NONE',  ( 72.38867513459481984, 140.7341522555726669, -4.635254915624220651 ) ) ;
#4682=CARTESIAN_POINT ( 'NONE',  ( 69.71132485994280614, 155.0000000000000000, -15.00000000000002487 ) ) ;
#4684=VERTEX_POINT ( 'NONE', #24894 ) ;
#4686=CARTESIAN_POINT ( 'NONE',  ( 34.71132485994281325, 155.0000000000000000, 15.00000000000001243 ) ) ;
#4687=ORIENTED_EDGE ( 'NONE', *, *, #19753, .F. ) ;
#4689=CARTESIAN_POINT ( 'NONE',  ( 83.22499999726879594, 160.0630714827496206, -15.58253175000000823 ) ) ;
#4692=CARTESIAN_POINT ( 'NONE',  ( 41.70000000000000284, 146.4771138417591203, 11.73074641843673227 ) ) ;
#4696=DIRECTION ( 'NONE',  ( 0.000000000000000000, -0.7071067811865442421, 0.7071067811865506814 ) ) ;
#4698=CARTESIAN_POINT ( 'NONE',  ( 56.32499999726881157, 145.8408176439707802, 12.60653300113718345 ) ) ;
#4699=CARTESIAN_POINT ( 'NONE',  ( 70.77499999726880731, 140.1801316387863778, 4.815267126137185549 ) ) ;
#4701=FACE_OUTER_BOUND ( 'NONE', #15033, .T. ) ;
#4709=CARTESIAN_POINT ( 'NONE',  ( 74.28867513459483973, 139.2280666364260071, -4.041636747397287284E-15 ) ) ;
#4716=CARTESIAN_POINT ( 'NONE',  ( 76.97499999726881015, 140.1801316387863778, -4.815267126137194431 ) ) ;
#4721=CARTESIAN_POINT ( 'NONE',  ( 69.02499999726880731, 149.9369285172503510, -15.58253175000000823 ) ) ;
#4725=CARTESIAN_POINT ( 'NONE',  ( 65.42499999726881299, 168.2552932293087906, -9.630534252274385310 ) ) ;
#4726=DIRECTION ( 'NONE',  ( 0.000000000000000000, 0.000000000000000000, -1.000000000000000000 ) ) ;
#4740=CARTESIAN_POINT ( 'NONE',  ( 38.92499999726881299, 145.8408176439707802, -12.60653300113719588 ) ) ;
#4749=CARTESIAN_POINT ( 'NONE',  ( 34.98867513459482126, 163.8167787843871110, -12.13525491562423397 ) ) ;
#4752=CARTESIAN_POINT ( 'NONE',  ( 72.69999999453763451, 167.3344367211045096, 8.961492836873468093 ) ) ;
#4769=CARTESIAN_POINT ( 'NONE',  ( 55.57499999726881157, 164.1591823560292198, -12.60653300113719766 ) ) ;
#4775=CARTESIAN_POINT ( 'NONE',  ( 67.87499999726881583, 171.3844434931184253, -7.942151717890132712E-15 ) ) ;
#4783=CARTESIAN_POINT ( 'NONE',  ( 33.52499999726880731, 169.8198683612136222, -4.815267126137197984 ) ) ;
#4785=CARTESIAN_POINT ( 'NONE',  ( 32.50000000000000000, 155.0000000000000000, -6.938893903907228378E-15 ) ) ;
#4788=CARTESIAN_POINT ( 'NONE',  ( 54.07499999726880446, 168.2552932293087906, 9.630534252274372875 ) ) ;
#4791=CARTESIAN_POINT ( 'NONE',  ( 88.02499999726880731, 160.0630714827496206, 15.58253174999999402 ) ) ;
#4792=CARTESIAN_POINT ( 'NONE',  ( 42.01132485994281751, 167.7597621252805880, -9.270509831248443078 ) ) ;
#4793=CARTESIAN_POINT ( 'NONE',  ( 32.50000000000000000, 155.0000000000000000, -6.938893903907228378E-15 ) ) ;
#4794=CARTESIAN_POINT ( 'NONE',  ( 56.59999999453763309, 168.7903194862797420, 4.480746418436729606 ) ) ;
#4801=CARTESIAN_POINT ( 'NONE',  ( 32.50000000000000000, 155.0000000000000000, 15.00000000000001243 ) ) ;
#4808=DIRECTION ( 'NONE',  ( -1.000000000000000000, -0.000000000000000000, -0.000000000000000000 ) ) ;
#4809=ORIENTED_EDGE ( 'NONE', *, *, #27849, .T. ) ;
#4812=CARTESIAN_POINT ( 'NONE',  ( 35.07499999726881157, 141.7447067706911810, -9.630534252274387086 ) ) ;
#4814=CARTESIAN_POINT ( 'NONE',  ( 43.02499999726880020, 149.9369285172503510, -15.58253175000000823 ) ) ;
#4817=CIRCLE ( 'NONE', #12432, 2.149999999999994138 ) ;
#4819=CARTESIAN_POINT ( 'NONE',  ( 50.17499999726881299, 164.1591823560292198, 12.60653300113718167 ) ) ;
#4826=CARTESIAN_POINT ( 'NONE',  ( 69.79999999999996874, 142.6655632788954620, 8.961492836873471646 ) ) ;
#4831=CARTESIAN_POINT ( 'NONE',  ( 34.07499999726879736, 168.2552932293087906, 9.630534252274372875 ) ) ;
#4834=CIRCLE ( 'NONE', #28789, 100.0000000000000284 ) ;
#4835=CARTESIAN_POINT ( 'NONE',  ( 71.82499999726883289, 168.2552932293087906, 9.630534252274372875 ) ) ;
#4837=ORIENTED_EDGE ( 'NONE', *, *, #10381, .T. ) ;
#4839=CARTESIAN_POINT ( 'NONE',  ( 37.09999999453763309, 150.2886644046228639, 14.49999999999999645 ) ) ;
#4849=CIRCLE ( 'NONE', #9202, 112.0000000000000711 ) ;
#4861=CARTESIAN_POINT ( 'NONE',  ( 81.12499999726881583, 155.0000000000000000, -15.58253175000000823 ) ) ;
#4865=CARTESIAN_POINT ( 'NONE',  ( 45.50000000000000000, 155.0000000000000000, 14.49999999999999467 ) ) ;
#4868=CARTESIAN_POINT ( 'NONE',  ( 67.28867513459482552, 170.7719333635740497, -7.904646289410545231E-15 ) ) ;
#4872=CARTESIAN_POINT ( 'NONE',  ( 57.12499999726880873, 155.0000000000000000, -15.58253175000000823 ) ) ;
#4873=CARTESIAN_POINT ( 'NONE',  ( 70.47499999726881015, 149.9369285172503510, 15.58253174999999580 ) ) ;
#4882=( BOUNDED_CURVE ( )  B_SPLINE_CURVE ( 2, ( #13053, #27748, #28086, #33204, #20085, #2994, #9867, #14797, #13373, #20250, #23770 ),
 .UNSPECIFIED., .F., .T. ) 
 B_SPLINE_CURVE_WITH_KNOTS ( ( 3, 2, 2, 2, 2, 3 ),
 ( 0.5892857142857139685, 0.5928571428571425272, 0.5964285714285710860, 0.5999999999999997558, 0.6035714285714283145, 0.6071428571428568732 ),
 .UNSPECIFIED. ) 
 CURVE ( )  GEOMETRIC_REPRESENTATION_ITEM ( )  RATIONAL_B_SPLINE_CURVE ( ( 1.000000000000003109, 0.9510565162951504226, 1.000000000000000000, 0.9510565162951534202, 1.000000000000000000, 0.9510565162951534202, 1.000000000000000000, 0.9510565162951534202, 1.000000000000000000, 0.9510565162951564178, 0.9999999999999970024 ) ) 
 REPRESENTATION_ITEM ( '' )  );
#4892=CARTESIAN_POINT ( 'NONE',  ( 81.07499999726880446, 141.7447067706911810, -9.630534252274385310 ) ) ;
#4896=CARTESIAN_POINT ( 'NONE',  ( 68.62499999726880162, 138.6155565068815747, -3.929120461958505118E-15 ) ) ;
#4899=CARTESIAN_POINT ( 'NONE',  ( 62.32499999726881867, 145.8408176439707802, 12.60653300113718345 ) ) ;
#4913=CARTESIAN_POINT ( 'NONE',  ( 46.18867513459481700, 140.7341522555726669, 4.635254915624211769 ) ) ;
#4915=CARTESIAN_POINT ( 'NONE',  ( 40.52499999726881441, 140.1801316387863778, 4.815267126137185549 ) ) ;
#4917=CYLINDRICAL_SURFACE ( 'NONE', #21679, 15.00000000000001776 ) ;
#4919=ADVANCED_FACE ( 'NONE', ( #10585 ), #17911, .T. ) ;
#4924=CARTESIAN_POINT ( 'NONE',  ( 74.29999999453762882, 167.3344367211045096, -8.961492836873482304 ) ) ;
#4925=ORIENTED_EDGE ( 'NONE', *, *, #8272, .F. ) ;
#4933=AXIS2_PLACEMENT_3D ( 'NONE', #12401, #27556, #32669 ) ;
#4942=CARTESIAN_POINT ( 'NONE',  ( 53.67499999726880588, 168.2552932293087906, -9.630534252274387086 ) ) ;
#4943=ORIENTED_EDGE ( 'NONE', *, *, #20444, .F. ) ;
#4949=CARTESIAN_POINT ( 'NONE',  ( 67.97499999726881015, 169.8198683612136222, 4.815267126137181997 ) ) ;
#4951=CARTESIAN_POINT ( 'NONE',  ( 86.71132485994282035, 155.0000000000000000, 15.00000000000001243 ) ) ;
#4957=CARTESIAN_POINT ( 'NONE',  ( 86.70000000000000284, 163.5228861582408797, -11.73074641843674470 ) ) ;
#4962=CARTESIAN_POINT ( 'NONE',  ( 48.87499999726880873, 138.6155565068815463, -3.929120461958505118E-15 ) ) ;
#4965=CARTESIAN_POINT ( 'NONE',  ( 87.42499999726881299, 168.2552932293087906, -9.630534252274385310 ) ) ;
#4966=CARTESIAN_POINT ( 'NONE',  ( 42.11132485994280472, 169.2658477444273331, -4.635254915624224203 ) ) ;
#4967=CARTESIAN_POINT ( 'NONE',  ( 125.5000000000000000, 231.4735983853249763, -73.43303922622312996 ) ) ;
#4968=CARTESIAN_POINT ( 'NONE',  ( 54.89999999453763024, 159.7113355953771077, 14.49999999999999289 ) ) ;
#4981=CARTESIAN_POINT ( 'NONE',  ( 80.38867513459483405, 140.7341522555726669, -4.635254915624220651 ) ) ;
#4983=VERTEX_POINT ( 'NONE', #17735 ) ;
#4987=CARTESIAN_POINT ( 'NONE',  ( 40.27499999726881441, 160.0630714827496206, 15.58253174999999224 ) ) ;
#4989=CARTESIAN_POINT ( 'NONE',  ( 44.62499999726880873, 138.6155565068815463, -3.929120461958505118E-15 ) ) ;
#4990=FACE_OUTER_BOUND ( 'NONE', #28545, .T. ) ;
#4993=CARTESIAN_POINT ( 'NONE',  ( 47.77499999726881441, 169.8198683612136222, -4.815267126137197984 ) ) ;
#4996=CARTESIAN_POINT ( 'NONE',  ( 125.5000000000000000, 80.04668119422662187, 74.95331880577468553 ) ) ;
#4997=CARTESIAN_POINT ( 'NONE',  ( 65.79999999999998295, 142.6655632788954620, 8.961492836873471646 ) ) ;
#5001=CARTESIAN_POINT ( 'NONE',  ( 86.68867513459481700, 150.1262045565063374, -14.99999999999995737 ) ) ;
#5002=CARTESIAN_POINT ( 'NONE',  ( 33.57499999726881157, 164.1591823560292198, -12.60653300113719766 ) ) ;
#5004=CARTESIAN_POINT ( 'NONE',  ( 73.52499999726882152, 169.8198683612136222, -4.815267126137197984 ) ) ;
#5007=CARTESIAN_POINT ( 'NONE',  ( 87.57499999726880446, 164.1591823560292198, -12.60653300113719766 ) ) ;
#5012=VECTOR ( 'NONE', #22251, 1000.000000000000000 ) ;
#5021=VERTEX_POINT ( 'NONE', #33411 ) ;
#5025=EDGE_CURVE ( 'NONE', #17895, #7373, #342, .T. ) ;
#5030=CARTESIAN_POINT ( 'NONE',  ( 85.42499999726879878, 168.2552932293087906, -9.630534252274385310 ) ) ;
#5035=CARTESIAN_POINT ( 'NONE',  ( 49.19999999999999574, 167.3344367211045096, 8.961492836873468093 ) ) ;
#5038=AXIS2_PLACEMENT_3D ( 'NONE', #18468, #28854, #5510 ) ;
#5039=CARTESIAN_POINT ( 'NONE',  ( 53.42499999726879878, 168.2552932293087906, -9.630534252274385310 ) ) ;
#5040=CARTESIAN_POINT ( 'NONE',  ( 125.5000000000000000, 81.56696077377769427, 76.47359838532574372 ) ) ;
#5042=CARTESIAN_POINT ( 'NONE',  ( 58.12499999726881583, 155.0000000000000000, 15.58253174999999402 ) ) ;
#5043=CARTESIAN_POINT ( 'NONE',  ( 70.27499999726880731, 160.0630714827496206, 15.58253174999999402 ) ) ;
#5045=CARTESIAN_POINT ( 'NONE',  ( 46.31132485994280756, 169.2658477444273331, 4.635254915624208216 ) ) ;
#5049=PRODUCT_DEFINITION_FORMATION_WITH_SPECIFIED_SOURCE ( 'ANY', '', #32253, .NOT_KNOWN. ) ;
#5061=CARTESIAN_POINT ( 'NONE',  ( 76.67499999726881299, 141.7447067706911810, 9.630534252274376428 ) ) ;
#5064=CARTESIAN_POINT ( 'NONE',  ( 74.22499999726881015, 149.9369285172503510, 15.58253174999999580 ) ) ;
#5066=CARTESIAN_POINT ( 'NONE',  ( 60.71132485994280614, 155.0000000000000000, 15.00000000000001243 ) ) ;
#5067=CARTESIAN_POINT ( 'NONE',  ( 61.12499999726880873, 155.0000000000000000, -15.58253175000000823 ) ) ;
#5082=CARTESIAN_POINT ( 'NONE',  ( 35.72499999726881015, 169.8198683612136222, 4.815267126137181997 ) ) ;
#5092=CARTESIAN_POINT ( 'NONE',  ( 74.59999999453762598, 168.7903194862797420, 4.480746418436729606 ) ) ;
#5096=CARTESIAN_POINT ( 'NONE',  ( 75.11132485994279762, 140.7341522555726669, 4.635254915624211769 ) ) ;
#5110=ADVANCED_FACE ( 'NONE', ( #23519 ), #28124, .T. ) ;
#5112=CARTESIAN_POINT ( 'NONE',  ( 64.37499999726881583, 155.0000000000000000, 15.58253174999999402 ) ) ;
#5118=CARTESIAN_POINT ( 'NONE',  ( 87.01132485994283172, 142.2402378747194405, 9.270509831248432420 ) ) ;
#5124=CARTESIAN_POINT ( 'NONE',  ( 87.40000000000000568, 159.7113355953771077, 14.49999999999999289 ) ) ;
#5129=CARTESIAN_POINT ( 'NONE',  ( 53.57499999726881157, 164.1591823560292198, -12.60653300113719766 ) ) ;
#5131=CARTESIAN_POINT ( 'NONE',  ( 127.5000000000000000, 157.1500000000010573, 105.9999999999999858 ) ) ;
#5135=CARTESIAN_POINT ( 'NONE',  ( 55.69999999453762030, 142.6655632788954620, -8.961492836873480528 ) ) ;
#5138=CARTESIAN_POINT ( 'NONE',  ( 47.41132485994281609, 142.2402378747194405, -9.270509831248439525 ) ) ;
#5151=CARTESIAN_POINT ( 'NONE',  ( 43.57499999726881157, 164.1591823560292198, -12.60653300113719766 ) ) ;
#5153=CARTESIAN_POINT ( 'NONE',  ( 51.62499999726880873, 171.3844434931184253, -7.942151717890132712E-15 ) ) ;
#5157=CARTESIAN_POINT ( 'NONE',  ( 43.97499999726881015, 169.8198683612136222, 4.815267126137181997 ) ) ;
#5158=CARTESIAN_POINT ( 'NONE',  ( 79.61132485994284025, 150.1262045565065364, -15.00000000000012434 ) ) ;
#5160=CARTESIAN_POINT ( 'NONE',  ( 43.78867513459481842, 155.0000000000000000, 15.00000000000001243 ) ) ;
#5162=CARTESIAN_POINT ( 'NONE',  ( 64.60000000000000853, 159.7113355953771077, -14.50000000000000888 ) ) ;
#5169=CARTESIAN_POINT ( 'NONE',  ( 73.02499999726882152, 149.9369285172503510, -15.58253175000000823 ) ) ;
#5171=CARTESIAN_POINT ( 'NONE',  ( 43.71132485994280614, 155.0000000000000000, -15.00000000000002487 ) ) ;
#5172=CARTESIAN_POINT ( 'NONE',  ( 35.69999999453762740, 142.6655632788954620, -8.961492836873480528 ) ) ;
#5174=ADVANCED_FACE ( 'NONE', ( #29457 ), #29126, .F. ) ;
#5188=VERTEX_POINT ( 'NONE', #16505 ) ;
#5191=ORIENTED_EDGE ( 'NONE', *, *, #15157, .T. ) ;
#5192=CARTESIAN_POINT ( 'NONE',  ( 81.31132485994280046, 140.7341522555726669, -4.635254915624220651 ) ) ;
#5193=CARTESIAN_POINT ( 'NONE',  ( 85.12499999726881583, 155.0000000000000000, -15.58253175000000823 ) ) ;
#5198=CARTESIAN_POINT ( 'NONE',  ( 51.19999999999999574, 167.3344367211045096, 8.961492836873468093 ) ) ;
#5203=CARTESIAN_POINT ( 'NONE',  ( 53.72499999726881015, 169.8198683612136222, 4.815267126137181997 ) ) ;
#5206=CARTESIAN_POINT ( 'NONE',  ( 56.72499999726881015, 140.1801316387863778, -4.815267126137194431 ) ) ;
#5207=CARTESIAN_POINT ( 'NONE',  ( 68.97499999726881015, 140.1801316387863778, -4.815267126137194431 ) ) ;
#5209=CARTESIAN_POINT ( 'NONE',  ( 46.21132485994280614, 170.7719333635740497, -7.904646289410545231E-15 ) ) ;
#5223=VERTEX_POINT ( 'NONE', #29294 ) ;
#5227=( BOUNDED_CURVE ( )  B_SPLINE_CURVE ( 2, ( #13125, #186, #10584, #17910, #11406, #18898, #1011, #3061, #3390, #21617, #21458 ),
 .UNSPECIFIED., .F., .T. ) 
 B_SPLINE_CURVE_WITH_KNOTS ( ( 3, 2, 2, 2, 2, 3 ),
 ( 0.1071428571428569843, 0.1107142857142855291, 0.1142857142857140879, 0.1178571428571426327, 0.1214285714285711915, 0.1249999999999998473 ),
 .UNSPECIFIED. ) 
 CURVE ( )  GEOMETRIC_REPRESENTATION_ITEM ( )  RATIONAL_B_SPLINE_CURVE ( ( 1.000000000000001554, 0.9510565162951518658, 1.000000000000000000, 0.9510565162951534202, 1.000000000000000000, 0.9510565162951534202, 1.000000000000000000, 0.9510565162951534202, 1.000000000000000000, 0.9510565162951555296, 0.9999999999999978906 ) ) 
 REPRESENTATION_ITEM ( '' )  );
#5228=CARTESIAN_POINT ( 'NONE',  ( 69.92499999726881299, 164.1591823560292198, 12.60653300113718167 ) ) ;
#5231=CARTESIAN_POINT ( 'NONE',  ( 60.72499999726881015, 140.1801316387863778, -4.815267126137194431 ) ) ;
#5247=CARTESIAN_POINT ( 'NONE',  ( 37.02499999726880731, 149.9369285172503510, -15.58253175000000823 ) ) ;
#5249=CARTESIAN_POINT ( 'NONE',  ( 32.50000000000000000, 155.0000000000000000, -6.938893903907228378E-15 ) ) ;
#5255=CARTESIAN_POINT ( 'NONE',  ( 79.19999999453763451, 146.4771138417591203, 11.73074641843673227 ) ) ;
#5260=CARTESIAN_POINT ( 'NONE',  ( 75.51132485994280330, 146.1832212156128890, -12.13525491562423042 ) ) ;
#5265=VECTOR ( 'NONE', #1502, 1000.000000000000000 ) ;
#5270=CARTESIAN_POINT ( 'NONE',  ( 82.71132485994282035, 155.0000000000000000, 15.00000000000001243 ) ) ;
#5272=CARTESIAN_POINT ( 'NONE',  ( 60.37499999726880873, 155.0000000000000000, 15.58253174999999402 ) ) ;
#5275=CARTESIAN_POINT ( 'NONE',  ( 32.50000000000000000, 155.0000000000000000, -6.938893903907228378E-15 ) ) ;
#5277=VECTOR ( 'NONE', #17549, 1000.000000000000000 ) ;
#5286=CARTESIAN_POINT ( 'NONE',  ( 34.22499999726881015, 149.9369285172503510, 15.58253174999999580 ) ) ;
#5291=CARTESIAN_POINT ( 'NONE',  ( 57.87499999726880873, 171.3844434931184253, -7.942151717890132712E-15 ) ) ;
#5297=CARTESIAN_POINT ( 'NONE',  ( 59.19999999453762740, 146.4771138417591203, 11.73074641843673227 ) ) ;
#5300=CARTESIAN_POINT ( 'NONE',  ( 125.5000000000000000, 48.99999999999998579, -1.387778780781445676E-14 ) ) ;
#5301=ADVANCED_FACE ( 'NONE', ( #21785 ), #21288, .T. ) ;
#5312=CARTESIAN_POINT ( 'NONE',  ( 79.88867513459481984, 150.1262045565063374, 14.99999999999994316 ) ) ;
#5316=CARTESIAN_POINT ( 'NONE',  ( 42.77499999726880731, 140.1801316387863778, 4.815267126137185549 ) ) ;
#5317=ORIENTED_EDGE ( 'NONE', *, *, #20997, .F. ) ;
#5318=CARTESIAN_POINT ( 'NONE',  ( 52.82499999726880446, 141.7447067706911810, -9.630534252274385310 ) ) ;
#5322=CARTESIAN_POINT ( 'NONE',  ( 53.37499999726881583, 155.0000000000000000, -15.58253175000000823 ) ) ;
#5325=CARTESIAN_POINT ( 'NONE',  ( 44.58867513459481557, 146.1832212156128890, -12.13525491562423042 ) ) ;
#5326=CARTESIAN_POINT ( 'NONE',  ( 65.10000000000000853, 168.7903194862797420, 4.480746418436729606 ) ) ;
#5332=CARTESIAN_POINT ( 'NONE',  ( 37.67499999726881299, 168.2552932293087906, -9.630534252274385310 ) ) ;
#5335=CARTESIAN_POINT ( 'NONE',  ( 69.92499999726881299, 164.1591823560292198, 12.60653300113718167 ) ) ;
#5339=CARTESIAN_POINT ( 'NONE',  ( 34.79999999453762882, 163.5228861582408797, 11.73074641843673049 ) ) ;
#5344=ORIENTED_EDGE ( 'NONE', *, *, #32854, .T. ) ;
#5349=ORIENTED_EDGE ( 'NONE', *, *, #43, .T. ) ;
#5352=CARTESIAN_POINT ( 'NONE',  ( 74.11132485994281183, 169.2658477444273331, -4.635254915624224203 ) ) ;
#5359=CARTESIAN_POINT ( 'NONE',  ( 56.61132485994281893, 159.8737954434936057, 15.00000000000001421 ) ) ;
#5361=CARTESIAN_POINT ( 'NONE',  ( 34.32499999726881157, 145.8408176439707802, 12.60653300113718345 ) ) ;
#5362=CARTESIAN_POINT ( 'NONE',  ( 87.42499999726881299, 168.2552932293087906, -9.630534252274385310 ) ) ;
#5367=CARTESIAN_POINT ( 'NONE',  ( 45.29999999999999716, 163.5228861582408797, 11.73074641843673049 ) ) ;
#5369=CARTESIAN_POINT ( 'NONE',  ( 83.81132485994281467, 159.8737954434936057, -15.00000000000002665 ) ) ;
#5371=CARTESIAN_POINT ( 'NONE',  ( 51.32499999726881157, 164.1591823560292198, -12.60653300113719766 ) ) ;
#5374=CARTESIAN_POINT ( 'NONE',  ( 66.42499999726881299, 141.7447067706911810, 9.630534252274376428 ) ) ;
#5375=CARTESIAN_POINT ( 'NONE',  ( 67.17499999726881299, 145.8408176439707802, -12.60653300113719588 ) ) ;
#5377=FACE_BOUND ( 'NONE', #11293, .T. ) ;
#5380=EDGE_CURVE ( 'NONE', #19088, #22486, #21665, .T. ) ;
#5391=ORIENTED_EDGE ( 'NONE', *, *, #351, .F. ) ;
#5399=CARTESIAN_POINT ( 'NONE',  ( 74.92499999726881299, 145.8408176439707802, -12.60653300113719588 ) ) ;
#5402=AXIS2_PLACEMENT_3D ( 'NONE', #32682, #14294, #8844 ) ;
#5403=CARTESIAN_POINT ( 'NONE',  ( 64.42499999726879878, 141.7447067706911810, 9.630534252274376428 ) ) ;
#5412=FACE_BOUND ( 'NONE', #31743, .T. ) ;
#5418=CARTESIAN_POINT ( 'NONE',  ( 38.72499999726881015, 140.1801316387863778, -4.815267126137194431 ) ) ;
#5425=CARTESIAN_POINT ( 'NONE',  ( 82.19999999453763451, 163.5228861582408797, -11.73074641843674470 ) ) ;
#5427=CIRCLE ( 'NONE', #5402, 13.00000000000001776 ) ;
#5429=( BOUNDED_CURVE ( )  B_SPLINE_CURVE ( 2, ( #22178, #32567, #9238, #19628, #27460, #9403, #7022, #17407, #14845, #22859, #27968 ),
 .UNSPECIFIED., .F., .T. ) 
 B_SPLINE_CURVE_WITH_KNOTS ( ( 3, 2, 2, 2, 2, 3 ),
 ( 0.4821428571428572063, 0.4857142857142857650, 0.4892857142857143238, 0.4928571428571428825, 0.4964285714285714413, 0.5000000000000000000 ),
 .UNSPECIFIED. ) 
 CURVE ( )  GEOMETRIC_REPRESENTATION_ITEM ( )  RATIONAL_B_SPLINE_CURVE ( ( 0.9999999999999992228, 0.9510565162951541973, 1.000000000000000000, 0.9510565162951534202, 1.000000000000000000, 0.9510565162951534202, 1.000000000000000000, 0.9510565162951534202, 1.000000000000000000, 0.9510565162951534202, 1.000000000000000000 ) ) 
 REPRESENTATION_ITEM ( '' )  );
#5432=ORIENTED_EDGE ( 'NONE', *, *, #24927, .T. ) ;
#5435=ORIENTED_EDGE ( 'NONE', *, *, #22701, .F. ) ;
#5438=CARTESIAN_POINT ( 'NONE',  ( 51.08867513459482979, 167.7597621252805880, -9.270509831248443078 ) ) ;
#5439=CYLINDRICAL_SURFACE ( 'NONE', #21978, 15.00000000000001776 ) ;
#5445=CARTESIAN_POINT ( 'NONE',  ( 64.67499999726879878, 141.7447067706911810, 9.630534252274376428 ) ) ;
#5447=CARTESIAN_POINT ( 'NONE',  ( 46.78867513459482552, 155.0000000000000000, -15.00000000000002487 ) ) ;
#5456=CARTESIAN_POINT ( 'NONE',  ( 35.92499999726880588, 164.1591823560292198, 12.60653300113718167 ) ) ;
#5462=CARTESIAN_POINT ( 'NONE',  ( 60.37499999726880873, 155.0000000000000000, 15.58253174999999402 ) ) ;
#5468=CARTESIAN_POINT ( 'NONE',  ( 61.19999999453762740, 146.4771138417591203, 11.73074641843673227 ) ) ;
#5471=CARTESIAN_POINT ( 'NONE',  ( 76.81132485994282888, 150.1262045565065364, 15.00000000000011191 ) ) ;
#5476=VERTEX_POINT ( 'NONE', #12240 ) ;
#5479=ORIENTED_EDGE ( 'NONE', *, *, #29715, .F. ) ;
#5482=CARTESIAN_POINT ( 'NONE',  ( 42.37499999726881583, 155.0000000000000000, 15.58253174999999402 ) ) ;
#5484=CARTESIAN_POINT ( 'NONE',  ( 49.32499999726881157, 164.1591823560292198, -12.60653300113719766 ) ) ;
#5489=CARTESIAN_POINT ( 'NONE',  ( 52.77499999726881441, 140.1801316387863778, 4.815267126137185549 ) ) ;
#5492=CYLINDRICAL_SURFACE ( 'NONE', #21386, 15.00000000000001776 ) ;
#5493=CARTESIAN_POINT ( 'NONE',  ( 66.80000000000001137, 167.3344367211045096, -8.961492836873482304 ) ) ;
#5497=CARTESIAN_POINT ( 'NONE',  ( 57.48867513459482126, 167.7597621252805880, 9.270509831248428867 ) ) ;
#5498=CARTESIAN_POINT ( 'NONE',  ( 39.67499999726881299, 168.2552932293087906, -9.630534252274385310 ) ) ;
#5500=CARTESIAN_POINT ( 'NONE',  ( 71.02499999726882152, 149.9369285172503510, -15.58253175000000823 ) ) ;
#5502=CARTESIAN_POINT ( 'NONE',  ( 48.71132485994280614, 155.0000000000000000, 15.00000000000001243 ) ) ;
#5503=CARTESIAN_POINT ( 'NONE',  ( 42.49999999453763166, 170.2462022514548323, -7.872454543227099337E-15 ) ) ;
#5510=DIRECTION ( 'NONE',  ( 0.000000000000000000, 0.000000000000000000, 1.000000000000000000 ) ) ;
#5515=VERTEX_POINT ( 'NONE', #33014 ) ;
#5521=CARTESIAN_POINT ( 'NONE',  ( 87.62499999726880162, 171.3844434931184253, -7.942151717890132712E-15 ) ) ;
#5524=EDGE_CURVE ( 'NONE', #9319, #5515, #22381, .T. ) ;
#5527=CARTESIAN_POINT ( 'NONE',  ( 48.20000000000000995, 142.6655632788954620, -8.961492836873480528 ) ) ;
#5529=CARTESIAN_POINT ( 'NONE',  ( 84.41132485994282320, 167.7597621252805880, 9.270509831248428867 ) ) ;
#5530=CARTESIAN_POINT ( 'NONE',  ( 50.12499999726881583, 155.0000000000000000, 15.58253174999999402 ) ) ;
#5532=EDGE_LOOP ( 'NONE', ( #26013, #2553, #20507, #13710 ) ) ;
#5535=CARTESIAN_POINT ( 'NONE',  ( 61.12499999726880873, 155.0000000000000000, -15.58253175000000823 ) ) ;
#5536=CARTESIAN_POINT ( 'NONE',  ( 76.27499999726877888, 160.0630714827496206, 15.58253174999999402 ) ) ;
#5538=CARTESIAN_POINT ( 'NONE',  ( 87.50000000000001421, 155.0000000000000000, 70.00000000000000000 ) ) ;
#5540=CARTESIAN_POINT ( 'NONE',  ( 84.78867513459482552, 155.0000000000000000, -15.00000000000002487 ) ) ;
#5541=ORIENTED_EDGE ( 'NONE', *, *, #3976, .F. ) ;
#5545=CARTESIAN_POINT ( 'NONE',  ( 34.48867513459482126, 142.2402378747194405, -9.270509831248439525 ) ) ;
#5548=ORIENTED_EDGE ( 'NONE', *, *, #30401, .T. ) ;
#5555=EDGE_LOOP ( 'NONE', ( #27000, #21510, #4809, #11843 ) ) ;
#5556=CARTESIAN_POINT ( 'NONE',  ( 78.22499999726881015, 149.9369285172503510, 15.58253174999999580 ) ) ;
#5561=CARTESIAN_POINT ( 'NONE',  ( 72.92499999726881299, 145.8408176439707802, -12.60653300113719588 ) ) ;
#5564=EDGE_CURVE ( 'NONE', #8437, #19762, #5963, .T. ) ;
#5567=CARTESIAN_POINT ( 'NONE',  ( 59.78867513459481842, 155.0000000000000000, 15.00000000000001243 ) ) ;
#5578=CARTESIAN_POINT ( 'NONE',  ( 46.32499999726881157, 145.8408176439707802, 12.60653300113718345 ) ) ;
#5585=CARTESIAN_POINT ( 'NONE',  ( 79.09999999453761177, 150.2886644046228639, 14.49999999999999645 ) ) ;
#5586=VECTOR ( 'NONE', #30769, 1000.000000000000000 ) ;
#5598=CARTESIAN_POINT ( 'NONE',  ( 77.97499999726881015, 169.8198683612136222, 4.815267126137181997 ) ) ;
#5601=CARTESIAN_POINT ( 'NONE',  ( 56.68867513459484542, 150.1262045565065364, -15.00000000000012434 ) ) ;
#5604=CARTESIAN_POINT ( 'NONE',  ( 62.17499999726882010, 164.1591823560292198, 12.60653300113718167 ) ) ;
#5606=CARTESIAN_POINT ( 'NONE',  ( 41.68867513459482410, 159.8737954434936057, 15.00000000000001421 ) ) ;
#5613=CARTESIAN_POINT ( 'NONE',  ( 87.50000000000002842, 145.7452232778646817, -11.80462230752951136 ) ) ;
#5615=CARTESIAN_POINT ( 'NONE',  ( 86.67499999726878457, 141.7447067706911810, 9.630534252274376428 ) ) ;
#5617=CARTESIAN_POINT ( 'NONE',  ( 39.62499999726880162, 171.3844434931184253, -7.942151717890132712E-15 ) ) ;
#5618=CARTESIAN_POINT ( 'NONE',  ( 36.58867513459482268, 146.1832212156128890, -12.13525491562423042 ) ) ;
#5619=DIRECTION ( 'NONE',  ( 1.000000000000000000, 0.000000000000000000, 0.000000000000000000 ) ) ;
#5622=CARTESIAN_POINT ( 'NONE',  ( 58.47499999726880304, 149.9369285172503510, 15.58253174999999580 ) ) ;
#5627=CARTESIAN_POINT ( 'NONE',  ( 125.5000000000000000, 80.04668119422662187, 74.95331880577468553 ) ) ;
#5631=CARTESIAN_POINT ( 'NONE',  ( 58.69999999453762740, 167.3344367211045096, 8.961492836873468093 ) ) ;
#5634=ADVANCED_FACE ( 'NONE', ( #33142 ), #22915, .T. ) ;
#5637=DIRECTION ( 'NONE',  ( 0.000000000000000000, 0.000000000000000000, -1.000000000000000000 ) ) ;
#5638=VERTEX_POINT ( 'NONE', #15245 ) ;
#5641=EDGE_CURVE ( 'NONE', #27342, #3282, #12942, .T. ) ;
#5649=CARTESIAN_POINT ( 'NONE',  ( 44.37499999726881583, 155.0000000000000000, 15.58253174999999402 ) ) ;
#5650=VERTEX_POINT ( 'NONE', #15071 ) ;
#5651=CARTESIAN_POINT ( 'NONE',  ( 49.62499999726880873, 171.3844434931184253, -7.942151717890132712E-15 ) ) ;
#5652=DIRECTION ( 'NONE',  ( 1.000000000000000000, 0.000000000000000000, 0.000000000000000000 ) ) ;
#5656=CARTESIAN_POINT ( 'NONE',  ( 51.37499999726881583, 155.0000000000000000, -15.58253175000000823 ) ) ;
#5658=CARTESIAN_POINT ( 'NONE',  ( 44.38867513459482694, 140.7341522555726669, -4.635254915624220651 ) ) ;
#5660=CARTESIAN_POINT ( 'NONE',  ( 76.20000000000000284, 142.6655632788954620, -8.961492836873480528 ) ) ;
#5666=CARTESIAN_POINT ( 'NONE',  ( 38.07499999726880446, 168.2552932293087906, 9.630534252274372875 ) ) ;
#5668=CARTESIAN_POINT ( 'NONE',  ( 75.62499999726881583, 171.3844434931184253, -7.942151717890132712E-15 ) ) ;
#5671=CARTESIAN_POINT ( 'NONE',  ( 40.09999999453762598, 159.7113355953771077, -14.50000000000000888 ) ) ;
#5672=CARTESIAN_POINT ( 'NONE',  ( 40.31132485994280756, 169.2658477444273331, 4.635254915624208216 ) ) ;
#5681=CARTESIAN_POINT ( 'NONE',  ( 125.5000000000000000, 229.9533188057739039, -74.95331880577418815 ) ) ;
#5689=CARTESIAN_POINT ( 'NONE',  ( 35.17499999726881299, 145.8408176439707802, -12.60653300113719588 ) ) ;
#5693=CARTESIAN_POINT ( 'NONE',  ( 57.40000000000000568, 159.7113355953771077, 14.49999999999999289 ) ) ;
#5696=CARTESIAN_POINT ( 'NONE',  ( 48.62499999726880873, 138.6155565068815463, -3.929120461958505118E-15 ) ) ;
#5700=CARTESIAN_POINT ( 'NONE',  ( 63.92499999726880588, 164.1591823560292198, 12.60653300113718167 ) ) ;
#5701=CARTESIAN_POINT ( 'NONE',  ( 78.17499999726881299, 164.1591823560292198, 12.60653300113718167 ) ) ;
#5705=CARTESIAN_POINT ( 'NONE',  ( 84.48867513459482836, 142.2402378747194405, -9.270509831248439525 ) ) ;
#5720=CARTESIAN_POINT ( 'NONE',  ( 76.92499999726881299, 145.8408176439707802, -12.60653300113719588 ) ) ;
#5721=DIRECTION ( 'NONE',  ( 0.000000000000000000, 0.000000000000000000, -1.000000000000000000 ) ) ;
#5723=CARTESIAN_POINT ( 'NONE',  ( 71.32499999726881867, 164.1591823560292198, -12.60653300113719766 ) ) ;
#5728=LINE ( 'NONE', #23795, #8523 ) ;
#5731=CARTESIAN_POINT ( 'NONE',  ( 63.48867513459483547, 167.7597621252805880, 9.270509831248428867 ) ) ;
#5737=CARTESIAN_POINT ( 'NONE',  ( 43.72499999726881015, 169.8198683612136222, 4.815267126137181997 ) ) ;
#5744=CARTESIAN_POINT ( 'NONE',  ( 79.49999999453764588, 139.7537977485451393, -4.138211985947621020E-15 ) ) ;
#5752=VERTEX_POINT ( 'NONE', #30756 ) ;
#5754=CARTESIAN_POINT ( 'NONE',  ( 78.87499999726880162, 138.6155565068815747, -3.929120461958505118E-15 ) ) ;
#5755=CARTESIAN_POINT ( 'NONE',  ( 86.98867513459482836, 163.8167787843871110, -12.13525491562423397 ) ) ;
#5761=CARTESIAN_POINT ( 'NONE',  ( 61.07499999726881157, 141.7447067706911810, -9.630534252274387086 ) ) ;
#5767=CARTESIAN_POINT ( 'NONE',  ( 82.98867513459481415, 163.8167787843871110, -12.13525491562423397 ) ) ;
#5770=CARTESIAN_POINT ( 'NONE',  ( 82.97499999726881015, 140.1801316387863778, -4.815267126137194431 ) ) ;
#5772=CARTESIAN_POINT ( 'NONE',  ( 40.32499999726881157, 145.8408176439707802, 12.60653300113718345 ) ) ;
#5773=CARTESIAN_POINT ( 'NONE',  ( 36.38867513459481984, 140.7341522555726669, -4.635254915624220651 ) ) ;
#5777=CARTESIAN_POINT ( 'NONE',  ( 58.97499999726881015, 140.1801316387863778, -4.815267126137194431 ) ) ;
#5782=CARTESIAN_POINT ( 'NONE',  ( 54.98867513459482126, 163.8167787843871110, -12.13525491562423397 ) ) ;
#5784=CARTESIAN_POINT ( 'NONE',  ( 57.39999999453762314, 141.2096805137202580, 4.480746418436733158 ) ) ;
#5789=CARTESIAN_POINT ( 'NONE',  ( 59.31132485994280756, 140.7341522555726669, -4.635254915624220651 ) ) ;
#5790=AXIS2_PLACEMENT_3D ( 'NONE', #30636, #2184, #12569 ) ;
#5791=EDGE_LOOP ( 'NONE', ( #18595, #33002, #16146, #33387 ) ) ;
#5794=DIRECTION ( 'NONE',  ( -1.000000000000000000, -0.000000000000000000, 0.000000000000000000 ) ) ;
#5796=VERTEX_POINT ( 'NONE', #15747 ) ;
#5803=CARTESIAN_POINT ( 'NONE',  ( 43.67499999726881299, 168.2552932293087906, -9.630534252274387086 ) ) ;
#5805=CARTESIAN_POINT ( 'NONE',  ( 50.72499999726881725, 140.1801316387863778, -4.815267126137194431 ) ) ;
#5811=CARTESIAN_POINT ( 'NONE',  ( 55.27499999726881441, 149.9369285172503510, -15.58253175000000823 ) ) ;
#5813=CARTESIAN_POINT ( 'NONE',  ( 73.58867513459482268, 163.8167787843871110, 12.13525491562421621 ) ) ;
#5817=CARTESIAN_POINT ( 'NONE',  ( 75.09999999999999432, 168.7903194862797420, 4.480746418436729606 ) ) ;
#5818=CARTESIAN_POINT ( 'NONE',  ( 65.48867513459484258, 167.7597621252805880, 9.270509831248428867 ) ) ;
#5819=DIRECTION ( 'NONE',  ( 0.000000000000000000, 0.000000000000000000, 1.000000000000000000 ) ) ;
#5822=CARTESIAN_POINT ( 'NONE',  ( 36.77499999726881441, 140.1801316387863778, 4.815267126137185549 ) ) ;
#5823=EDGE_CURVE ( 'NONE', #7737, #17237, #33073, .T. ) ;
#5825=CARTESIAN_POINT ( 'NONE',  ( 74.52499999726880731, 140.1801316387863778, 4.815267126137185549 ) ) ;
#5828=CARTESIAN_POINT ( 'NONE',  ( 39.69999999453763451, 142.6655632788954620, -8.961492836873480528 ) ) ;
#5834=VECTOR ( 'NONE', #19885, 1000.000000000000000 ) ;
#5842=CARTESIAN_POINT ( 'NONE',  ( 79.28867513459482552, 170.7719333635740497, -7.904646289410545231E-15 ) ) ;
#5845=EDGE_CURVE ( 'NONE', #2840, #25792, #21193, .T. ) ;
#5847=DIRECTION ( 'NONE',  ( 0.000000000000000000, 0.000000000000000000, -1.000000000000000000 ) ) ;
#5851=CARTESIAN_POINT ( 'NONE',  ( 86.22499999726882436, 149.9369285172503510, 15.58253174999999580 ) ) ;
#5855=CARTESIAN_POINT ( 'NONE',  ( 52.39999999999999858, 150.2886644046228639, -14.50000000000000888 ) ) ;
#5859=CARTESIAN_POINT ( 'NONE',  ( 55.72499999726881015, 169.8198683612136222, 4.815267126137181997 ) ) ;
#5863=CARTESIAN_POINT ( 'NONE',  ( 61.82499999726881157, 168.2552932293087906, 9.630534252274372875 ) ) ;
#5864=CARTESIAN_POINT ( 'NONE',  ( 77.67499999726879878, 168.2552932293087906, -9.630534252274385310 ) ) ;
#5874=CARTESIAN_POINT ( 'NONE',  ( 32.50000000000000000, 155.0000000000000000, -15.00000000000002487 ) ) ;
#5885=CARTESIAN_POINT ( 'NONE',  ( 74.72499999726881015, 140.1801316387863778, -4.815267126137194431 ) ) ;
#5889=CARTESIAN_POINT ( 'NONE',  ( 70.32499999726881867, 145.8408176439707802, 12.60653300113718345 ) ) ;
#5894=CARTESIAN_POINT ( 'NONE',  ( 35.70000000000000284, 146.4771138417591203, 11.73074641843673227 ) ) ;
#5900=CARTESIAN_POINT ( 'NONE',  ( 127.5000000000000000, 228.4330392262239116, 76.47359838532422316 ) ) ;
#5904=CARTESIAN_POINT ( 'NONE',  ( 45.72499999726881015, 169.8198683612136222, 4.815267126137181997 ) ) ;
#5906=CARTESIAN_POINT ( 'NONE',  ( 127.5000000000000000, 48.99999999999998579, 2.149999999999971489 ) ) ;
#5912=CARTESIAN_POINT ( 'NONE',  ( 77.69999999453762030, 142.6655632788954620, -8.961492836873480528 ) ) ;
#5917=ORIENTED_EDGE ( 'NONE', *, *, #26515, .F. ) ;
#5921=CIRCLE ( 'NONE', #7584, 2.149999999999984812 ) ;
#5923=CARTESIAN_POINT ( 'NONE',  ( 73.87499999726881583, 171.3844434931184253, -7.942151717890134290E-15 ) ) ;
#5924=CARTESIAN_POINT ( 'NONE',  ( 53.61132485994281183, 150.1262045565062806, -14.99999999999993072 ) ) ;
#5931=CARTESIAN_POINT ( 'NONE',  ( 66.67499999726881299, 141.7447067706911810, 9.630534252274376428 ) ) ;
#5933=CARTESIAN_POINT ( 'NONE',  ( 40.78867513459481842, 155.0000000000000000, -15.00000000000002487 ) ) ;
#5937=CARTESIAN_POINT ( 'NONE',  ( 80.11132485994279762, 169.2658477444273331, -4.635254915624224203 ) ) ;
#5940=CARTESIAN_POINT ( 'NONE',  ( 82.57499999726880446, 145.8408176439707802, 12.60653300113718345 ) ) ;
#5943=CARTESIAN_POINT ( 'NONE',  ( 37.72499999726881015, 169.8198683612136222, 4.815267126137181997 ) ) ;
#5944=CARTESIAN_POINT ( 'NONE',  ( 36.78867513459482552, 155.0000000000000000, -15.00000000000002487 ) ) ;
#5949=CARTESIAN_POINT ( 'NONE',  ( 56.87499999726880162, 138.6155565068815463, -3.929120461958505118E-15 ) ) ;
#5956=CARTESIAN_POINT ( 'NONE',  ( 58.09999999453763309, 159.7113355953771077, -14.50000000000000888 ) ) ;
#5959=FACE_OUTER_BOUND ( 'NONE', #15281, .T. ) ;
#5961=CARTESIAN_POINT ( 'NONE',  ( 72.31132485994281467, 169.2658477444273331, 4.635254915624208216 ) ) ;
#5963=( BOUNDED_CURVE ( )  B_SPLINE_CURVE ( 2, ( #32347, #9514, #27564, #22459, #3891, #14790, #17010, #9011, #19400, #1348, #14286, #11735, #27404, #4231, #14629, #30300, #32851, #17356, #27742, #31148, #26196, #25869, #7985, #31319, #20926, #15302, #5082, #30647, #18369, #20243, #15636, #25527, #28596, #26040, #2710, #22971, #7815, #20422, #12755, #5247, #22807, #28761, #15803, #2196, #33197, #10378, #15478, #2535, #28079, #18032, #33370, #17692, #13088, #2864, #30815, #28427, #5418, #17863, #4740, #12578, #30993, #12918, #7478, #20592, #18205, #10545, #23314, #23477, #9861, #17921, #144, #23146, #28261, #7650, #4915, #7315, #15132, #10044, #25694, #2365, #33534, #10207, #20751, #10873, #3519, #29089, #6242, #23804, #18536, #18700, #6067, #21248, #13249, #31486, #476, #8468, #26520, #26689, #16461, #15971, #23645, #13912, #8309, #31641, #3350, #26859, #5737, #13740, #16630, #24297, #16128, #305, #3192, #965, #10704, #24137, #13581, #8153, #23972, #804, #11194, #21082, #19194, #634, #29591, #32135, #5904, #11033, #21415, #21573, #31802, #28918, #5578, #18856, #27026, #11365, #29252, #26365, #16298, #21745, #3024, #13410, #31965, #8797, #8636, #19029, #29417, #32805, #6920, #14417, #30258, #32307, #32639, #17140, #16965, #20034, #3686, #14245, #30087, #32973, #22082, #27360, #1803, #6752, #22587, #12200, #9639, #29928, #19694, #11528, #30434, #1135, #17311, #6417, #9472, #27701, #4363, #3853, #12027, #1310, #4026, #16800, #7094, #17475, #14079, #27197, #24474, #24984, #27526, #4187, #8969, #9302, #24644, #19359, #14746, #21910, #11699, #14583, #29754, #32468, #9135, #1635, #25139, #22415, #19534, #1470, #19860, #6581, #24810, #11865, #22252, #10160, #18164, #17815, #25481, #25653, #9993, #7941, #14925, #25994, #12538, #22928, #33323, #102, #2492, #17994, #13047, #27860, #4532, #20380, #22764, #33663, #4698, #28558, #2664, #15088, #5206, #20543, #10504, #7434, #4872, #30601, #25313, #28037, #20883, #30772, #28213, #10339, #15261, #2320, #5042, #2155, #23437, #15592, #9820, #12707, #31281, #23103, #1977, #33491, #30945, #28385, #15432, #7610, #25828, #20711, #7266, #12368, #12875, #33157, #23268, #31111, #7773, #20201, #17649, #29211, #28879, #16420, #8596, #270, #5535, #15762, #8431, #8268, #2823, #15925, #18817, #5863, #594, #13538, #18656, #10665, #23932, #11160, #13368, #26323, #761, #13694, #21535, #29046, #31925, #11324, #18992, #2988, #21041, #10990, #29382, #16088, #5700, #23765, #16260, #26482, #26816, #21369, #3480, #13871, #24256, #10832, #31765, #26157, #926, #26646, #21708, #3310, #3151, #24094, #13207, #6028, #18494, #32099, #18323, #31444, #28718, #5374, #23606, #8112, #430, #21207, #31601, #14041, #19150, #3646, #8762, #16590, #24437, #1101, #26982, #6201, #29547, #11494, #21872, #7293, #22787, #13068, #12898, #4896, #33180, #31130, #25334, #4721, #28405, #7795, #30795, #15112, #15282, #22952, #20905, #27885, #5228, #25506, #14947, #33349, #30625, #18185, #10021, #2176, #28578, #20402, #124, #17672, #12393, #33686, #12560, #7116, #2002, #28060, #2345, #7457, #20569, #17839, #28239, #9843, #15614, #25676, #4559, #23458, #12735, #10526, #26019, #33512, #23124, #23293, #2512, #10360, #10186, #20733, #20224, #30972, #7632, #18014, #17496, #5064, #15457, #25851, #2690, #15950, #5885, #947, #5399, #31623, #6051, #29402, #23787, #13564, #15782, #16442, #28739, #24118, #288, #3332, #785, #11178, #31466, #16282, #28900, #21228, #13717, #31301, #5720, #21555, #18838, #7963, #29233, #23953, #11013, #2843, #26504, #8133, #26175, #31948, #11347, #5556, #3173, #13894, #26345, #13230, #10682, #18517, #23625, #3503, #8618, #26671, #19013, #614, #26840, #24275, #21395, #18348, #8290, #3009, #29068, #13388, #21065, #457, #10855, #18680, #16108, #31785, #8452, #32788, #14230, #6904, #1784, #21728, #6398, #16612, #27514, #32292, #22397, #19848, #8953, #12011, #14406, #4348, #1293, #32450, #19342, #19516, #1621, #9461, #16784, #22067, #4172, #9119, #24628, #32624, #29735, #30245, #17297, #3668, #27183, #27685, #16948, #8781, #14732, #32118, #3839, #27343, #25122, #11684, #27007, #19175, #1454, #11850, #29572, #29912, #6738, #6223, #4011, #14567, #14062, #24798, #24458, #6566, #22235, #9286, #19680, #1121, #11513, #21893, #30072, #17128, #24968, #18146, #20525 ),
 .UNSPECIFIED., .F., .F. ) 
 B_SPLINE_CURVE_WITH_KNOTS ( ( 3, 2, 2, 2, 2, 2, 2, 2, 2, 2, 2, 2, 2, 2, 2, 2, 2, 2, 2, 2, 2, 2, 2, 2, 2, 2, 2, 2, 2, 2, 2, 2, 2, 2, 2, 2, 2, 2, 2, 2, 2, 2, 2, 2, 2, 2, 2, 2, 2, 2, 2, 2, 2, 2, 2, 2, 2, 2, 2, 2, 2, 2, 2, 2, 2, 2, 2, 2, 2, 2, 2, 2, 2, 2, 2, 2, 2, 2, 2, 2, 2, 2, 2, 2, 2, 2, 2, 2, 2, 2, 2, 2, 2, 2, 2, 2, 2, 2, 2, 2, 2, 2, 2, 2, 2, 2, 2, 2, 2, 2, 2, 2, 2, 2, 2, 2, 2, 2, 2, 2, 2, 2, 2, 2, 2, 2, 2, 2, 2, 2, 2, 2, 2, 2, 2, 2, 2, 2, 2, 2, 2, 2, 2, 2, 2, 2, 2, 2, 2, 2, 2, 2, 2, 2, 2, 2, 2, 2, 2, 2, 2, 2, 2, 2, 2, 2, 2, 2, 2, 2, 2, 2, 2, 2, 2, 2, 2, 2, 2, 2, 2, 2, 2, 2, 2, 2, 2, 2, 2, 2, 2, 2, 2, 2, 2, 2, 2, 2, 2, 2, 2, 2, 2, 2, 2, 2, 2, 2, 2, 2, 2, 2, 2, 2, 2, 2, 2, 2, 2, 2, 2, 2, 2, 2, 2, 2, 2, 2, 2, 2, 2, 2, 2, 2, 2, 2, 2, 2, 2, 2, 2, 2, 2, 2, 2, 2, 2, 2, 2, 2, 2, 2, 2, 2, 2, 2, 2, 2, 2, 2, 2, 2, 2, 2, 2, 2, 2, 2, 2, 2, 2, 2, 3 ),
 ( 0.000000000000000000, 0.003571428571428571317, 0.007142857142857142634, 0.01071428571428571438, 0.01428571428571428527, 0.01785714285714285615, 0.02142857142857142877, 0.02500000000000000139, 0.02857142857142857054, 0.03214285714285713969, 0.03571428571428571230, 0.03928571428571428492, 0.04285714285714285754, 0.04642857142857143016, 0.05000000000000000278, 0.05357142857142856845, 0.05714285714285714107, 0.06071428571428571369, 0.06428571428571427937, 0.06785714285714285199, 0.07142857142857142461, 0.07499999999999999722, 0.07857142857142856984, 0.08214285714285714246, 0.08571428571428571508, 0.08928571428571428770, 0.09285714285714286031, 0.09642857142857143293, 0.1000000000000000056, 0.1035714285714285782, 0.1071428571428571369, 0.1107142857142857095, 0.1142857142857142821, 0.1178571428571428548, 0.1214285714285714274, 0.1250000000000000000, 0.1285714285714285587, 0.1321428571428571452, 0.1357142857142857040, 0.1392857142857142905, 0.1428571428571428492, 0.1464285714285714357, 0.1499999999999999944, 0.1535714285714285809, 0.1571428571428571397, 0.1607142857142856984, 0.1642857142857142849, 0.1678571428571428437, 0.1714285714285714302, 0.1749999999999999889, 0.1785714285714285754, 0.1821428571428571341, 0.1857142857142857206, 0.1892857142857142794, 0.1928571428571428659, 0.1964285714285714524, 0.2000000000000000111, 0.2035714285714285698, 0.2071428571428571563, 0.2107142857142857151, 0.2142857142857142738, 0.2178571428571428603, 0.2214285714285714191, 0.2250000000000000056, 0.2285714285714285643, 0.2321428571428571230, 0.2357142857142857095, 0.2392857142857142960, 0.2428571428571428548, 0.2464285714285714413, 0.2500000000000000000, 0.2535714285714285587, 0.2571428571428571175, 0.2607142857142857317, 0.2642857142857142905, 0.2678571428571428492, 0.2714285714285714080, 0.2750000000000000222, 0.2785714285714285809, 0.2821428571428571397, 0.2857142857142856984, 0.2892857142857143127, 0.2928571428571428714, 0.2964285714285714302, 0.2999999999999999889, 0.3035714285714285476, 0.3071428571428571619, 0.3107142857142857206, 0.3142857142857142794, 0.3178571428571428381, 0.3214285714285713969, 0.3250000000000000111, 0.3285714285714285698, 0.3321428571428571286, 0.3357142857142856873, 0.3392857142857143016, 0.3428571428571428603, 0.3464285714285714191, 0.3499999999999999778, 0.3535714285714285920, 0.3571428571428571508, 0.3607142857142857095, 0.3642857142857142683, 0.3678571428571428825, 0.3714285714285714413, 0.3750000000000000000, 0.3785714285714285587, 0.3821428571428571175, 0.3857142857142857317, 0.3892857142857142905, 0.3928571428571429047, 0.3964285714285714080, 0.4000000000000000222, 0.4035714285714285809, 0.4071428571428571397, 0.4107142857142856984, 0.4142857142857143127, 0.4178571428571428714, 0.4214285714285714302, 0.4249999999999999889, 0.4285714285714285476, 0.4321428571428571619, 0.4357142857142857206, 0.4392857142857142794, 0.4428571428571428381, 0.4464285714285714524, 0.4500000000000000111, 0.4535714285714285698, 0.4571428571428571286, 0.4607142857142856873, 0.4642857142857142461, 0.4678571428571428603, 0.4714285714285714191, 0.4749999999999999778, 0.4785714285714285920, 0.4821428571428571508, 0.4857142857142857095, 0.4892857142857142683, 0.4928571428571428825, 0.4964285714285714413, 0.5000000000000000000, 0.5035714285714285587, 0.5071428571428571175, 0.5107142857142856762, 0.5142857142857142350, 0.5178571428571429047, 0.5214285714285714635, 0.5250000000000000222, 0.5285714285714285809, 0.5321428571428571397, 0.5357142857142856984, 0.5392857142857142572, 0.5428571428571428159, 0.5464285714285713746, 0.5500000000000000444, 0.5535714285714286031, 0.5571428571428571619, 0.5607142857142857206, 0.5642857142857142794, 0.5678571428571428381, 0.5714285714285713969, 0.5749999999999999556, 0.5785714285714286254, 0.5821428571428571841, 0.5857142857142857428, 0.5892857142857143016, 0.5928571428571428603, 0.5964285714285714191, 0.5999999999999999778, 0.6035714285714285365, 0.6071428571428570953, 0.6107142857142857650, 0.6142857142857143238, 0.6178571428571428825, 0.6214285714285714413, 0.6250000000000000000, 0.6285714285714285587, 0.6321428571428571175, 0.6357142857142856762, 0.6392857142857141239, 0.6428571428571427937, 0.6464285714285714635, 0.6500000000000000222, 0.6535714285714285809, 0.6571428571428571397, 0.6607142857142856984, 0.6642857142857142572, 0.6678571428571428159, 0.6714285714285713746, 0.6750000000000000444, 0.6785714285714286031, 0.6821428571428571619, 0.6857142857142857206, 0.6892857142857142794, 0.6928571428571428381, 0.6964285714285713969, 0.6999999999999999556, 0.7035714285714286254, 0.7071428571428571841, 0.7107142857142857428, 0.7142857142857143016, 0.7178571428571428603, 0.7214285714285714191, 0.7249999999999999778, 0.7285714285714285365, 0.7321428571428570953, 0.7357142857142857650, 0.7392857142857143238, 0.7428571428571428825, 0.7464285714285714413, 0.7500000000000000000, 0.7535714285714285587, 0.7571428571428571175, 0.7607142857142856762, 0.7642857142857142350, 0.7678571428571429047, 0.7714285714285714635, 0.7750000000000000222, 0.7785714285714285809, 0.7821428571428571397, 0.7857142857142858094, 0.7892857142857142572, 0.7928571428571428159, 0.7964285714285713746, 0.8000000000000000444, 0.8035714285714286031, 0.8071428571428571619, 0.8107142857142857206, 0.8142857142857142794, 0.8178571428571428381, 0.8214285714285713969, 0.8249999999999999556, 0.8285714285714286254, 0.8321428571428571841, 0.8357142857142857428, 0.8392857142857143016, 0.8428571428571428603, 0.8464285714285714191, 0.8499999999999999778, 0.8535714285714285365, 0.8571428571428570953, 0.8607142857142857650, 0.8642857142857143238, 0.8678571428571428825, 0.8714285714285714413, 0.8750000000000000000, 0.8785714285714285587, 0.8821428571428571175, 0.8857142857142856762, 0.8892857142857142350, 0.8928571428571429047, 0.8964285714285714635, 0.9000000000000000222, 0.9035714285714285809, 0.9071428571428571397, 0.9107142857142856984, 0.9142857142857142572, 0.9178571428571428159, 0.9214285714285713746, 0.9250000000000000444, 0.9285714285714284921, 0.9321428571428571619, 0.9357142857142857206, 0.9392857142857142794, 0.9428571428571428381, 0.9464285714285713969, 0.9499999999999999556, 0.9535714285714286254, 0.9571428571428571841, 0.9607142857142857428, 0.9642857142857143016, 0.9678571428571428603, 0.9709674003564926492 ),
 .UNSPECIFIED. ) 
 CURVE ( )  GEOMETRIC_REPRESENTATION_ITEM ( )  RATIONAL_B_SPLINE_CURVE ( ( 1.000000000000000000, 0.9510565162951535312, 1.000000000000000000, 0.9510565162951535312, 1.000000000000000000, 0.9510565162951535312, 1.000000000000000000, 0.9510565162951535312, 1.000000000000000000, 0.9510565162951535312, 1.000000000000000000, 0.9510565162951535312, 1.000000000000000000, 0.9510565162951535312, 1.000000000000000000, 0.9510565162951535312, 1.000000000000000000, 0.9510565162951535312, 1.000000000000000000, 0.9510565162951535312, 1.000000000000000000, 0.9510565162951535312, 1.000000000000000000, 0.9510565162951535312, 1.000000000000000000, 0.9510565162951535312, 1.000000000000000000, 0.9510565162951535312, 1.000000000000000000, 0.9510565162951535312, 1.000000000000000000, 0.9510565162951535312, 1.000000000000000000, 0.9510565162951535312, 1.000000000000000000, 0.9510565162951535312, 1.000000000000000000, 0.9510565162951535312, 1.000000000000000000, 0.9510565162951535312, 1.000000000000000000, 0.9510565162951535312, 1.000000000000000000, 0.9510565162951535312, 1.000000000000000000, 0.9510565162951535312, 1.000000000000000000, 0.9510565162951535312, 1.000000000000000000, 0.9510565162951535312, 1.000000000000000000, 0.9510565162951535312, 1.000000000000000000, 0.9510565162951535312, 1.000000000000000000, 0.9510565162951535312, 1.000000000000000000, 0.9510565162951535312, 1.000000000000000000, 0.9510565162951535312, 1.000000000000000000, 0.9510565162951535312, 1.000000000000000000, 0.9510565162951535312, 1.000000000000000000, 0.9510565162951535312, 1.000000000000000000, 0.9510565162951535312, 1.000000000000000000, 0.9510565162951535312, 1.000000000000000000, 0.9510565162951535312, 1.000000000000000000, 0.9510565162951535312, 1.000000000000000000, 0.9510565162951535312, 1.000000000000000000, 0.9510565162951535312, 1.000000000000000000, 0.9510565162951535312, 1.000000000000000000, 0.9510565162951535312, 1.000000000000000000, 0.9510565162951535312, 1.000000000000000000, 0.9510565162951535312, 1.000000000000000000, 0.9510565162951535312, 1.000000000000000000, 0.9510565162951535312, 1.000000000000000000, 0.9510565162951535312, 1.000000000000000000, 0.9510565162951535312, 1.000000000000000000, 0.9510565162951535312, 1.000000000000000000, 0.9510565162951535312, 1.000000000000000000, 0.9510565162951535312, 1.000000000000000000, 0.9510565162951535312, 1.000000000000000000, 0.9510565162951535312, 1.000000000000000000, 0.9510565162951535312, 1.000000000000000000, 0.9510565162951535312, 1.000000000000000000, 0.9510565162951535312, 1.000000000000000000, 0.9510565162951535312, 1.000000000000000000, 0.9510565162951535312, 1.000000000000000000, 0.9510565162951535312, 1.000000000000000000, 0.9510565162951535312, 1.000000000000000000, 0.9510565162951535312, 1.000000000000000000, 0.9510565162951535312, 1.000000000000000000, 0.9510565162951535312, 1.000000000000000000, 0.9510565162951535312, 1.000000000000000000, 0.9510565162951535312, 1.000000000000000000, 0.9510565162951535312, 1.000000000000000000, 0.9510565162951535312, 1.000000000000000000, 0.9510565162951535312, 1.000000000000000000, 0.9510565162951535312, 1.000000000000000000, 0.9510565162951535312, 1.000000000000000000, 0.9510565162951535312, 1.000000000000000000, 0.9510565162951535312, 1.000000000000000000, 0.9510565162951535312, 1.000000000000000000, 0.9510565162951535312, 1.000000000000000000, 0.9510565162951535312, 1.000000000000000000, 0.9510565162951535312, 1.000000000000000000, 0.9510565162951535312, 1.000000000000000000, 0.9510565162951535312, 1.000000000000000000, 0.9510565162951535312, 1.000000000000000000, 0.9510565162951535312, 1.000000000000000000, 0.9510565162951535312, 1.000000000000000000, 0.9510565162951535312, 1.000000000000000000, 0.9510565162951535312, 1.000000000000000000, 0.9510565162951535312, 1.000000000000000000, 0.9510565162951535312, 1.000000000000000000, 0.9510565162951535312, 1.000000000000000000, 0.9510565162951535312, 1.000000000000000000, 0.9510565162951535312, 1.000000000000000000, 0.9510565162951535312, 1.000000000000000000, 0.9510565162951535312, 1.000000000000000000, 0.9510565162951535312, 1.000000000000000000, 0.9510565162951535312, 1.000000000000000000, 0.9510565162951535312, 1.000000000000000000, 0.9510565162951535312, 1.000000000000000000, 0.9510565162951535312, 1.000000000000000000, 0.9510565162951535312, 1.000000000000000000, 0.9510565162951535312, 1.000000000000000000, 0.9510565162951535312, 1.000000000000000000, 0.9510565162951535312, 1.000000000000000000, 0.9510565162951535312, 1.000000000000000000, 0.9510565162951535312, 1.000000000000000000, 0.9510565162951535312, 1.000000000000000000, 0.9510565162951535312, 1.000000000000000000, 0.9510565162951535312, 1.000000000000000000, 0.9510565162951535312, 1.000000000000000000, 0.9510565162951535312, 1.000000000000000000, 0.9510565162951535312, 1.000000000000000000, 0.9510565162951535312, 1.000000000000000000, 0.9510565162951535312, 1.000000000000000000, 0.9510565162951535312, 1.000000000000000000, 0.9510565162951535312, 1.000000000000000000, 0.9510565162951535312, 1.000000000000000000, 0.9510565162951535312, 1.000000000000000000, 0.9510565162951535312, 1.000000000000000000, 0.9510565162951535312, 1.000000000000000000, 0.9510565162951535312, 1.000000000000000000, 0.9510565162951535312, 1.000000000000000000, 0.9510565162951535312, 1.000000000000000000, 0.9510565162951535312, 1.000000000000000000, 0.9510565162951535312, 1.000000000000000000, 0.9510565162951535312, 1.000000000000000000, 0.9510565162951535312, 1.000000000000000000, 0.9510565162951535312, 1.000000000000000000, 0.9510565162951535312, 1.000000000000000000, 0.9510565162951535312, 1.000000000000000000, 0.9510565162951535312, 1.000000000000000000, 0.9510565162951535312, 1.000000000000000000, 0.9510565162951535312, 1.000000000000000000, 0.9510565162951535312, 1.000000000000000000, 0.9510565162951535312, 1.000000000000000000, 0.9510565162951535312, 1.000000000000000000, 0.9510565162951535312, 1.000000000000000000, 0.9510565162951535312, 1.000000000000000000, 0.9510565162951535312, 1.000000000000000000, 0.9510565162951535312, 1.000000000000000000, 0.9510565162951535312, 1.000000000000000000, 0.9510565162951535312, 1.000000000000000000, 0.9510565162951535312, 1.000000000000000000, 0.9510565162951535312, 1.000000000000000000, 0.9510565162951535312, 1.000000000000000000, 0.9510565162951535312, 1.000000000000000000, 0.9510565162951535312, 1.000000000000000000, 0.9510565162951535312, 1.000000000000000000, 0.9510565162951535312, 1.000000000000000000, 0.9510565162951535312, 1.000000000000000000, 0.9510565162951535312, 1.000000000000000000, 0.9510565162951535312, 1.000000000000000000, 0.9510565162951535312, 1.000000000000000000, 0.9510565162951535312, 1.000000000000000000, 0.9510565162951535312, 1.000000000000000000, 0.9510565162951535312, 1.000000000000000000, 0.9510565162951535312, 1.000000000000000000, 0.9510565162951535312, 1.000000000000000000, 0.9510565162951535312, 1.000000000000000000, 0.9510565162951535312, 1.000000000000000000, 0.9510565162951535312, 1.000000000000000000, 0.9510565162951535312, 1.000000000000000000, 0.9510565162951535312, 1.000000000000000000, 0.9510565162951535312, 1.000000000000000000, 0.9510565162951535312, 1.000000000000000000, 0.9510565162951535312, 1.000000000000000000, 0.9510565162951535312, 1.000000000000000000, 0.9510565162951535312, 1.000000000000000000, 0.9510565162951535312, 1.000000000000000000, 0.9510565162951535312, 1.000000000000000000, 0.9510565162951535312, 1.000000000000000000, 0.9510565162951535312, 1.000000000000000000, 0.9510565162951535312, 1.000000000000000000, 0.9510565162951535312, 1.000000000000000000, 0.9510565162951535312, 1.000000000000000000, 0.9510565162951535312, 1.000000000000000000, 0.9510565162951535312, 1.000000000000000000, 0.9510565162951535312, 1.000000000000000000, 0.9510565162951535312, 1.000000000000000000, 0.9510565162951535312, 1.000000000000000000, 0.9510565162951535312, 1.000000000000000000, 0.9510565162951535312, 1.000000000000000000, 0.9510565162951535312, 1.000000000000000000, 0.9510565162951535312, 1.000000000000000000, 0.9510565162951535312, 1.000000000000000000, 0.9510565162951535312, 1.000000000000000000, 0.9510565162951535312, 1.000000000000000000, 0.9510565162951535312, 1.000000000000000000, 0.9510565162951535312, 1.000000000000000000, 0.9510565162951535312, 1.000000000000000000, 0.9510565162951535312, 1.000000000000000000, 0.9510565162951535312, 1.000000000000000000, 0.9510565162951535312, 1.000000000000000000, 0.9510565162951535312, 1.000000000000000000, 0.9510565162951535312, 1.000000000000000000, 0.9510565162951535312, 1.000000000000000000, 0.9510565162951535312, 1.000000000000000000, 0.9510565162951535312, 1.000000000000000000, 0.9510565162951535312, 1.000000000000000000, 0.9510565162951535312, 1.000000000000000000, 0.9510565162951535312, 1.000000000000000000, 0.9510565162951535312, 1.000000000000000000, 0.9510565162951535312, 1.000000000000000000, 0.9510565162951535312, 1.000000000000000000, 0.9510565162951535312, 1.000000000000000000, 0.9510565162951535312, 1.000000000000000000, 0.9510565162951535312, 1.000000000000000000, 0.9510565162951535312, 1.000000000000000000, 0.9510565162951535312, 1.000000000000000000, 0.9510565162951535312, 1.000000000000000000, 0.9510565162951535312, 1.000000000000000000, 0.9510565162951535312, 1.000000000000000000, 0.9510565162951535312, 1.000000000000000000, 0.9510565162951535312, 1.000000000000000000, 0.9510565162951535312, 1.000000000000000000, 0.9510565162951535312, 1.000000000000000000, 0.9510565162951535312, 1.000000000000000000, 0.9510565162951535312, 1.000000000000000000, 0.9510565162951535312, 1.000000000000000000, 0.9510565162951535312, 1.000000000000000000, 0.9510565162951535312, 1.000000000000000000, 0.9510565162951535312, 1.000000000000000000, 0.9510565162951535312, 1.000000000000000000, 0.9510565162951535312, 1.000000000000000000, 0.9510565162951535312, 1.000000000000000000, 0.9510565162951535312, 1.000000000000000000, 0.9510565162951535312, 1.000000000000000000, 0.9510565162951535312, 1.000000000000000000, 0.9510565162951535312, 1.000000000000000000, 0.9510565162951535312, 1.000000000000000000, 0.9510565162951535312, 1.000000000000000000, 0.9510565162951535312, 1.000000000000000000, 0.9510565162951535312, 1.000000000000000000, 0.9510565162951535312, 1.000000000000000000, 0.9510565162951535312, 1.000000000000000000, 0.9510565162951535312, 1.000000000000000000, 0.9510565162951535312, 1.000000000000000000, 0.9510565162951535312, 1.000000000000000000, 0.9510565162951535312, 1.000000000000000000, 0.9510565162951535312, 1.000000000000000000, 0.9510565162951535312, 1.000000000000000000, 0.9510565162951535312, 1.000000000000000000, 0.9510565162951535312, 1.000000000000000000, 0.9510565162951535312, 1.000000000000000000, 0.9510565162951535312, 1.000000000000000000, 0.9510565162951535312, 1.000000000000000000, 0.9510565162951535312, 1.000000000000000000, 0.9510565162951535312, 1.000000000000000000, 0.9510565162951535312, 1.000000000000000000, 0.9510565162951535312, 1.000000000000000000, 0.9510565162951535312, 1.000000000000000000, 0.9510565162951535312, 1.000000000000000000, 0.9510565162951535312, 1.000000000000000000, 0.9510565162951535312, 1.000000000000000000, 0.9510565162951535312, 1.000000000000000000, 0.9510565162951535312, 1.000000000000000000, 0.9510565162951535312, 1.000000000000000000, 0.9510565162951535312, 1.000000000000000000, 0.9510565162951535312, 1.000000000000000000, 0.9510565162951535312, 1.000000000000000000, 0.9510565162951535312, 1.000000000000000000, 0.9510565162951535312, 1.000000000000000000, 0.9510565162951535312, 1.000000000000000000, 0.9510565162951535312, 1.000000000000000000, 0.9510565162951535312, 1.000000000000000000, 0.9510565162951535312, 1.000000000000000000, 0.9510565162951535312, 1.000000000000000000, 0.9510565162951535312, 1.000000000000000000, 0.9510565162951535312, 1.000000000000000000, 0.9510565162951535312, 1.000000000000000000, 0.9510565162951535312, 1.000000000000000000, 0.9510565162951535312, 1.000000000000000000, 0.9510565162951535312, 1.000000000000000000, 0.9510565162951535312, 1.000000000000000000, 0.9510565162951535312, 1.000000000000000000, 0.9510565162951535312, 1.000000000000000000, 0.9510565162951535312, 1.000000000000000000, 0.9573764855735550361, 0.9889922301674671790 ) ) 
 REPRESENTATION_ITEM ( '' )  );
#5966=FACE_OUTER_BOUND ( 'NONE', #25364, .T. ) ;
#5973=CARTESIAN_POINT ( 'NONE',  ( 48.17499999726881299, 164.1591823560292198, 12.60653300113718167 ) ) ;
#5975=CARTESIAN_POINT ( 'NONE',  ( 60.32499999726881157, 145.8408176439707802, 12.60653300113718345 ) ) ;
#5976=DIRECTION ( 'NONE',  ( 0.000000000000000000, -1.000000000000000000, 6.454785026890489601E-15 ) ) ;
#5980=CARTESIAN_POINT ( 'NONE',  ( 55.37499999726881583, 155.0000000000000000, -15.58253175000000823 ) ) ;
#5985=VECTOR ( 'NONE', #2751, 1000.000000000000000 ) ;
#5986=CARTESIAN_POINT ( 'NONE',  ( 73.79999999999999716, 142.6655632788954620, 8.961492836873471646 ) ) ;
#5987=CARTESIAN_POINT ( 'NONE',  ( 40.78867513459481842, 155.0000000000000000, -15.00000000000002487 ) ) ;
#5988=CARTESIAN_POINT ( 'NONE',  ( 125.5000000000000000, 155.0000000000000000, -6.938893903907228378E-15 ) ) ;
#5990=CARTESIAN_POINT ( 'NONE',  ( 125.5000000000000000, 229.9533188057749555, 74.95331880577313655 ) ) ;
#5991=CARTESIAN_POINT ( 'NONE',  ( 38.87499999726880873, 138.6155565068815463, -3.929120461958505118E-15 ) ) ;
#5993=CARTESIAN_POINT ( 'NONE',  ( 78.02499999726879309, 160.0630714827496206, 15.58253174999999402 ) ) ;
#5997=CARTESIAN_POINT ( 'NONE',  ( 43.79999999453762172, 146.4771138417591203, -11.73074641843674470 ) ) ;
#5999=CARTESIAN_POINT ( 'NONE',  ( 40.41132485994280898, 167.7597621252805880, 9.270509831248428867 ) ) ;
#6000=DIRECTION ( 'NONE',  ( 1.000000000000000000, 0.000000000000000000, 0.000000000000000000 ) ) ;
#6009=CARTESIAN_POINT ( 'NONE',  ( 70.78867513459482552, 155.0000000000000000, -15.00000000000002487 ) ) ;
#6017=CARTESIAN_POINT ( 'NONE',  ( 33.87499999726881583, 171.3844434931184253, -7.942151717890132712E-15 ) ) ;
#6021=CARTESIAN_POINT ( 'NONE',  ( 53.69999999999999574, 146.4771138417591203, 11.73074641843673227 ) ) ;
#6024=CARTESIAN_POINT ( 'NONE',  ( 60.42499999726881299, 141.7447067706911810, 9.630534252274376428 ) ) ;
#6028=CARTESIAN_POINT ( 'NONE',  ( 65.82499999726883289, 168.2552932293087906, 9.630534252274372875 ) ) ;
#6029=CARTESIAN_POINT ( 'NONE',  ( 75.97499999726881015, 169.8198683612136222, 4.815267126137181997 ) ) ;
#6044=ORIENTED_EDGE ( 'NONE', *, *, #10231, .T. ) ;
#6051=CARTESIAN_POINT ( 'NONE',  ( 75.12499999726881583, 155.0000000000000000, -15.58253175000000823 ) ) ;
#6055=CARTESIAN_POINT ( 'NONE',  ( 68.82499999726880446, 141.7447067706911810, -9.630534252274385310 ) ) ;
#6059=CARTESIAN_POINT ( 'NONE',  ( 37.59999999999999432, 150.2886644046228639, 14.49999999999999645 ) ) ;
#6066=CARTESIAN_POINT ( 'NONE',  ( 60.58867513459482979, 146.1832212156128890, -12.13525491562423042 ) ) ;
#6067=CARTESIAN_POINT ( 'NONE',  ( 42.12499999726881583, 155.0000000000000000, 15.58253174999999402 ) ) ;
#6074=CARTESIAN_POINT ( 'NONE',  ( 85.09999999453764019, 150.2886644046228639, 14.49999999999999645 ) ) ;
#6084=ORIENTED_EDGE ( 'NONE', *, *, #32854, .F. ) ;
#6085=CARTESIAN_POINT ( 'NONE',  ( 78.97499999726881015, 140.1801316387863778, -4.815267126137194431 ) ) ;
#6091=CARTESIAN_POINT ( 'NONE',  ( 69.47499999726882436, 160.0630714827496206, -15.58253175000000823 ) ) ;
#6092=ORIENTED_EDGE ( 'NONE', *, *, #16655, .T. ) ;
#6093=CARTESIAN_POINT ( 'NONE',  ( 61.98867513459482836, 146.1832212156128890, 12.13525491562421976 ) ) ;
#6096=CARTESIAN_POINT ( 'NONE',  ( 52.18867513459482410, 140.7341522555726669, 4.635254915624211769 ) ) ;
#6102=CARTESIAN_POINT ( 'NONE',  ( 83.57499999726880446, 164.1591823560292198, -12.60653300113719766 ) ) ;
#6105=VECTOR ( 'NONE', #18772, 1000.000000000000000 ) ;
#6106=CARTESIAN_POINT ( 'NONE',  ( 40.92499999726881299, 145.8408176439707802, -12.60653300113719588 ) ) ;
#6111=CARTESIAN_POINT ( 'NONE',  ( 60.57499999726881157, 145.8408176439707802, 12.60653300113718345 ) ) ;
#6119=CARTESIAN_POINT ( 'NONE',  ( 65.99999999453761745, 155.0000000000000000, -14.50000000000000711 ) ) ;
#6120=EDGE_LOOP ( 'NONE', ( #24074, #20729, #30226, #21111 ) ) ;
#6123=LINE ( 'NONE', #25494, #21344 ) ;
#6140=CARTESIAN_POINT ( 'NONE',  ( 47.77499999726881441, 169.8198683612136222, -4.815267126137197984 ) ) ;
#6141=ORIENTED_EDGE ( 'NONE', *, *, #3918, .F. ) ;
#6142=CARTESIAN_POINT ( 'NONE',  ( 56.92499999726881299, 145.8408176439707802, -12.60653300113719588 ) ) ;
#6147=CARTESIAN_POINT ( 'NONE',  ( 62.57499999726881867, 145.8408176439707802, 12.60653300113718345 ) ) ;
#6152=CARTESIAN_POINT ( 'NONE',  ( 71.80000000000001137, 142.6655632788954620, 8.961492836873471646 ) ) ;
#6153=CARTESIAN_POINT ( 'NONE',  ( 65.38867513459483405, 169.2658477444273331, 4.635254915624208216 ) ) ;
#6156=CARTESIAN_POINT ( 'NONE',  ( 33.08867513459482979, 167.7597621252805880, -9.270509831248443078 ) ) ;
#6157=CARTESIAN_POINT ( 'NONE',  ( 42.47499999726880304, 149.9369285172503510, 15.58253174999999580 ) ) ;
#6159=CARTESIAN_POINT ( 'NONE',  ( 78.72499999726881015, 140.1801316387863778, -4.815267126137194431 ) ) ;
#6160=ORIENTED_EDGE ( 'NONE', *, *, #19153, .F. ) ;
#6161=CARTESIAN_POINT ( 'NONE',  ( 48.21132485994281325, 170.7719333635740497, -7.904646289410545231E-15 ) ) ;
#6163=CARTESIAN_POINT ( 'NONE',  ( 38.29999999453762882, 167.3344367211045096, -8.961492836873482304 ) ) ;
#6164=( BOUNDED_CURVE ( )  B_SPLINE_CURVE ( 2, ( #26716, #8179, #23833, #24169, #18564, #19224, #31999, #28949, #6093, #16491, #29621 ),
 .UNSPECIFIED., .F., .T. ) 
 B_SPLINE_CURVE_WITH_KNOTS ( ( 3, 2, 2, 2, 2, 3 ),
 ( 0.4464285714285712858, 0.4499999999999998446, 0.4535714285714284588, 0.4571428571428570176, 0.4607142857142856318, 0.4642857142857141906 ),
 .UNSPECIFIED. ) 
 CURVE ( )  GEOMETRIC_REPRESENTATION_ITEM ( )  RATIONAL_B_SPLINE_CURVE ( ( 1.000000000000001554, 0.9510565162951518658, 1.000000000000000000, 0.9510565162951534202, 1.000000000000000000, 0.9510565162951534202, 1.000000000000000000, 0.9510565162951534202, 1.000000000000000000, 0.9510565162951534202, 1.000000000000000000 ) ) 
 REPRESENTATION_ITEM ( '' )  );
#6179=CARTESIAN_POINT ( 'NONE',  ( 79.78867513459482552, 155.0000000000000000, 15.00000000000001243 ) ) ;
#6184=CARTESIAN_POINT ( 'NONE',  ( 33.67499999726881299, 168.2552932293087906, -9.630534252274387086 ) ) ;
#6186=CARTESIAN_POINT ( 'NONE',  ( 35.42499999726880588, 168.2552932293087906, -9.630534252274385310 ) ) ;
#6187=ADVANCED_FACE ( 'NONE', ( #14021 ), #9417, .T. ) ;
#6191=CARTESIAN_POINT ( 'NONE',  ( 40.57499999726881157, 145.8408176439707802, 12.60653300113718345 ) ) ;
#6194=CARTESIAN_POINT ( 'NONE',  ( 56.30000000000000426, 146.4771138417591203, -11.73074641843674470 ) ) ;
#6196=DIRECTION ( 'NONE',  ( 1.000000000000000000, 0.000000000000000000, 0.000000000000000000 ) ) ;
#6198=CARTESIAN_POINT ( 'NONE',  ( 57.02499999726882152, 149.9369285172503510, -15.58253175000000823 ) ) ;
#6201=CARTESIAN_POINT ( 'NONE',  ( 67.82499999726881867, 168.2552932293087906, 9.630534252274372875 ) ) ;
#6202=CARTESIAN_POINT ( 'NONE',  ( 74.67499999726879878, 141.7447067706911810, 9.630534252274376428 ) ) ;
#6223=CARTESIAN_POINT ( 'NONE',  ( 85.82499999726879025, 168.2552932293087906, 9.630534252274372875 ) ) ;
#6224=ORIENTED_EDGE ( 'NONE', *, *, #16821, .T. ) ;
#6225=CARTESIAN_POINT ( 'NONE',  ( 69.11132485994281183, 140.7341522555726669, 4.635254915624211769 ) ) ;
#6227=CARTESIAN_POINT ( 'NONE',  ( 71.92499999726881299, 164.1591823560292198, 12.60653300113718167 ) ) ;
#6232=CARTESIAN_POINT ( 'NONE',  ( 37.90000000000000568, 141.2096805137202580, 4.480746418436733158 ) ) ;
#6242=CARTESIAN_POINT ( 'NONE',  ( 41.72499999726881015, 169.8198683612136222, 4.815267126137181997 ) ) ;
#6250=CARTESIAN_POINT ( 'NONE',  ( 88.79999999453764303, 163.5228861582408797, 11.73074641843673049 ) ) ;
#6255=ORIENTED_EDGE ( 'NONE', *, *, #2441, .T. ) ;
#6258=CARTESIAN_POINT ( 'NONE',  ( 73.17499999726881299, 145.8408176439707802, -12.60653300113719588 ) ) ;
#6261=CARTESIAN_POINT ( 'NONE',  ( 79.37499999726881583, 155.0000000000000000, -15.58253175000000823 ) ) ;
#6265=EDGE_CURVE ( 'NONE', #28846, #9319, #9648, .T. ) ;
#6267=CARTESIAN_POINT ( 'NONE',  ( 70.07499999726881867, 168.2552932293087906, 9.630534252274372875 ) ) ;
#6269=CARTESIAN_POINT ( 'NONE',  ( 68.18867513459483121, 140.7341522555726669, 4.635254915624211769 ) ) ;
#6271=CARTESIAN_POINT ( 'NONE',  ( 43.38867513459481984, 169.2658477444273331, 4.635254915624208216 ) ) ;
#6276=CARTESIAN_POINT ( 'NONE',  ( 85.67499999726879878, 168.2552932293087906, -9.630534252274385310 ) ) ;
#6278=CARTESIAN_POINT ( 'NONE',  ( 43.52499999726881441, 169.8198683612136222, -4.815267126137197984 ) ) ;
#6289=CARTESIAN_POINT ( 'NONE',  ( 67.19999999453763451, 146.4771138417591203, 11.73074641843673227 ) ) ;
#6290=VERTEX_POINT ( 'NONE', #31317 ) ;
#6304=( BOUNDED_CURVE ( )  B_SPLINE_CURVE ( 2, ( #29962, #6961, #6618, #17003, #17175, #14450, #24844, #1507, #33486, #11905, #22291 ),
 .UNSPECIFIED., .F., .F. ) 
 B_SPLINE_CURVE_WITH_KNOTS ( ( 3, 2, 2, 2, 2, 3 ),
 ( 0.6607142857142856984, 0.6642857142857142572, 0.6678571428571428159, 0.6714285714285712636, 0.6749999999999999334, 0.6785714285714284921 ),
 .UNSPECIFIED. ) 
 CURVE ( )  GEOMETRIC_REPRESENTATION_ITEM ( )  RATIONAL_B_SPLINE_CURVE ( ( 1.000000000000000000, 0.9510565162951534202, 1.000000000000000000, 0.9510565162951534202, 1.000000000000000000, 0.9510565162951534202, 1.000000000000000000, 0.9510565162951534202, 1.000000000000000000, 0.9510565162951549745, 0.9999999999999984457 ) ) 
 REPRESENTATION_ITEM ( '' )  );
#6307=CARTESIAN_POINT ( 'NONE',  ( 49.07499999726881157, 141.7447067706911810, -9.630534252274387086 ) ) ;
#6309=CARTESIAN_POINT ( 'NONE',  ( 59.02499999726880731, 149.9369285172503510, -15.58253175000000823 ) ) ;
#6311=CARTESIAN_POINT ( 'NONE',  ( 60.78867513459481842, 155.0000000000000000, -15.00000000000002487 ) ) ;
#6315=CARTESIAN_POINT ( 'NONE',  ( 61.47499999726879594, 160.0630714827496206, -15.58253175000000823 ) ) ;
#6321=CARTESIAN_POINT ( 'NONE',  ( 75.60000000000000853, 150.2886644046228639, 14.49999999999999645 ) ) ;
#6322=CARTESIAN_POINT ( 'NONE',  ( 40.08867513459482979, 142.2402378747194405, 9.270509831248432420 ) ) ;
#6325=FACE_OUTER_BOUND ( 'NONE', #2508, .T. ) ;
#6326=CARTESIAN_POINT ( 'NONE',  ( 44.47499999726879594, 149.9369285172503510, 15.58253174999999580 ) ) ;
#6328=EDGE_CURVE ( 'NONE', #5021, #20942, #4817, .T. ) ;
#6329=AXIS2_PLACEMENT_3D ( 'NONE', #18023, #295, #13239 ) ;
#6330=CARTESIAN_POINT ( 'NONE',  ( 76.32499999726881867, 145.8408176439707802, 12.60653300113718345 ) ) ;
#6332=CARTESIAN_POINT ( 'NONE',  ( 51.81132485994281467, 159.8737954434937478, -14.99999999999993072 ) ) ;
#6333=CARTESIAN_POINT ( 'NONE',  ( 47.19999999453762740, 146.4771138417591203, 11.73074641843673227 ) ) ;
#6338=VERTEX_POINT ( 'NONE', #26038 ) ;
#6340=CARTESIAN_POINT ( 'NONE',  ( 85.78867513459481131, 155.0000000000000000, 15.00000000000001243 ) ) ;
#6347=CARTESIAN_POINT ( 'NONE',  ( 50.38867513459482694, 140.7341522555726669, -4.635254915624220651 ) ) ;
#6352=CARTESIAN_POINT ( 'NONE',  ( 32.50000000000000000, 155.0000000000000000, -6.938893903907228378E-15 ) ) ;
#6355=CARTESIAN_POINT ( 'NONE',  ( 40.52499999726881441, 140.1801316387863778, 4.815267126137185549 ) ) ;
#6357=CARTESIAN_POINT ( 'NONE',  ( 43.07499999726881157, 141.7447067706911810, -9.630534252274385310 ) ) ;
#6360=CARTESIAN_POINT ( 'NONE',  ( 53.40000000000000568, 159.7113355953771077, 14.49999999999999289 ) ) ;
#6369=CARTESIAN_POINT ( 'NONE',  ( 54.72499999726881015, 140.1801316387863778, -4.815267126137194431 ) ) ;
#6372=ORIENTED_EDGE ( 'NONE', *, *, #16423, .T. ) ;
#6374=CARTESIAN_POINT ( 'NONE',  ( 81.27499999726877888, 149.9369285172503510, -15.58253175000000823 ) ) ;
#6396=EDGE_LOOP ( 'NONE', ( #12689, #1942, #23086, #31010 ) ) ;
#6398=CARTESIAN_POINT ( 'NONE',  ( 81.52499999726880731, 169.8198683612136222, -4.815267126137197984 ) ) ;
#6399=ORIENTED_EDGE ( 'NONE', *, *, #22723, .T. ) ;
#6404=CARTESIAN_POINT ( 'NONE',  ( 74.92499999726881299, 145.8408176439707802, -12.60653300113719588 ) ) ;
#6409=CARTESIAN_POINT ( 'NONE',  ( 38.29999999999999716, 146.4771138417591203, -11.73074641843674470 ) ) ;
#6413=EDGE_CURVE ( 'NONE', #9970, #8044, #12037, .T. ) ;
#6416=DIRECTION ( 'NONE',  ( 1.000000000000000000, 0.000000000000000000, 0.000000000000000000 ) ) ;
#6417=CARTESIAN_POINT ( 'NONE',  ( 50.42499999726880588, 141.7447067706911810, 9.630534252274376428 ) ) ;
#6424=AXIS2_PLACEMENT_3D ( 'NONE', #26924, #14143, #32036 ) ;
#6427=CARTESIAN_POINT ( 'NONE',  ( 82.99999999453763166, 155.0000000000000000, 14.49999999999999467 ) ) ;
#6437=CARTESIAN_POINT ( 'NONE',  ( 74.37499999726881583, 155.0000000000000000, 15.58253174999999402 ) ) ;
#6441=CARTESIAN_POINT ( 'NONE',  ( 86.47499999726881015, 149.9369285172503510, 15.58253174999999580 ) ) ;
#6449=CARTESIAN_POINT ( 'NONE',  ( 67.67499999726881299, 168.2552932293087906, -9.630534252274387086 ) ) ;
#6450=ORIENTED_EDGE ( 'NONE', *, *, #8545, .T. ) ;
#6453=CARTESIAN_POINT ( 'NONE',  ( 52.08867513459482268, 142.2402378747194405, 9.270509831248432420 ) ) ;
#6460=CARTESIAN_POINT ( 'NONE',  ( 44.82499999726880446, 141.7447067706911810, -9.630534252274385310 ) ) ;
#6467=CARTESIAN_POINT ( 'NONE',  ( 32.50000000000000000, 155.0000000000000000, -15.00000000000002487 ) ) ;
#6471=CARTESIAN_POINT ( 'NONE',  ( 64.69999999453762030, 167.3344367211045096, 8.961492836873468093 ) ) ;
#6486=CARTESIAN_POINT ( 'NONE',  ( 42.78867513459481842, 155.0000000000000000, -15.00000000000002487 ) ) ;
#6488=ORIENTED_EDGE ( 'NONE', *, *, #15413, .F. ) ;
#6492=CARTESIAN_POINT ( 'NONE',  ( 50.37499999726881583, 155.0000000000000000, 15.58253174999999402 ) ) ;
#6499=CARTESIAN_POINT ( 'NONE',  ( 59.67499999726880588, 168.2552932293087906, -9.630534252274385310 ) ) ;
#6501=DIRECTION ( 'NONE',  ( 1.000000000000000000, 0.000000000000000000, 0.000000000000000000 ) ) ;
#6503=CARTESIAN_POINT ( 'NONE',  ( 83.19999999999998863, 167.3344367211045096, 8.961492836873468093 ) ) ;
#6504=CARTESIAN_POINT ( 'NONE',  ( 65.78867513459482552, 155.0000000000000000, 15.00000000000001243 ) ) ;
#6505=CARTESIAN_POINT ( 'NONE',  ( 117.5000000000000142, 155.0000000000000000, -6.938893903907228378E-15 ) ) ;
#6508=CARTESIAN_POINT ( 'NONE',  ( 45.87499999726880162, 171.3844434931184253, -7.942151717890132712E-15 ) ) ;
#6510=CARTESIAN_POINT ( 'NONE',  ( 85.02499999726882152, 149.9369285172503510, -15.58253175000000823 ) ) ;
#6514=CARTESIAN_POINT ( 'NONE',  ( 49.99999999453763166, 155.0000000000000000, -14.50000000000000711 ) ) ;
#6523=( BOUNDED_CURVE ( )  B_SPLINE_CURVE ( 2, ( #26333, #30960, #15602, #5545, #2999, #13378, #23776, #12886, #13217, #18335, #29058 ),
 .UNSPECIFIED., .F., .T. ) 
 B_SPLINE_CURVE_WITH_KNOTS ( ( 3, 2, 2, 2, 2, 3 ),
 ( 0.9464285714285712858, 0.9499999999999998446, 0.9535714285714284033, 0.9571428571428569620, 0.9607142857142855208, 0.9642857142857140795 ),
 .UNSPECIFIED. ) 
 CURVE ( )  GEOMETRIC_REPRESENTATION_ITEM ( )  RATIONAL_B_SPLINE_CURVE ( ( 1.000000000000001554, 0.9510565162951518658, 1.000000000000000000, 0.9510565162951534202, 1.000000000000000000, 0.9510565162951534202, 1.000000000000000000, 0.9510565162951534202, 1.000000000000000000, 0.9510565162951549745, 0.9999999999999984457 ) ) 
 REPRESENTATION_ITEM ( '' )  );
#6525=CARTESIAN_POINT ( 'NONE',  ( 79.48867513459484258, 167.7597621252805880, 9.270509831248428867 ) ) ;
#6526=VERTEX_POINT ( 'NONE', #802 ) ;
#6532=CARTESIAN_POINT ( 'NONE',  ( 36.12499999726881583, 155.0000000000000000, 15.58253174999999402 ) ) ;
#6533=CARTESIAN_POINT ( 'NONE',  ( 39.18867513459482410, 169.2658477444273331, -4.635254915624224203 ) ) ;
#6535=CARTESIAN_POINT ( 'NONE',  ( 37.77499999726881441, 169.8198683612136222, -4.815267126137197984 ) ) ;
#6538=CARTESIAN_POINT ( 'NONE',  ( 63.79999999999999716, 142.6655632788954620, 8.961492836873471646 ) ) ;
#6541=DIRECTION ( 'NONE',  ( 1.000000000000000000, 0.000000000000000000, 0.000000000000000000 ) ) ;
#6543=CARTESIAN_POINT ( 'NONE',  ( 57.52499999726881441, 169.8198683612136222, -4.815267126137197984 ) ) ;
#6545=ORIENTED_EDGE ( 'NONE', *, *, #27084, .T. ) ;
#6547=CARTESIAN_POINT ( 'NONE',  ( 84.07499999726877604, 168.2552932293087906, 9.630534252274372875 ) ) ;
#6550=CARTESIAN_POINT ( 'NONE',  ( 53.48867513459483547, 167.7597621252805880, 9.270509831248428867 ) ) ;
#6559=CARTESIAN_POINT ( 'NONE',  ( 38.71132485994280614, 155.0000000000000000, 15.00000000000001243 ) ) ;
#6566=CARTESIAN_POINT ( 'NONE',  ( 86.42499999726881299, 141.7447067706911810, 9.630534252274376428 ) ) ;
#6569=CARTESIAN_POINT ( 'NONE',  ( 73.32499999726880446, 164.1591823560292198, -12.60653300113719766 ) ) ;
#6575=CARTESIAN_POINT ( 'NONE',  ( 38.40000000000000568, 150.2886644046228639, -14.50000000000000888 ) ) ;
#6579=CARTESIAN_POINT ( 'NONE',  ( 73.21132485994282035, 139.2280666364260071, -4.041636747397287284E-15 ) ) ;
#6581=CARTESIAN_POINT ( 'NONE',  ( 53.82499999726880446, 168.2552932293087906, 9.630534252274372875 ) ) ;
#6589=CARTESIAN_POINT ( 'NONE',  ( 85.29999999453761461, 142.6655632788954620, 8.961492836873471646 ) ) ;
#6599=CARTESIAN_POINT ( 'NONE',  ( 69.57499999726881867, 164.1591823560292198, -12.60653300113719766 ) ) ;
#6603=CARTESIAN_POINT ( 'NONE',  ( 83.87499999726880162, 171.3844434931184253, -7.942151717890134290E-15 ) ) ;
#6609=CARTESIAN_POINT ( 'NONE',  ( 67.57499999726881867, 164.1591823560292198, -12.60653300113719766 ) ) ;
#6618=CARTESIAN_POINT ( 'NONE',  ( 70.91132485994280898, 146.1832212156128890, 12.13525491562421976 ) ) ;
#6623=CARTESIAN_POINT ( 'NONE',  ( 46.12499999726880873, 155.0000000000000000, 15.58253174999999402 ) ) ;
#6625=CARTESIAN_POINT ( 'NONE',  ( 87.50000000000004263, 150.3648420706765592, -14.53435407936543200 ) ) ;
#6632=CARTESIAN_POINT ( 'NONE',  ( 33.24999999726880873, 155.0000000000000000, -15.58253175000000823 ) ) ;
#6635=CARTESIAN_POINT ( 'NONE',  ( 64.09999999453764019, 159.7113355953771077, -14.50000000000000888 ) ) ;
#6636=VECTOR ( 'NONE', #20990, 1000.000000000000000 ) ;
#6640=EDGE_CURVE ( 'NONE', #29364, #22604, #30553, .T. ) ;
#6642=DIRECTION ( 'NONE',  ( 1.000000000000000000, 0.000000000000000000, 0.000000000000000000 ) ) ;
#6643=ORIENTED_EDGE ( 'NONE', *, *, #9825, .F. ) ;
#6650=CARTESIAN_POINT ( 'NONE',  ( 85.61132485994281183, 150.1262045565064227, -15.00000000000002665 ) ) ;
#6652=CARTESIAN_POINT ( 'NONE',  ( 53.37499999726881583, 155.0000000000000000, -15.58253175000000823 ) ) ;
#6660=CARTESIAN_POINT ( 'NONE',  ( 60.17499999726881299, 164.1591823560292198, 12.60653300113718167 ) ) ;
#6663=EDGE_CURVE ( 'NONE', #3719, #5223, #9300, .T. ) ;
#6664=EDGE_CURVE ( 'NONE', #25327, #7152, #16963, .T. ) ;
#6667=CARTESIAN_POINT ( 'NONE',  ( 77.59999999999999432, 150.2886644046228639, 14.49999999999999645 ) ) ;
#6672=CARTESIAN_POINT ( 'NONE',  ( 45.67499999726881299, 168.2552932293087906, -9.630534252274385310 ) ) ;
#6675=CARTESIAN_POINT ( 'NONE',  ( 85.62499999726880162, 171.3844434931184253, -7.942151717890132712E-15 ) ) ;
#6679=CARTESIAN_POINT ( 'NONE',  ( 47.79999999453762882, 146.4771138417591203, -11.73074641843674470 ) ) ;
#6685=ORIENTED_EDGE ( 'NONE', *, *, #31152, .F. ) ;
#6699=EDGE_LOOP ( 'NONE', ( #20691, #17591, #7058, #2558 ) ) ;
#6700=CARTESIAN_POINT ( 'NONE',  ( 38.52499999726881441, 140.1801316387863778, 4.815267126137185549 ) ) ;
#6705=CARTESIAN_POINT ( 'NONE',  ( 38.07499999726880446, 168.2552932293087906, 9.630534252274372875 ) ) ;
#6709=CARTESIAN_POINT ( 'NONE',  ( 63.10000000000000142, 168.7903194862797420, 4.480746418436729606 ) ) ;
#6713=AXIS2_PLACEMENT_3D ( 'NONE', #5681, #2641, #10645 ) ;
#6714=DIRECTION ( 'NONE',  ( 1.000000000000000000, 0.000000000000000000, 0.000000000000000000 ) ) ;
#6716=CARTESIAN_POINT ( 'NONE',  ( 66.82499999726881867, 141.7447067706911810, -9.630534252274385310 ) ) ;
#6720=CARTESIAN_POINT ( 'NONE',  ( 81.67499999726881299, 168.2552932293087906, -9.630534252274385310 ) ) ;
#6722=CARTESIAN_POINT ( 'NONE',  ( 72.28867513459482552, 139.2280666364260071, -4.041636747397287284E-15 ) ) ;
#6730=CARTESIAN_POINT ( 'NONE',  ( 66.38867513459483405, 140.7341522555726669, -4.635254915624220651 ) ) ;
#6732=CARTESIAN_POINT ( 'NONE',  ( 39.61132485994280472, 150.1262045565063943, -15.00000000000000355 ) ) ;
#6738=CARTESIAN_POINT ( 'NONE',  ( 85.72499999726882436, 169.8198683612136222, 4.815267126137181997 ) ) ;
#6739=ORIENTED_EDGE ( 'NONE', *, *, #16983, .F. ) ;
#6740=CARTESIAN_POINT ( 'NONE',  ( 69.51132485994280330, 146.1832212156128890, -12.13525491562423042 ) ) ;
#6741=CARTESIAN_POINT ( 'NONE',  ( 76.92499999726881299, 145.8408176439707802, -12.60653300113719588 ) ) ;
#6742=DIRECTION ( 'NONE',  ( 0.000000000000000000, 1.000000000000000000, -6.454785026890489601E-15 ) ) ;
#6746=CARTESIAN_POINT ( 'NONE',  ( 44.70000000000000284, 163.5228861582408797, -11.73074641843674470 ) ) ;
#6749=CARTESIAN_POINT ( 'NONE',  ( 73.31132485994281467, 140.7341522555726669, -4.635254915624220651 ) ) ;
#6752=CARTESIAN_POINT ( 'NONE',  ( 49.42499999726880588, 168.2552932293087906, -9.630534252274387086 ) ) ;
#6753=CARTESIAN_POINT ( 'NONE',  ( 65.97499999726881015, 169.8198683612136222, 4.815267126137181997 ) ) ;
#6754=( BOUNDED_CURVE ( )  B_SPLINE_CURVE ( 2, ( #25739, #10746, #10422, #10087, #28635, #10259, #20794, #31525, #18412, #20464, #31358 ),
 .UNSPECIFIED., .F., .T. ) 
 B_SPLINE_CURVE_WITH_KNOTS ( ( 3, 2, 2, 2, 2, 3 ),
 ( 0.4107142857142855874, 0.4142857142857141461, 0.4178571428571427049, 0.4214285714285713191, 0.4249999999999998779, 0.4285714285714284366 ),
 .UNSPECIFIED. ) 
 CURVE ( )  GEOMETRIC_REPRESENTATION_ITEM ( )  RATIONAL_B_SPLINE_CURVE ( ( 1.000000000000001554, 0.9510565162951518658, 1.000000000000000000, 0.9510565162951534202, 1.000000000000000000, 0.9510565162951534202, 1.000000000000000000, 0.9510565162951534202, 1.000000000000000000, 0.9510565162951541973, 0.9999999999999992228 ) ) 
 REPRESENTATION_ITEM ( '' )  );
#6759=EDGE_CURVE ( 'NONE', #317, #17109, #11356, .T. ) ;
#6763=CARTESIAN_POINT ( 'NONE',  ( 88.29999999453762882, 167.3344367211045096, -8.961492836873482304 ) ) ;
#6772=CARTESIAN_POINT ( 'NONE',  ( 69.07499999726881867, 141.7447067706911810, -9.630534252274385310 ) ) ;
#6775=CARTESIAN_POINT ( 'NONE',  ( 82.87499999726880162, 138.6155565068815747, -3.929120461958505118E-15 ) ) ;
#6776=FACE_OUTER_BOUND ( 'NONE', #8694, .T. ) ;
#6788=CARTESIAN_POINT ( 'NONE',  ( 38.31132485994280756, 169.2658477444273331, 4.635254915624208216 ) ) ;
#6791=CARTESIAN_POINT ( 'NONE',  ( 47.02499999726881441, 149.9369285172503510, -15.58253175000000823 ) ) ;
#6797=EDGE_CURVE ( 'NONE', #8990, #8808, #7277, .T. ) ;
#6803=CARTESIAN_POINT ( 'NONE',  ( 68.29999999453761461, 167.3344367211045096, -8.961492836873482304 ) ) ;
#6815=DIRECTION ( 'NONE',  ( 0.000000000000000000, 0.000000000000000000, -1.000000000000000000 ) ) ;
#6819=DIRECTION ( 'NONE',  ( -1.000000000000000000, -0.000000000000000000, -0.000000000000000000 ) ) ;
#6822=CARTESIAN_POINT ( 'NONE',  ( 59.07499999726880446, 141.7447067706911810, -9.630534252274387086 ) ) ;
#6829=CARTESIAN_POINT ( 'NONE',  ( 61.07499999726881867, 141.7447067706911810, -9.630534252274385310 ) ) ;
#6834=CARTESIAN_POINT ( 'NONE',  ( 79.50000000000000000, 155.0000000000000000, 14.49999999999999467 ) ) ;
#6836=DIRECTION ( 'NONE',  ( 1.000000000000000000, 0.000000000000000000, 0.000000000000000000 ) ) ;
#6839=CARTESIAN_POINT ( 'NONE',  ( 44.67499999726881299, 141.7447067706911810, 9.630534252274376428 ) ) ;
#6841=CARTESIAN_POINT ( 'NONE',  ( 85.72499999726882436, 169.8198683612136222, 4.815267126137181997 ) ) ;
#6842=CARTESIAN_POINT ( 'NONE',  ( 125.5000000000000000, 261.0000000000000000, 2.149999999999985256 ) ) ;
#6844=CARTESIAN_POINT ( 'NONE',  ( 49.79999999453762882, 146.4771138417591203, -11.73074641843674470 ) ) ;
#6847=CARTESIAN_POINT ( 'NONE',  ( 32.50000000000000000, 155.0000000000000000, -6.938893903907228378E-15 ) ) ;
#6848=FACE_OUTER_BOUND ( 'NONE', #11014, .T. ) ;
#6849=ORIENTED_EDGE ( 'NONE', *, *, #32692, .F. ) ;
#6860=AXIS2_PLACEMENT_3D ( 'NONE', #22595, #25321, #7618 ) ;
#6863=ORIENTED_EDGE ( 'NONE', *, *, #13724, .F. ) ;
#6864=CARTESIAN_POINT ( 'NONE',  ( 43.92499999726881299, 164.1591823560292198, 12.60653300113718167 ) ) ;
#6869=CARTESIAN_POINT ( 'NONE',  ( 41.47499999726880304, 160.0630714827496206, -15.58253175000000823 ) ) ;
#6873=CARTESIAN_POINT ( 'NONE',  ( 59.79999999999999716, 142.6655632788954620, 8.961492836873471646 ) ) ;
#6876=CARTESIAN_POINT ( 'NONE',  ( 32.50000000000000000, 155.0000000000000000, -6.938893903907228378E-15 ) ) ;
#6879=CARTESIAN_POINT ( 'NONE',  ( 62.82499999726881867, 141.7447067706911810, -9.630534252274385310 ) ) ;
#6881=ORIENTED_EDGE ( 'NONE', *, *, #27020, .T. ) ;
#6883=CARTESIAN_POINT ( 'NONE',  ( 81.07499999726880446, 141.7447067706911810, -9.630534252274385310 ) ) ;
#6904=CARTESIAN_POINT ( 'NONE',  ( 81.22499999726881015, 160.0630714827496206, -15.58253175000000823 ) ) ;
#6905=ORIENTED_EDGE ( 'NONE', *, *, #19495, .T. ) ;
#6908=CARTESIAN_POINT ( 'NONE',  ( 76.82499999726881867, 141.7447067706911810, -9.630534252274385310 ) ) ;
#6909=CARTESIAN_POINT ( 'NONE',  ( 63.71132485994279904, 155.0000000000000000, -15.00000000000002487 ) ) ;
#6911=CARTESIAN_POINT ( 'NONE',  ( 127.5000000000000000, 155.0000000000000000, 98.00000000000000000 ) ) ;
#6914=CARTESIAN_POINT ( 'NONE',  ( 42.60000000000000142, 159.7113355953771077, -14.50000000000000888 ) ) ;
#6917=FACE_OUTER_BOUND ( 'NONE', #26797, .T. ) ;
#6920=CARTESIAN_POINT ( 'NONE',  ( 47.92499999726881299, 164.1591823560292198, 12.60653300113718167 ) ) ;
#6921=CARTESIAN_POINT ( 'NONE',  ( 64.57499999726881867, 145.8408176439707802, 12.60653300113718345 ) ) ;
#6930=LINE ( 'NONE', #16687, #30055 ) ;
#6936=VERTEX_POINT ( 'NONE', #15258 ) ;
#6941=CARTESIAN_POINT ( 'NONE',  ( 72.67499999726881299, 141.7447067706911810, 9.630534252274376428 ) ) ;
#6945=CARTESIAN_POINT ( 'NONE',  ( 81.47499999726879594, 160.0630714827496206, -15.58253175000000823 ) ) ;
#6948=CARTESIAN_POINT ( 'NONE',  ( 59.22499999726879594, 160.0630714827496206, -15.58253175000000823 ) ) ;
#6961=CARTESIAN_POINT ( 'NONE',  ( 70.81132485994281467, 150.1262045565064227, 15.00000000000001599 ) ) ;
#6962=VECTOR ( 'NONE', #15321, 1000.000000000000000 ) ;
#6966=CARTESIAN_POINT ( 'NONE',  ( 45.42499999726879878, 168.2552932293087906, -9.630534252274385310 ) ) ;
#6973=VECTOR ( 'NONE', #25355, 1000.000000000000000 ) ;
#6975=CARTESIAN_POINT ( 'NONE',  ( 35.48867513459483547, 167.7597621252805880, 9.270509831248428867 ) ) ;
#6978=CARTESIAN_POINT ( 'NONE',  ( 72.39999999453763735, 168.7903194862797420, -4.480746418436745593 ) ) ;
#6983=CARTESIAN_POINT ( 'NONE',  ( 76.51132485994280330, 163.8167787843871110, 12.13525491562421621 ) ) ;
#6986=EDGE_LOOP ( 'NONE', ( #2282, #30319, #13558, #8732 ) ) ;
#6993=CARTESIAN_POINT ( 'NONE',  ( 85.21132485994283456, 139.2280666364260071, -4.041636747397287284E-15 ) ) ;
#6996=CARTESIAN_POINT ( 'NONE',  ( 54.17499999726881299, 164.1591823560292198, 12.60653300113718167 ) ) ;
#7000=DIRECTION ( 'NONE',  ( 0.000000000000000000, 0.000000000000000000, -1.000000000000000000 ) ) ;
#7001=CARTESIAN_POINT ( 'NONE',  ( 57.61132485994281183, 150.1262045565064227, -15.00000000000002665 ) ) ;
#7003=CARTESIAN_POINT ( 'NONE',  ( 64.77499999726882152, 140.1801316387863778, 4.815267126137185549 ) ) ;
#7007=CARTESIAN_POINT ( 'NONE',  ( 82.60000000000002274, 159.7113355953771077, -14.50000000000000888 ) ) ;
#7011=CARTESIAN_POINT ( 'NONE',  ( 48.78867513459482552, 155.0000000000000000, -15.00000000000002487 ) ) ;
#7012=CARTESIAN_POINT ( 'NONE',  ( 50.87499999726881583, 138.6155565068815463, -3.929120461958505118E-15 ) ) ;
#7014=CARTESIAN_POINT ( 'NONE',  ( 81.82499999726879025, 168.2552932293087906, 9.630534252274372875 ) ) ;
#7016=CARTESIAN_POINT ( 'NONE',  ( 51.71132485994281325, 155.0000000000000000, -15.00000000000002487 ) ) ;
#7017=ADVANCED_FACE ( 'NONE', ( #8586 ), #19140, .F. ) ;
#7018=DIRECTION ( 'NONE',  ( 1.000000000000000000, 0.000000000000000000, 0.000000000000000000 ) ) ;
#7019=CARTESIAN_POINT ( 'NONE',  ( 46.19999999453763451, 163.5228861582408797, -11.73074641843674470 ) ) ;
#7020=VERTEX_POINT ( 'NONE', #23436 ) ;
#7022=CARTESIAN_POINT ( 'NONE',  ( 61.31132485994281467, 140.7341522555726669, -4.635254915624220651 ) ) ;
#7031=DIRECTION ( 'NONE',  ( -1.000000000000000000, -0.000000000000000000, -0.000000000000000000 ) ) ;
#7038=CARTESIAN_POINT ( 'NONE',  ( 40.57499999726881157, 145.8408176439707802, 12.60653300113718345 ) ) ;
#7039=EDGE_LOOP ( 'NONE', ( #11143, #4668 ) ) ;
#7040=CARTESIAN_POINT ( 'NONE',  ( 43.22499999726881015, 160.0630714827496206, -15.58253175000000823 ) ) ;
#7044=CARTESIAN_POINT ( 'NONE',  ( 47.27499999726880731, 149.9369285172503510, -15.58253175000000823 ) ) ;
#7045=CARTESIAN_POINT ( 'NONE',  ( 32.50000000000000000, 155.0000000000000000, 13.00000000000001066 ) ) ;
#7050=CARTESIAN_POINT ( 'NONE',  ( 60.20000000000000995, 142.6655632788954620, -8.961492836873480528 ) ) ;
#7056=CARTESIAN_POINT ( 'NONE',  ( 65.92499999726881299, 164.1591823560292198, 12.60653300113718167 ) ) ;
#7058=ORIENTED_EDGE ( 'NONE', *, *, #23044, .T. ) ;
#7060=CARTESIAN_POINT ( 'NONE',  ( 83.87499999726878741, 171.3844434931184253, -7.942151717890132712E-15 ) ) ;
#7080=ORIENTED_EDGE ( 'NONE', *, *, #822, .F. ) ;
#7082=CARTESIAN_POINT ( 'NONE',  ( 77.82499999726880446, 168.2552932293087906, 9.630534252274372875 ) ) ;
#7083=CARTESIAN_POINT ( 'NONE',  ( 125.5000000000000000, 154.9999999999996305, -106.0000000000000142 ) ) ;
#7087=CARTESIAN_POINT ( 'NONE',  ( 40.00000000000000711, 139.7537977485451393, -4.138211985947621020E-15 ) ) ;
#7094=CARTESIAN_POINT ( 'NONE',  ( 51.32499999726881157, 164.1591823560292198, -12.60653300113719766 ) ) ;
#7095=CARTESIAN_POINT ( 'NONE',  ( 61.27499999726882152, 149.9369285172503510, -15.58253175000000823 ) ) ;
#7105=CARTESIAN_POINT ( 'NONE',  ( 83.71132485994282035, 155.0000000000000000, -15.00000000000002487 ) ) ;
#7109=CARTESIAN_POINT ( 'NONE',  ( 81.37499999726881583, 155.0000000000000000, -15.58253175000000823 ) ) ;
#7110=VERTEX_POINT ( 'NONE', #16087 ) ;
#7113=CARTESIAN_POINT ( 'NONE',  ( 80.67499999726881299, 141.7447067706911810, 9.630534252274376428 ) ) ;
#7116=CARTESIAN_POINT ( 'NONE',  ( 71.42499999726879878, 168.2552932293087906, -9.630534252274387086 ) ) ;
#7119=CARTESIAN_POINT ( 'NONE',  ( 59.72499999726881015, 169.8198683612136222, 4.815267126137181997 ) ) ;
#7120=CYLINDRICAL_SURFACE ( 'NONE', #4204, 2.149999999999985256 ) ;
#7122=ORIENTED_EDGE ( 'NONE', *, *, #26380, .F. ) ;
#7126=DIRECTION ( 'NONE',  ( -1.000000000000000000, -0.000000000000000000, 0.000000000000000000 ) ) ;
#7129=DIRECTION ( 'NONE',  ( -1.000000000000000000, -0.000000000000000000, -0.000000000000000000 ) ) ;
#7134=CARTESIAN_POINT ( 'NONE',  ( 53.22499999726879594, 160.0630714827496206, -15.58253175000000823 ) ) ;
#7146=CARTESIAN_POINT ( 'NONE',  ( 73.49999999453763166, 139.7537977485451393, -4.138211985947621020E-15 ) ) ;
#7152=VERTEX_POINT ( 'NONE', #21534 ) ;
#7155=DIRECTION ( 'NONE',  ( 0.000000000000000000, 0.000000000000000000, -1.000000000000000000 ) ) ;
#7159=( BOUNDED_CURVE ( )  B_SPLINE_CURVE ( 2, ( #7011, #12284, #22676, #9733, #7693, #15349, #13292, #2580, #30864, #12966, #28472 ),
 .UNSPECIFIED., .F., .T. ) 
 B_SPLINE_CURVE_WITH_KNOTS ( ( 3, 2, 2, 2, 2, 3 ),
 ( 0.6964285714285712858, 0.6999999999999998446, 0.7035714285714284033, 0.7071428571428569620, 0.7107142857142855208, 0.7142857142857140795 ),
 .UNSPECIFIED. ) 
 CURVE ( )  GEOMETRIC_REPRESENTATION_ITEM ( )  RATIONAL_B_SPLINE_CURVE ( ( 1.000000000000001554, 0.9510565162951518658, 1.000000000000000000, 0.9510565162951534202, 1.000000000000000000, 0.9510565162951534202, 1.000000000000000000, 0.9510565162951534202, 1.000000000000000000, 0.9510565162951549745, 0.9999999999999984457 ) ) 
 REPRESENTATION_ITEM ( '' )  );
#7162=CARTESIAN_POINT ( 'NONE',  ( 59.37499999726881583, 155.0000000000000000, -15.58253175000000823 ) ) ;
#7165=CARTESIAN_POINT ( 'NONE',  ( 67.21132485994282035, 139.2280666364260071, -4.041636747397287284E-15 ) ) ;
#7167=( NAMED_UNIT ( * ) SI_UNIT ( $, .STERADIAN. ) SOLID_ANGLE_UNIT ( ) );
#7170=CARTESIAN_POINT ( 'NONE',  ( 63.87499999726881583, 171.3844434931184253, -7.942151717890132712E-15 ) ) ;
#7175=AXIS2_PLACEMENT_3D ( 'NONE', #9420, #14526, #17423 ) ;
#7176=CARTESIAN_POINT ( 'NONE',  ( 78.70000000000000284, 163.5228861582408797, -11.73074641843674470 ) ) ;
#7181=CARTESIAN_POINT ( 'NONE',  ( 52.27499999726880020, 160.0630714827496206, 15.58253174999999402 ) ) ;
#7183=CARTESIAN_POINT ( 'NONE',  ( 81.62499999726878741, 171.3844434931184253, -7.942151717890132712E-15 ) ) ;
#7186=CARTESIAN_POINT ( 'NONE',  ( 54.29999999453762172, 167.3344367211045096, -8.961492836873482304 ) ) ;
#7189=CARTESIAN_POINT ( 'NONE',  ( 37.58867513459482268, 163.8167787843871110, 12.13525491562421621 ) ) ;
#7199=ORIENTED_EDGE ( 'NONE', *, *, #26031, .F. ) ;
#7204=CARTESIAN_POINT ( 'NONE',  ( 38.57499999726881157, 145.8408176439707802, 12.60653300113718345 ) ) ;
#7206=CARTESIAN_POINT ( 'NONE',  ( 43.42499999726881299, 168.2552932293087906, -9.630534252274385310 ) ) ;
#7207=CARTESIAN_POINT ( 'NONE',  ( 39.68867513459483121, 159.8737954434936057, 15.00000000000001421 ) ) ;
#7210=CARTESIAN_POINT ( 'NONE',  ( 48.67499999726881299, 141.7447067706911810, 9.630534252274376428 ) ) ;
#7215=CARTESIAN_POINT ( 'NONE',  ( 58.39999999999999858, 150.2886644046228639, -14.50000000000000888 ) ) ;
#7217=CARTESIAN_POINT ( 'NONE',  ( 125.5000000000000000, 48.99999999999998579, 2.149999999999971489 ) ) ;
#7220=CARTESIAN_POINT ( 'NONE',  ( 34.77499999726880731, 140.1801316387863778, 4.815267126137185549 ) ) ;
#7222=CARTESIAN_POINT ( 'NONE',  ( 64.02499999726880731, 160.0630714827496206, 15.58253174999999402 ) ) ;
#7227=CARTESIAN_POINT ( 'NONE',  ( 86.27499999726880731, 160.0630714827496206, 15.58253174999999402 ) ) ;
#7230=CARTESIAN_POINT ( 'NONE',  ( 125.5000000000000000, 80.04668119422662187, 74.95331880577468553 ) ) ;
#7231=ADVANCED_FACE ( 'NONE', ( #16418 ), #14040, .T. ) ;
#7240=AXIS2_PLACEMENT_3D ( 'NONE', #28131, #15184, #25577 ) ;
#7252=CARTESIAN_POINT ( 'NONE',  ( 73.77499999726882152, 169.8198683612136222, -4.815267126137197984 ) ) ;
#7253=CARTESIAN_POINT ( 'NONE',  ( 83.12499999726881583, 155.0000000000000000, -15.58253175000000823 ) ) ;
#7259=CARTESIAN_POINT ( 'NONE',  ( 45.00000000000000000, 170.2462022514548323, -7.872454543227099337E-15 ) ) ;
#7262=VECTOR ( 'NONE', #15307, 1000.000000000000000 ) ;
#7266=CARTESIAN_POINT ( 'NONE',  ( 59.72499999726881015, 169.8198683612136222, 4.815267126137181997 ) ) ;
#7267=CARTESIAN_POINT ( 'NONE',  ( 61.67499999726881299, 168.2552932293087906, -9.630534252274385310 ) ) ;
#7270=DIRECTION ( 'NONE',  ( 0.000000000000000000, 0.000000000000000000, -1.000000000000000000 ) ) ;
#7277=( BOUNDED_CURVE ( )  B_SPLINE_CURVE ( 2, ( #1633, #1468, #27358, #17647, #14581, #9470, #20199, #14744, #25137, #22413, #32803 ),
 .UNSPECIFIED., .F., .T. ) 
 B_SPLINE_CURVE_WITH_KNOTS ( ( 3, 2, 2, 2, 2, 3 ),
 ( 0.1607142857142858372, 0.1642857142857143127, 0.1678571428571427882, 0.1714285714285712636, 0.1749999999999997391, 0.1785714285714282146 ),
 .UNSPECIFIED. ) 
 CURVE ( )  GEOMETRIC_REPRESENTATION_ITEM ( )  RATIONAL_B_SPLINE_CURVE ( ( 0.9999999999999981126, 0.9510565162951553075, 1.000000000000000000, 0.9510565162951534202, 1.000000000000000000, 0.9510565162951534202, 1.000000000000000000, 0.9510565162951534202, 1.000000000000000000, 0.9510565162951571949, 0.9999999999999962252 ) ) 
 REPRESENTATION_ITEM ( '' )  );
#7281=AXIS2_PLACEMENT_3D ( 'NONE', #20311, #10441, #13474 ) ;
#7283=VECTOR ( 'NONE', #23533, 1000.000000000000000 ) ;
#7288=CARTESIAN_POINT ( 'NONE',  ( 75.27499999726879309, 149.9369285172503510, -15.58253175000000823 ) ) ;
#7293=CARTESIAN_POINT ( 'NONE',  ( 68.22499999726881015, 149.9369285172503510, 15.58253174999999580 ) ) ;
#7297=CARTESIAN_POINT ( 'NONE',  ( 65.02499999726882152, 149.9369285172503510, -15.58253175000000823 ) ) ;
#7298=EDGE_CURVE ( 'NONE', #11884, #32735, #30355, .T. ) ;
#7304=CARTESIAN_POINT ( 'NONE',  ( 127.5000000000000000, 155.0000000000000000, -6.938893903907228378E-15 ) ) ;
#7315=CARTESIAN_POINT ( 'NONE',  ( 40.62499999726880873, 138.6155565068815747, -3.929120461958505118E-15 ) ) ;
#7322=CARTESIAN_POINT ( 'NONE',  ( 35.18867513459482410, 169.2658477444273331, -4.635254915624224203 ) ) ;
#7325=CARTESIAN_POINT ( 'NONE',  ( 70.89999999453762314, 159.7113355953771077, 14.49999999999999289 ) ) ;
#7326=VERTEX_POINT ( 'NONE', #29045 ) ;
#7333=VERTEX_POINT ( 'NONE', #18655 ) ;
#7336=CYLINDRICAL_SURFACE ( 'NONE', #28221, 15.00000000000001776 ) ;
#7342=CARTESIAN_POINT ( 'NONE',  ( 55.97499999726881015, 169.8198683612136222, 4.815267126137181997 ) ) ;
#7343=VERTEX_POINT ( 'NONE', #27323 ) ;
#7348=CARTESIAN_POINT ( 'NONE',  ( 65.37499999726881583, 155.0000000000000000, -15.58253175000000823 ) ) ;
#7350=CARTESIAN_POINT ( 'NONE',  ( 70.68867513459485963, 150.1262045565065648, -15.00000000000016520 ) ) ;
#7354=CARTESIAN_POINT ( 'NONE',  ( 85.79999999999999716, 142.6655632788954620, 8.961492836873471646 ) ) ;
#7359=CARTESIAN_POINT ( 'NONE',  ( 49.47499999726881725, 160.0630714827496206, -15.58253175000000823 ) ) ;
#7361=CARTESIAN_POINT ( 'NONE',  ( 35.01132485994281041, 142.2402378747194405, 9.270509831248432420 ) ) ;
#7364=CARTESIAN_POINT ( 'NONE',  ( 54.39999999453763024, 168.7903194862797420, -4.480746418436745593 ) ) ;
#7365=ORIENTED_EDGE ( 'NONE', *, *, #31069, .T. ) ;
#7373=VERTEX_POINT ( 'NONE', #33117 ) ;
#7379=CARTESIAN_POINT ( 'NONE',  ( 38.97499999726881015, 140.1801316387863778, -4.815267126137194431 ) ) ;
#7381=CARTESIAN_POINT ( 'NONE',  ( 42.82499999726879736, 141.7447067706911810, -9.630534252274385310 ) ) ;
#7385=CARTESIAN_POINT ( 'NONE',  ( 49.27499999726880020, 149.9369285172503510, -15.58253175000000823 ) ) ;
#7389=CARTESIAN_POINT ( 'NONE',  ( 69.20000000000001705, 167.3344367211045096, 8.961492836873468093 ) ) ;
#7394=CARTESIAN_POINT ( 'NONE',  ( 87.50000000000001421, 155.0000000000000000, -6.938893903907228378E-15 ) ) ;
#7396=CARTESIAN_POINT ( 'NONE',  ( 66.02499999726879309, 160.0630714827496206, 15.58253174999999402 ) ) ;
#7399=CARTESIAN_POINT ( 'NONE',  ( 43.31132485994280756, 140.7341522555726669, -4.635254915624220651 ) ) ;
#7400=CARTESIAN_POINT ( 'NONE',  ( 35.19999999453762740, 146.4771138417591203, 11.73074641843673227 ) ) ;
#7402=DIRECTION ( 'NONE',  ( 1.000000000000000000, 0.000000000000000000, 0.000000000000000000 ) ) ;
#7412=CARTESIAN_POINT ( 'NONE',  ( 125.5000000000000000, 155.0000000000000000, 112.0000000000000426 ) ) ;
#7419=CARTESIAN_POINT ( 'NONE',  ( 81.02499999726880731, 149.9369285172503510, -15.58253175000000823 ) ) ;
#7421=( BOUNDED_CURVE ( )  B_SPLINE_CURVE ( 2, ( #21269, #27051, #656, #26710, #15993, #26541, #13933, #18724, #26385, #3045, #825 ),
 .UNSPECIFIED., .F., .T. ) 
 B_SPLINE_CURVE_WITH_KNOTS ( ( 3, 2, 2, 2, 2, 3 ),
 ( 0.4999999999999998890, 0.5035714285714285587, 0.5071428571428571175, 0.5107142857142856762, 0.5142857142857142350, 0.5178571428571427937 ),
 .UNSPECIFIED. ) 
 CURVE ( )  GEOMETRIC_REPRESENTATION_ITEM ( )  RATIONAL_B_SPLINE_CURVE ( ( 1.000000000000000666, 0.9510565162951526430, 1.000000000000000000, 0.9510565162951534202, 1.000000000000000000, 0.9510565162951534202, 1.000000000000000000, 0.9510565162951534202, 1.000000000000000000, 0.9510565162951534202, 1.000000000000000000 ) ) 
 REPRESENTATION_ITEM ( '' )  );
#7424=EDGE_CURVE ( 'NONE', #7326, #11207, #5921, .T. ) ;
#7425=CARTESIAN_POINT ( 'NONE',  ( 48.40000000000000568, 150.2886644046228639, -14.50000000000000888 ) ) ;
#7434=CARTESIAN_POINT ( 'NONE',  ( 57.02499999726882152, 149.9369285172503510, -15.58253175000000823 ) ) ;
#7435=CARTESIAN_POINT ( 'NONE',  ( 72.57499999726880446, 145.8408176439707802, 12.60653300113718345 ) ) ;
#7448=EDGE_LOOP ( 'NONE', ( #18051, #2303, #25121, #207 ) ) ;
#7452=CARTESIAN_POINT ( 'NONE',  ( 76.07499999726879025, 168.2552932293087906, 9.630534252274372875 ) ) ;
#7457=CARTESIAN_POINT ( 'NONE',  ( 71.82499999726881867, 168.2552932293087906, 9.630534252274372875 ) ) ;
#7460=CARTESIAN_POINT ( 'NONE',  ( 60.42499999726881299, 141.7447067706911810, 9.630534252274376428 ) ) ;
#7478=CARTESIAN_POINT ( 'NONE',  ( 39.32499999726881157, 164.1591823560292198, -12.60653300113719766 ) ) ;
#7479=( BOUNDED_CURVE ( )  B_SPLINE_CURVE ( 2, ( #23353, #31184, #23510, #10578, #5937, #24004, #16497, #3055, #29119, #16329, #26896 ),
 .UNSPECIFIED., .F., .F. ) 
 B_SPLINE_CURVE_WITH_KNOTS ( ( 3, 2, 2, 2, 2, 3 ),
 ( 0.8214285714285715079, 0.8250000000000000666, 0.8285714285714287364, 0.8321428571428572951, 0.8357142857142858539, 0.8392857142857144126 ),
 .UNSPECIFIED. ) 
 CURVE ( )  GEOMETRIC_REPRESENTATION_ITEM ( )  RATIONAL_B_SPLINE_CURVE ( ( 0.9999999999999984457, 0.9510565162951549745, 1.000000000000000000, 0.9510565162951534202, 1.000000000000000000, 0.9510565162951534202, 1.000000000000000000, 0.9510565162951534202, 1.000000000000000000, 0.9510565162951518658, 1.000000000000001554 ) ) 
 REPRESENTATION_ITEM ( '' )  );
#7482=TOROIDAL_SURFACE ( 'NONE', #26501, 70.00000000000001421, 30.00000000000000000 ) ;
#7490=CARTESIAN_POINT ( 'NONE',  ( 72.19999999453763451, 163.5228861582408797, -11.73074641843674470 ) ) ;
#7502=ORIENTED_EDGE ( 'NONE', *, *, #25531, .F. ) ;
#7510=CARTESIAN_POINT ( 'NONE',  ( 59.57499999726881157, 164.1591823560292198, -12.60653300113719766 ) ) ;
#7514=FILL_AREA_STYLE_COLOUR ( '', #23627 ) ;
#7517=CARTESIAN_POINT ( 'NONE',  ( 65.87499999726880162, 171.3844434931184253, -7.942151717890132712E-15 ) ) ;
#7520=CARTESIAN_POINT ( 'NONE',  ( 32.50000000000000000, 155.0000000000000000, -6.938893903907228378E-15 ) ) ;
#7521=CIRCLE ( 'NONE', #12960, 2.149999999999985256 ) ;
#7524=CARTESIAN_POINT ( 'NONE',  ( 83.80000000000002558, 142.6655632788954620, 8.961492836873471646 ) ) ;
#7529=CARTESIAN_POINT ( 'NONE',  ( 48.27499999726880731, 160.0630714827496206, 15.58253174999999402 ) ) ;
#7533=FACE_OUTER_BOUND ( 'NONE', #31859, .T. ) ;
#7534=CARTESIAN_POINT ( 'NONE',  ( 77.91132485994280898, 163.8167787843871110, -12.13525491562423397 ) ) ;
#7536=CARTESIAN_POINT ( 'NONE',  ( 55.19999999453763451, 146.4771138417591203, 11.73074641843673227 ) ) ;
#7539=EDGE_CURVE ( 'NONE', #31727, #24269, #16809, .T. ) ;
#7550=CARTESIAN_POINT ( 'NONE',  ( 80.78867513459482552, 155.0000000000000000, -15.00000000000002487 ) ) ;
#7554=CARTESIAN_POINT ( 'NONE',  ( 38.67499999726880588, 141.7447067706911810, 9.630534252274376428 ) ) ;
#7555=EDGE_LOOP ( 'NONE', ( #30664, #29064 ) ) ;
#7556=CARTESIAN_POINT ( 'NONE',  ( 43.72499999726881015, 169.8198683612136222, 4.815267126137181997 ) ) ;
#7561=CARTESIAN_POINT ( 'NONE',  ( 47.97499999726881015, 169.8198683612136222, 4.815267126137181997 ) ) ;
#7566=CARTESIAN_POINT ( 'NONE',  ( 65.29999999999999716, 163.5228861582408797, 11.73074641843673049 ) ) ;
#7574=CARTESIAN_POINT ( 'NONE',  ( 73.42499999726881299, 168.2552932293087906, -9.630534252274385310 ) ) ;
#7577=CARTESIAN_POINT ( 'NONE',  ( 36.19999999453762740, 163.5228861582408797, -11.73074641843674470 ) ) ;
#7584=AXIS2_PLACEMENT_3D ( 'NONE', #16928, #22046, #22214 ) ;
#7595=CARTESIAN_POINT ( 'NONE',  ( 33.81132485994280756, 159.8737954434936057, -15.00000000000002665 ) ) ;
#7596=VERTEX_POINT ( 'NONE', #20842 ) ;
#7599=CARTESIAN_POINT ( 'NONE',  ( 83.42499999726882720, 168.2552932293087906, -9.630534252274385310 ) ) ;
#7603=CARTESIAN_POINT ( 'NONE',  ( 47.20000000000000284, 167.3344367211045096, 8.961492836873468093 ) ) ;
#7606=CARTESIAN_POINT ( 'NONE',  ( 38.51132485994280330, 163.8167787843871110, 12.13525491562421621 ) ) ;
#7610=CARTESIAN_POINT ( 'NONE',  ( 59.42499999726880588, 168.2552932293087906, -9.630534252274387086 ) ) ;
#7611=CARTESIAN_POINT ( 'NONE',  ( 67.67499999726881299, 168.2552932293087906, -9.630534252274385310 ) ) ;
#7618=DIRECTION ( 'NONE',  ( 0.000000000000000000, 0.000000000000000000, -1.000000000000000000 ) ) ;
#7620=CARTESIAN_POINT ( 'NONE',  ( 68.31132485994278625, 169.2658477444273331, 4.635254915624208216 ) ) ;
#7628=CARTESIAN_POINT ( 'NONE',  ( 81.27499999726877888, 149.9369285172503510, -15.58253175000000823 ) ) ;
#7631=( BOUNDED_CURVE ( )  B_SPLINE_CURVE ( 2, ( #30758, #12528, #25640, #17463, #28370, #25815, #5192, #2306, #12860, #33477, #28023 ),
 .UNSPECIFIED., .F., .F. ) 
 B_SPLINE_CURVE_WITH_KNOTS ( ( 3, 2, 2, 2, 2, 3 ),
 ( 0.8392857142857144126, 0.8428571428571429713, 0.8464285714285715301, 0.8500000000000000888, 0.8535714285714286476, 0.8571428571428572063 ),
 .UNSPECIFIED. ) 
 CURVE ( )  GEOMETRIC_REPRESENTATION_ITEM ( )  RATIONAL_B_SPLINE_CURVE ( ( 0.9999999999999984457, 0.9510565162951549745, 1.000000000000000000, 0.9510565162951534202, 1.000000000000000000, 0.9510565162951534202, 1.000000000000000000, 0.9510565162951534202, 1.000000000000000000, 0.9510565162951518658, 1.000000000000001554 ) ) 
 REPRESENTATION_ITEM ( '' )  );
#7632=CARTESIAN_POINT ( 'NONE',  ( 73.92499999726881299, 164.1591823560292198, 12.60653300113718167 ) ) ;
#7635=CARTESIAN_POINT ( 'NONE',  ( 61.92499999726882010, 164.1591823560292198, 12.60653300113718167 ) ) ;
#7650=CARTESIAN_POINT ( 'NONE',  ( 40.42499999726881299, 141.7447067706911810, 9.630534252274376428 ) ) ;
#7658=CARTESIAN_POINT ( 'NONE',  ( 73.19999999453763451, 146.4771138417591203, 11.73074641843673227 ) ) ;
#7664=CARTESIAN_POINT ( 'NONE',  ( 75.71132485994280614, 155.0000000000000000, -15.00000000000002487 ) ) ;
#7665=ORIENTED_EDGE ( 'NONE', *, *, #28275, .T. ) ;
#7669=CARTESIAN_POINT ( 'NONE',  ( 32.50000000000000000, 155.0000000000000000, -6.938893903907228378E-15 ) ) ;
#7672=VERTEX_POINT ( 'NONE', #2629 ) ;
#7674=CARTESIAN_POINT ( 'NONE',  ( 44.78867513459481842, 155.0000000000000000, -15.00000000000002487 ) ) ;
#7676=CARTESIAN_POINT ( 'NONE',  ( 65.97499999726881015, 169.8198683612136222, 4.815267126137181997 ) ) ;
#7677=ORIENTED_EDGE ( 'NONE', *, *, #27899, .T. ) ;
#7689=CARTESIAN_POINT ( 'NONE',  ( 34.92499999726881299, 145.8408176439707802, -12.60653300113719588 ) ) ;
#7693=CARTESIAN_POINT ( 'NONE',  ( 48.38867513459482694, 140.7341522555726669, -4.635254915624220651 ) ) ;
#7694=CARTESIAN_POINT ( 'NONE',  ( 53.77499999726881441, 169.8198683612136222, -4.815267126137197984 ) ) ;
#7697=CARTESIAN_POINT ( 'NONE',  ( 34.81132485994281467, 150.1262045565062522, 14.99999999999989697 ) ) ;
#7700=CARTESIAN_POINT ( 'NONE',  ( 52.89999999453763024, 159.7113355953771077, 14.49999999999999289 ) ) ;
#7703=CARTESIAN_POINT ( 'NONE',  ( 46.91132485994280188, 146.1832212156128890, 12.13525491562421976 ) ) ;
#7711=CARTESIAN_POINT ( 'NONE',  ( 44.31132485994280046, 169.2658477444273331, 4.635254915624208216 ) ) ;
#7717=CARTESIAN_POINT ( 'NONE',  ( 45.27499999726880731, 149.9369285172503510, -15.58253175000000823 ) ) ;
#7719=CARTESIAN_POINT ( 'NONE',  ( 51.22499999726881015, 160.0630714827496206, -15.58253175000000823 ) ) ;
#7723=CARTESIAN_POINT ( 'NONE',  ( 46.77499999726881441, 140.1801316387863778, 4.815267126137185549 ) ) ;
#7728=CARTESIAN_POINT ( 'NONE',  ( 67.50000000000000000, 155.0000000000000000, 14.49999999999999467 ) ) ;
#7730=CARTESIAN_POINT ( 'NONE',  ( 38.78867513459481842, 155.0000000000000000, -15.00000000000002487 ) ) ;
#7736=CARTESIAN_POINT ( 'NONE',  ( 69.82499999726880446, 168.2552932293087906, 9.630534252274372875 ) ) ;
#7737=VERTEX_POINT ( 'NONE', #18788 ) ;
#7740=CARTESIAN_POINT ( 'NONE',  ( 86.37499999726881583, 155.0000000000000000, 15.58253174999999402 ) ) ;
#7743=ORIENTED_EDGE ( 'NONE', *, *, #15182, .F. ) ;
#7747=DIRECTION ( 'NONE',  ( 1.000000000000000000, 0.000000000000000000, 0.000000000000000000 ) ) ;
#7760=CARTESIAN_POINT ( 'NONE',  ( 84.52499999726880731, 140.1801316387863778, 4.815267126137185549 ) ) ;
#7766=CARTESIAN_POINT ( 'NONE',  ( 49.80000000000000426, 142.6655632788954620, 8.961492836873471646 ) ) ;
#7770=CARTESIAN_POINT ( 'NONE',  ( 53.52499999726881441, 169.8198683612136222, -4.815267126137197984 ) ) ;
#7771=LINE ( 'NONE', #5040, #5586 ) ;
#7773=CARTESIAN_POINT ( 'NONE',  ( 60.32499999726881157, 145.8408176439707802, 12.60653300113718345 ) ) ;
#7774=CARTESIAN_POINT ( 'NONE',  ( 67.77499999726880731, 169.8198683612136222, -4.815267126137197984 ) ) ;
#7786=VERTEX_POINT ( 'NONE', #29348 ) ;
#7790=ORIENTED_EDGE ( 'NONE', *, *, #30352, .T. ) ;
#7791=CARTESIAN_POINT ( 'NONE',  ( 76.27499999726877888, 160.0630714827496206, 15.58253174999999402 ) ) ;
#7794=CIRCLE ( 'NONE', #13755, 2.149999999999985256 ) ;
#7795=CARTESIAN_POINT ( 'NONE',  ( 69.22499999726881015, 160.0630714827496206, -15.58253175000000823 ) ) ;
#7798=CARTESIAN_POINT ( 'NONE',  ( 63.02499999726882152, 149.9369285172503510, -15.58253175000000823 ) ) ;
#7807=CARTESIAN_POINT ( 'NONE',  ( 44.98867513459482836, 163.8167787843871110, -12.13525491562423397 ) ) ;
#7815=CARTESIAN_POINT ( 'NONE',  ( 36.72499999726881015, 140.1801316387863778, -4.815267126137194431 ) ) ;
#7821=AXIS2_PLACEMENT_3D ( 'NONE', #1400, #27129, #1229 ) ;
#7825=CARTESIAN_POINT ( 'NONE',  ( 77.79999999453762882, 146.4771138417591203, -11.73074641843674470 ) ) ;
#7828=( BOUNDED_CURVE ( )  B_SPLINE_CURVE ( 2, ( #24196, #11252, #18758, #32030, #2923, #18915, #5789, #26252, #26920, #10602, #16185 ),
 .UNSPECIFIED., .F., .T. ) 
 B_SPLINE_CURVE_WITH_KNOTS ( ( 3, 2, 2, 2, 2, 3 ),
 ( 0.4464285714285713969, 0.4499999999999999556, 0.4535714285714285143, 0.4571428571428570731, 0.4607142857142856318, 0.4642857142857142461 ),
 .UNSPECIFIED. ) 
 CURVE ( )  GEOMETRIC_REPRESENTATION_ITEM ( )  RATIONAL_B_SPLINE_CURVE ( ( 1.000000000000000666, 0.9510565162951526430, 1.000000000000000000, 0.9510565162951534202, 1.000000000000000000, 0.9510565162951534202, 1.000000000000000000, 0.9510565162951534202, 1.000000000000000000, 0.9510565162951541973, 0.9999999999999992228 ) ) 
 REPRESENTATION_ITEM ( '' )  );
#7840=VECTOR ( 'NONE', #20784, 1000.000000000000000 ) ;
#7843=CARTESIAN_POINT ( 'NONE',  ( 82.41132485994280898, 167.7597621252805880, 9.270509831248428867 ) ) ;
#7845=CARTESIAN_POINT ( 'NONE',  ( 62.67499999726879878, 141.7447067706911810, 9.630534252274376428 ) ) ;
#7846=ORIENTED_EDGE ( 'NONE', *, *, #22042, .F. ) ;
#7847=CARTESIAN_POINT ( 'NONE',  ( 68.38867513459481984, 140.7341522555726669, -4.635254915624220651 ) ) ;
#7852=CARTESIAN_POINT ( 'NONE',  ( 36.71132485994280614, 155.0000000000000000, 15.00000000000001243 ) ) ;
#7853=EDGE_CURVE ( 'NONE', #4513, #3461, #23729, .T. ) ;
#7857=CARTESIAN_POINT ( 'NONE',  ( 35.22499999726881015, 160.0630714827496206, -15.58253175000000823 ) ) ;
#7862=CARTESIAN_POINT ( 'NONE',  ( 60.17499999726881299, 164.1591823560292198, 12.60653300113718167 ) ) ;
#7864=CYLINDRICAL_SURFACE ( 'NONE', #20831, 15.00000000000001776 ) ;
#7868=CARTESIAN_POINT ( 'NONE',  ( 51.89999999453762314, 150.2886644046228639, -14.50000000000000888 ) ) ;
#7887=CARTESIAN_POINT ( 'NONE',  ( 41.97499999726881015, 169.8198683612136222, 4.815267126137181997 ) ) ;
#7889=CARTESIAN_POINT ( 'NONE',  ( 52.12499999726881583, 155.0000000000000000, 15.58253174999999402 ) ) ;
#7893=CARTESIAN_POINT ( 'NONE',  ( 52.47499999726881015, 149.9369285172503510, 15.58253174999999580 ) ) ;
#7894=CARTESIAN_POINT ( 'NONE',  ( 79.51132485994280330, 146.1832212156128890, -12.13525491562423042 ) ) ;
#7896=DIRECTION ( 'NONE',  ( 1.000000000000000000, 0.000000000000000000, 0.000000000000000000 ) ) ;
#7898=CARTESIAN_POINT ( 'NONE',  ( 66.50000000000000000, 155.0000000000000000, -14.50000000000000711 ) ) ;
#7902=FACE_OUTER_BOUND ( 'NONE', #19210, .T. ) ;
#7903=CARTESIAN_POINT ( 'NONE',  ( 36.47499999726881015, 149.9369285172503510, 15.58253174999999580 ) ) ;
#7905=CARTESIAN_POINT ( 'NONE',  ( 71.52499999726882152, 169.8198683612136222, -4.815267126137197984 ) ) ;
#7908=CARTESIAN_POINT ( 'NONE',  ( 37.99999999453762456, 155.0000000000000000, -14.50000000000000711 ) ) ;
#7919=EDGE_CURVE ( 'NONE', #3834, #3719, #23594, .T. ) ;
#7922=ORIENTED_EDGE ( 'NONE', *, *, #23130, .F. ) ;
#7928=ORIENTED_EDGE ( 'NONE', *, *, #324, .T. ) ;
#7930=CARTESIAN_POINT ( 'NONE',  ( 86.52499999726882152, 140.1801316387863778, 4.815267126137185549 ) ) ;
#7935=CARTESIAN_POINT ( 'NONE',  ( 46.90000000000000568, 168.7903194862797420, -4.480746418436745593 ) ) ;
#7938=CARTESIAN_POINT ( 'NONE',  ( 48.72499999726881725, 140.1801316387863778, -4.815267126137194431 ) ) ;
#7941=CARTESIAN_POINT ( 'NONE',  ( 54.82499999726880446, 141.7447067706911810, -9.630534252274387086 ) ) ;
#7942=CARTESIAN_POINT ( 'NONE',  ( 68.37499999726881583, 155.0000000000000000, 15.58253174999999402 ) ) ;
#7944=CARTESIAN_POINT ( 'NONE',  ( 68.78867513459482552, 155.0000000000000000, -15.00000000000002487 ) ) ;
#7963=CARTESIAN_POINT ( 'NONE',  ( 77.22499999726881015, 160.0630714827496206, -15.58253175000000823 ) ) ;
#7967=CARTESIAN_POINT ( 'NONE',  ( 64.22499999726881015, 149.9369285172503510, 15.58253174999999580 ) ) ;
#7971=VERTEX_POINT ( 'NONE', #3610 ) ;
#7978=CARTESIAN_POINT ( 'NONE',  ( 63.58867513459481557, 163.8167787843871110, 12.13525491562421621 ) ) ;
#7983=DIRECTION ( 'NONE',  ( -1.000000000000000000, 0.000000000000000000, -0.000000000000000000 ) ) ;
#7985=CARTESIAN_POINT ( 'NONE',  ( 35.32499999726881157, 164.1591823560292198, -12.60653300113719766 ) ) ;
#7992=CARTESIAN_POINT ( 'NONE',  ( 81.39999999453763735, 141.2096805137202580, 4.480746418436733158 ) ) ;
#7996=AXIS2_PLACEMENT_3D ( 'NONE', #27970, #25585, #15527 ) ;
#8005=CARTESIAN_POINT ( 'NONE',  ( 51.48867513459483547, 167.7597621252805880, 9.270509831248428867 ) ) ;
#8010=CARTESIAN_POINT ( 'NONE',  ( 61.87499999726880162, 171.3844434931184253, -7.942151717890134290E-15 ) ) ;
#8019=VECTOR ( 'NONE', #20260, 1000.000000000000000 ) ;
#8023=CARTESIAN_POINT ( 'NONE',  ( 38.82499999726881157, 141.7447067706911810, -9.630534252274385310 ) ) ;
#8025=DIRECTION ( 'NONE',  ( 0.000000000000000000, 0.000000000000000000, -1.000000000000000000 ) ) ;
#8027=CARTESIAN_POINT ( 'NONE',  ( 83.71132485994282035, 155.0000000000000000, -15.00000000000002487 ) ) ;
#8028=CARTESIAN_POINT ( 'NONE',  ( 59.97499999726881015, 169.8198683612136222, 4.815267126137181997 ) ) ;
#8032=CARTESIAN_POINT ( 'NONE',  ( 127.5000000000000000, 157.1499999999996362, -106.0000000000000284 ) ) ;
#8034=CARTESIAN_POINT ( 'NONE',  ( 65.31132485994281467, 140.7341522555726669, -4.635254915624220651 ) ) ;
#8035=CARTESIAN_POINT ( 'NONE',  ( 60.29999999453761461, 167.3344367211045096, -8.961492836873482304 ) ) ;
#8038=CARTESIAN_POINT ( 'NONE',  ( 76.71132485994280614, 155.0000000000000000, 15.00000000000001243 ) ) ;
#8040=CARTESIAN_POINT ( 'NONE',  ( 71.78867513459482552, 155.0000000000000000, 15.00000000000001243 ) ) ;
#8044=VERTEX_POINT ( 'NONE', #11957 ) ;
#8053=CARTESIAN_POINT ( 'NONE',  ( 41.37499999726880873, 155.0000000000000000, -15.58253175000000823 ) ) ;
#8056=CARTESIAN_POINT ( 'NONE',  ( 53.42499999726879878, 168.2552932293087906, -9.630534252274385310 ) ) ;
#8060=CARTESIAN_POINT ( 'NONE',  ( 50.87499999726881583, 138.6155565068815463, -3.929120461958505118E-15 ) ) ;
#8064=CARTESIAN_POINT ( 'NONE',  ( 67.59999999999998010, 150.2886644046228639, 14.49999999999999645 ) ) ;
#8069=CARTESIAN_POINT ( 'NONE',  ( 86.08867513459483689, 142.2402378747194405, 9.270509831248432420 ) ) ;
#8070=CARTESIAN_POINT ( 'NONE',  ( 35.97499999726881015, 169.8198683612136222, 4.815267126137181997 ) ) ;
#8073=CARTESIAN_POINT ( 'NONE',  ( 69.72499999726881015, 169.8198683612136222, 4.815267126137181997 ) ) ;
#8075=CARTESIAN_POINT ( 'NONE',  ( 48.01132485994280330, 167.7597621252805880, -9.270509831248443078 ) ) ;
#8076=CARTESIAN_POINT ( 'NONE',  ( 38.19999999453763451, 163.5228861582408797, -11.73074641843674470 ) ) ;
#8080=AXIS2_PLACEMENT_3D ( 'NONE', #5990, #24222, #19281 ) ;
#8090=ORIENTED_EDGE ( 'NONE', *, *, #11237, .T. ) ;
#8097=CARTESIAN_POINT ( 'NONE',  ( 127.5000000000000000, 261.0000000000000000, 2.149999999999985256 ) ) ;
#8099=CARTESIAN_POINT ( 'NONE',  ( 86.42499999726881299, 141.7447067706911810, 9.630534252274376428 ) ) ;
#8104=CARTESIAN_POINT ( 'NONE',  ( 50.70000000000000284, 163.5228861582408797, -11.73074641843674470 ) ) ;
#8108=CARTESIAN_POINT ( 'NONE',  ( 49.52499999726880731, 169.8198683612136222, -4.815267126137197984 ) ) ;
#8112=CARTESIAN_POINT ( 'NONE',  ( 66.62499999726881583, 138.6155565068815747, -3.929120461958505118E-15 ) ) ;
#8113=CARTESIAN_POINT ( 'NONE',  ( 69.57499999726881867, 164.1591823560292198, -12.60653300113719766 ) ) ;
#8115=CARTESIAN_POINT ( 'NONE',  ( 49.41132485994282320, 142.2402378747194405, -9.270509831248439525 ) ) ;
#8118=CARTESIAN_POINT ( 'NONE',  ( 84.88867513459487668, 159.8737954434937478, -14.99999999999992362 ) ) ;
#8133=CARTESIAN_POINT ( 'NONE',  ( 77.82499999726880446, 168.2552932293087906, 9.630534252274372875 ) ) ;
#8137=CARTESIAN_POINT ( 'NONE',  ( 71.52499999726882152, 169.8198683612136222, -4.815267126137197984 ) ) ;
#8146=PLANE ( 'NONE',  #24550 ) ;
#8153=CARTESIAN_POINT ( 'NONE',  ( 44.82499999726880446, 141.7447067706911810, -9.630534252274387086 ) ) ;
#8161=CARTESIAN_POINT ( 'NONE',  ( 76.89999999453763735, 159.7113355953771077, 14.49999999999999289 ) ) ;
#8167=ORIENTED_EDGE ( 'NONE', *, *, #16367, .F. ) ;
#8170=ORIENTED_EDGE ( 'NONE', *, *, #28609, .F. ) ;
#8171=CARTESIAN_POINT ( 'NONE',  ( 78.17499999726881299, 164.1591823560292198, 12.60653300113718167 ) ) ;
#8173=CARTESIAN_POINT ( 'NONE',  ( 47.78867513459482552, 155.0000000000000000, 15.00000000000001243 ) ) ;
#8177=CARTESIAN_POINT ( 'NONE',  ( 65.47499999726881015, 160.0630714827496206, -15.58253175000000823 ) ) ;
#8178=EDGE_LOOP ( 'NONE', ( #1837, #29659, #17373, #33643 ) ) ;
#8179=CARTESIAN_POINT ( 'NONE',  ( 62.68867513459484542, 150.1262045565065364, -15.00000000000012434 ) ) ;
#8187=CARTESIAN_POINT ( 'NONE',  ( 86.37499999726881583, 155.0000000000000000, 15.58253174999999402 ) ) ;
#8190=CARTESIAN_POINT ( 'NONE',  ( 37.02499999726880020, 149.9369285172503510, -15.58253175000000823 ) ) ;
#8191=CARTESIAN_POINT ( 'NONE',  ( 35.78867513459482552, 155.0000000000000000, 15.00000000000001243 ) ) ;
#8192=CARTESIAN_POINT ( 'NONE',  ( 32.50000000000000000, 155.0000000000000000, -6.938893903907228378E-15 ) ) ;
#8195=CARTESIAN_POINT ( 'NONE',  ( 58.07499999726880446, 168.2552932293087906, 9.630534252274372875 ) ) ;
#8199=CARTESIAN_POINT ( 'NONE',  ( 55.28867513459483973, 170.7719333635740497, -7.904646289410545231E-15 ) ) ;
#8201=CARTESIAN_POINT ( 'NONE',  ( 57.49999999453763166, 139.7537977485451393, -4.138211985947621020E-15 ) ) ;
#8204=CYLINDRICAL_SURFACE ( 'NONE', #24684, 15.00000000000001776 ) ;
#8206=CARTESIAN_POINT ( 'NONE',  ( 70.98867513459484258, 163.8167787843871110, -12.13525491562423397 ) ) ;
#8215=CARTESIAN_POINT ( 'NONE',  ( 45.97499999726881015, 169.8198683612136222, 4.815267126137181997 ) ) ;
#8217=CARTESIAN_POINT ( 'NONE',  ( 49.82499999726881157, 168.2552932293087906, 9.630534252274372875 ) ) ;
#8221=CARTESIAN_POINT ( 'NONE',  ( 55.17499999726881299, 145.8408176439707802, -12.60653300113719588 ) ) ;
#8223=DIRECTION ( 'NONE',  ( 0.000000000000000000, -0.7071067811865506814, -0.7071067811865442421 ) ) ;
#8224=CARTESIAN_POINT ( 'NONE',  ( 73.00000000000001421, 170.2462022514548323, -7.872454543227099337E-15 ) ) ;
#8229=CARTESIAN_POINT ( 'NONE',  ( 40.87499999726880873, 138.6155565068815463, -3.929120461958505118E-15 ) ) ;
#8232=CARTESIAN_POINT ( 'NONE',  ( 68.72499999726881015, 140.1801316387863778, -4.815267126137194431 ) ) ;
#8235=CARTESIAN_POINT ( 'NONE',  ( 38.79999999453762882, 163.5228861582408797, 11.73074641843673049 ) ) ;
#8238=ORIENTED_EDGE ( 'NONE', *, *, #28899, .T. ) ;
#8253=CARTESIAN_POINT ( 'NONE',  ( 33.32499999726881157, 164.1591823560292198, -12.60653300113719766 ) ) ;
#8254=CARTESIAN_POINT ( 'NONE',  ( 87.72499999726882436, 169.8198683612136222, 4.815267126137181997 ) ) ;
#8259=CARTESIAN_POINT ( 'NONE',  ( 54.10000000000000142, 141.2096805137202580, -4.480746418436742040 ) ) ;
#8261=CARTESIAN_POINT ( 'NONE',  ( 84.51132485994280330, 163.8167787843871110, 12.13525491562421621 ) ) ;
#8262=EDGE_CURVE ( 'NONE', #26876, #23763, #32903, .T. ) ;
#8263=CARTESIAN_POINT ( 'NONE',  ( 50.82499999726880446, 141.7447067706911810, -9.630534252274385310 ) ) ;
#8268=CARTESIAN_POINT ( 'NONE',  ( 61.42499999726882010, 168.2552932293087906, -9.630534252274387086 ) ) ;
#8269=CARTESIAN_POINT ( 'NONE',  ( 78.77499999726880731, 140.1801316387863778, 4.815267126137185549 ) ) ;
#8272=EDGE_CURVE ( 'NONE', #33266, #12632, #22284, .T. ) ;
#8285=ORIENTED_EDGE ( 'NONE', *, *, #3345, .T. ) ;
#8288=EDGE_LOOP ( 'NONE', ( #3326, #25894, #8285, #9877 ) ) ;
#8290=CARTESIAN_POINT ( 'NONE',  ( 79.92499999726881299, 164.1591823560292198, 12.60653300113718167 ) ) ;
#8291=CYLINDRICAL_SURFACE ( 'NONE', #29310, 15.00000000000001776 ) ;
#8296=CARTESIAN_POINT ( 'NONE',  ( 71.72499999726881015, 169.8198683612136222, 4.815267126137181997 ) ) ;
#8309=CARTESIAN_POINT ( 'NONE',  ( 43.32499999726881157, 164.1591823560292198, -12.60653300113719766 ) ) ;
#8316=CARTESIAN_POINT ( 'NONE',  ( 77.89999999453763735, 150.2886644046228639, -14.50000000000000888 ) ) ;
#8323=CARTESIAN_POINT ( 'NONE',  ( 49.38867513459482694, 169.2658477444273331, 4.635254915624208216 ) ) ;
#8329=CARTESIAN_POINT ( 'NONE',  ( 74.97499999726881015, 140.1801316387863778, -4.815267126137194431 ) ) ;
#8337=CARTESIAN_POINT ( 'NONE',  ( 66.17499999726881299, 164.1591823560292198, 12.60653300113718167 ) ) ;
#8345=CARTESIAN_POINT ( 'NONE',  ( 83.58867513459483689, 163.8167787843871110, 12.13525491562421621 ) ) ;
#8347=CARTESIAN_POINT ( 'NONE',  ( 81.67499999726881299, 168.2552932293087906, -9.630534252274385310 ) ) ;
#8350=CARTESIAN_POINT ( 'NONE',  ( 38.02499999726881441, 160.0630714827496206, 15.58253174999999402 ) ) ;
#8354=CARTESIAN_POINT ( 'NONE',  ( 82.38867513459483405, 140.7341522555726669, -4.635254915624220651 ) ) ;
#8355=CARTESIAN_POINT ( 'NONE',  ( 58.87499999726880162, 138.6155565068815463, -3.929120461958505118E-15 ) ) ;
#8361=CARTESIAN_POINT ( 'NONE',  ( 62.79999999453762882, 163.5228861582408797, 11.73074641843673049 ) ) ;
#8362=ORIENTED_EDGE ( 'NONE', *, *, #5823, .F. ) ;
#8366=EDGE_CURVE ( 'NONE', #8954, #31727, #31642, .T. ) ;
#8367=ORIENTED_EDGE ( 'NONE', *, *, #11235, .F. ) ;
#8368=CIRCLE ( 'NONE', #21413, 30.00000000000000000 ) ;
#8369=( BOUNDED_CURVE ( )  B_SPLINE_CURVE ( 2, ( #8822, #5606, #15999, #3720, #21447, #1162, #31829, #21112, #8495, #29282, #5933 ),
 .UNSPECIFIED., .F., .F. ) 
 B_SPLINE_CURVE_WITH_KNOTS ( ( 3, 2, 2, 2, 2, 3 ),
 ( 0.8214285714285713969, 0.8249999999999999556, 0.8285714285714285143, 0.8321428571428570731, 0.8357142857142856318, 0.8392857142857141906 ),
 .UNSPECIFIED. ) 
 CURVE ( )  GEOMETRIC_REPRESENTATION_ITEM ( )  RATIONAL_B_SPLINE_CURVE ( ( 1.000000000000000000, 0.9510565162951534202, 1.000000000000000000, 0.9510565162951534202, 1.000000000000000000, 0.9510565162951534202, 1.000000000000000000, 0.9510565162951534202, 1.000000000000000000, 0.9510565162951534202, 1.000000000000000000 ) ) 
 REPRESENTATION_ITEM ( '' )  );
#8371=VECTOR ( 'NONE', #12478, 1000.000000000000000 ) ;
#8374=AXIS2_PLACEMENT_3D ( 'NONE', #16026, #13303, #18756 ) ;
#8381=CARTESIAN_POINT ( 'NONE',  ( 46.17499999726881299, 164.1591823560292198, 12.60653300113718167 ) ) ;
#8383=CARTESIAN_POINT ( 'NONE',  ( 50.02499999726880020, 160.0630714827496206, 15.58253174999999402 ) ) ;
#8387=CARTESIAN_POINT ( 'NONE',  ( 50.67499999726880588, 141.7447067706911810, 9.630534252274376428 ) ) ;
#8389=CARTESIAN_POINT ( 'NONE',  ( 47.18867513459482410, 169.2658477444273331, -4.635254915624224203 ) ) ;
#8391=CARTESIAN_POINT ( 'NONE',  ( 75.70000000000000284, 146.4771138417591203, 11.73074641843673227 ) ) ;
#8392=CARTESIAN_POINT ( 'NONE',  ( 62.11132485994280472, 169.2658477444273331, -4.635254915624224203 ) ) ;
#8393=DIRECTION ( 'NONE',  ( 1.000000000000000000, 0.000000000000000000, 0.000000000000000000 ) ) ;
#8397=CARTESIAN_POINT ( 'NONE',  ( 36.07499999726880446, 168.2552932293087906, 9.630534252274372875 ) ) ;
#8399=CARTESIAN_POINT ( 'NONE',  ( 74.12499999726881583, 155.0000000000000000, 15.58253174999999402 ) ) ;
#8402=CARTESIAN_POINT ( 'NONE',  ( 44.39999999453763024, 168.7903194862797420, -4.480746418436745593 ) ) ;
#8406=( GEOMETRIC_REPRESENTATION_CONTEXT ( 3 ) GLOBAL_UNCERTAINTY_ASSIGNED_CONTEXT ( ( #14795 ) ) GLOBAL_UNIT_ASSIGNED_CONTEXT ( ( #17725, #27944, #7167 ) ) REPRESENTATION_CONTEXT ( 'NONE', 'WORKASPACE' ) );
#8414=EDGE_LOOP ( 'NONE', ( #31093, #16234, #31622, #32687 ) ) ;
#8418=ORIENTED_EDGE ( 'NONE', *, *, #8366, .T. ) ;
#8420=CARTESIAN_POINT ( 'NONE',  ( 34.67499999726880588, 141.7447067706911810, 9.630534252274376428 ) ) ;
#8424=CARTESIAN_POINT ( 'NONE',  ( 55.30000000000000426, 163.5228861582408797, 11.73074641843673049 ) ) ;
#8427=CARTESIAN_POINT ( 'NONE',  ( 60.72499999726881015, 140.1801316387863778, -4.815267126137194431 ) ) ;
#8430=CARTESIAN_POINT ( 'NONE',  ( 32.50000000000000000, 155.0000000000000000, -6.938893903907228378E-15 ) ) ;
#8431=CARTESIAN_POINT ( 'NONE',  ( 61.32499999726881157, 164.1591823560292198, -12.60653300113719766 ) ) ;
#8432=CARTESIAN_POINT ( 'NONE',  ( 77.07499999726881867, 141.7447067706911810, -9.630534252274385310 ) ) ;
#8437=VERTEX_POINT ( 'NONE', #23020 ) ;
#8452=CARTESIAN_POINT ( 'NONE',  ( 80.92499999726882720, 145.8408176439707802, -12.60653300113719588 ) ) ;
#8454=DIRECTION ( 'NONE',  ( 0.5000000000000001110, 0.000000000000000000, 0.8660254037844385966 ) ) ;
#8455=CARTESIAN_POINT ( 'NONE',  ( 72.12499999726881583, 155.0000000000000000, 15.58253174999999402 ) ) ;
#8457=DIRECTION ( 'NONE',  ( 1.000000000000000000, 0.000000000000000000, 0.000000000000000000 ) ) ;
#8459=EDGE_CURVE ( 'NONE', #2009, #25327, #1594, .T. ) ;
#8460=CARTESIAN_POINT ( 'NONE',  ( 36.40000000000000568, 150.2886644046228639, -14.50000000000000888 ) ) ;
#8468=CARTESIAN_POINT ( 'NONE',  ( 42.62499999726881583, 138.6155565068815747, -3.929120461958505118E-15 ) ) ;
#8474=CARTESIAN_POINT ( 'NONE',  ( 81.59999999453762598, 141.2096805137202580, -4.480746418436742040 ) ) ;
#8486=CIRCLE ( 'NONE', #25369, 70.00000000000002842 ) ;
#8487=CARTESIAN_POINT ( 'NONE',  ( 76.47499999726881015, 149.9369285172503510, 15.58253174999999580 ) ) ;
#8488=CARTESIAN_POINT ( 'NONE',  ( 87.38867513459483405, 169.2658477444273331, 4.635254915624208216 ) ) ;
#8491=CARTESIAN_POINT ( 'NONE',  ( 32.50000000000000000, 155.0000000000000000, 15.00000000000001243 ) ) ;
#8493=CARTESIAN_POINT ( 'NONE',  ( 72.47499999726879594, 149.9369285172503510, 15.58253174999999580 ) ) ;
#8494=EDGE_LOOP ( 'NONE', ( #25927, #29907, #8776, #12592, #26213, #9621, #3922, #30363, #23000, #9037, #20055, #1323, #14481, #14807, #30873, #7922, #32906, #23821, #23212, #23249, #19722, #33253, #5917, #30755, #8767, #21101, #22648, #4215, #31331, #30757, #8167, #9703, #14954, #26612, #14901, #21314, #30666, #9569, #20021, #4925, #30528, #821, #24150, #2205, #14321, #21807, #22009, #20811, #2305, #33553, #5479, #1274, #8985, #20576, #27595, #12465, #15612 ) ) ;
#8495=CARTESIAN_POINT ( 'NONE',  ( 40.98867513459482126, 163.8167787843871110, -12.13525491562423397 ) ) ;
#8497=CARTESIAN_POINT ( 'NONE',  ( 42.88867513459482694, 159.8737954434936057, -15.00000000000002665 ) ) ;
#8502=CARTESIAN_POINT ( 'NONE',  ( 85.57499999726880446, 164.1591823560292198, -12.60653300113719766 ) ) ;
#8504=CARTESIAN_POINT ( 'NONE',  ( 36.72499999726881015, 140.1801316387863778, -4.815267126137194431 ) ) ;
#8508=CARTESIAN_POINT ( 'NONE',  ( 59.67499999726880588, 168.2552932293087906, -9.630534252274385310 ) ) ;
#8512=AXIS2_PLACEMENT_3D ( 'NONE', #31371, #8693, #5637 ) ;
#8517=CARTESIAN_POINT ( 'NONE',  ( 62.99999999453763166, 155.0000000000000000, 14.49999999999999467 ) ) ;
#8518=EDGE_LOOP ( 'NONE', ( #27416, #4308, #11147, #5435 ) ) ;
#8520=CARTESIAN_POINT ( 'NONE',  ( 77.71132485994280614, 155.0000000000000000, -15.00000000000002487 ) ) ;
#8523=VECTOR ( 'NONE', #2354, 1000.000000000000000 ) ;
#8524=ORIENTED_EDGE ( 'NONE', *, *, #32787, .F. ) ;
#8532=AXIS2_PLACEMENT_3D ( 'NONE', #18716, #21260, #29429 ) ;
#8534=CARTESIAN_POINT ( 'NONE',  ( 49.87499999726880873, 171.3844434931184253, -7.942151717890134290E-15 ) ) ;
#8536=CARTESIAN_POINT ( 'NONE',  ( 58.32499999726881157, 145.8408176439707802, 12.60653300113718345 ) ) ;
#8537=CARTESIAN_POINT ( 'NONE',  ( 32.50000000000000000, 155.0000000000000000, -15.00000000000002487 ) ) ;
#8542=CARTESIAN_POINT ( 'NONE',  ( 52.27499999726880020, 160.0630714827496206, 15.58253174999999402 ) ) ;
#8545=EDGE_CURVE ( 'NONE', #15361, #33178, #1397, .T. ) ;
#8549=CARTESIAN_POINT ( 'NONE',  ( 73.29999999999999716, 163.5228861582408797, 11.73074641843673049 ) ) ;
#8550=CARTESIAN_POINT ( 'NONE',  ( 62.31132485994281467, 169.2658477444273331, 4.635254915624208216 ) ) ;
#8551=CYLINDRICAL_SURFACE ( 'NONE', #32710, 112.0000000000000711 ) ;
#8554=CARTESIAN_POINT ( 'NONE',  ( 36.97499999726881015, 140.1801316387863778, -4.815267126137194431 ) ) ;
#8557=CARTESIAN_POINT ( 'NONE',  ( 76.12499999726881583, 155.0000000000000000, 15.58253174999999402 ) ) ;
#8560=CARTESIAN_POINT ( 'NONE',  ( 43.59999999453763309, 141.2096805137202580, -4.480746418436742040 ) ) ;
#8561=( BOUNDED_CURVE ( )  B_SPLINE_CURVE ( 2, ( #22242, #4524, #19686, #8958, #14574, #24635, #24464, #24975, #1628, #1126, #22404 ),
 .UNSPECIFIED., .F., .T. ) 
 B_SPLINE_CURVE_WITH_KNOTS ( ( 3, 2, 2, 2, 2, 3 ),
 ( 0.2142857142857139685, 0.2178571428571426383, 0.2214285714285711970, 0.2249999999999997280, 0.2285714285714282867, 0.2321428571428568455 ),
 .UNSPECIFIED. ) 
 CURVE ( )  GEOMETRIC_REPRESENTATION_ITEM ( )  RATIONAL_B_SPLINE_CURVE ( ( 1.000000000000003109, 0.9510565162951504226, 1.000000000000000000, 0.9510565162951534202, 1.000000000000000000, 0.9510565162951534202, 1.000000000000000000, 0.9510565162951534202, 1.000000000000000000, 0.9510565162951568619, 0.9999999999999965583 ) ) 
 REPRESENTATION_ITEM ( '' )  );
#8565=CARTESIAN_POINT ( 'NONE',  ( 40.51132485994280330, 163.8167787843871110, 12.13525491562421621 ) ) ;
#8583=CARTESIAN_POINT ( 'NONE',  ( 34.02499999726880731, 160.0630714827496206, 15.58253174999999402 ) ) ;
#8585=CARTESIAN_POINT ( 'NONE',  ( 86.82499999726879025, 141.7447067706911810, -9.630534252274385310 ) ) ;
#8586=FACE_OUTER_BOUND ( 'NONE', #2136, .T. ) ;
#8589=CARTESIAN_POINT ( 'NONE',  ( 54.59999999999999432, 159.7113355953771077, -14.50000000000000888 ) ) ;
#8591=CARTESIAN_POINT ( 'NONE',  ( 125.5000000000000000, 155.0000000000000000, -6.938893903907228378E-15 ) ) ;
#8593=CARTESIAN_POINT ( 'NONE',  ( 55.12499999726881583, 155.0000000000000000, -15.58253175000000823 ) ) ;
#8596=CARTESIAN_POINT ( 'NONE',  ( 60.92499999726882010, 145.8408176439707802, -12.60653300113719588 ) ) ;
#8597=CARTESIAN_POINT ( 'NONE',  ( 79.67499999726881299, 168.2552932293087906, -9.630534252274385310 ) ) ;
#8618=CARTESIAN_POINT ( 'NONE',  ( 79.12499999726881583, 155.0000000000000000, -15.58253175000000823 ) ) ;
#8621=CARTESIAN_POINT ( 'NONE',  ( 69.52499999726880731, 169.8198683612136222, -4.815267126137197984 ) ) ;
#8625=CARTESIAN_POINT ( 'NONE',  ( 36.19999999999999574, 142.6655632788954620, -8.961492836873480528 ) ) ;
#8631=AXIS2_PLACEMENT_3D ( 'NONE', #26761, #11272, #875 ) ;
#8636=CARTESIAN_POINT ( 'NONE',  ( 47.52499999726881441, 169.8198683612136222, -4.815267126137197984 ) ) ;
#8645=CARTESIAN_POINT ( 'NONE',  ( 88.59999999453762598, 168.7903194862797420, 4.480746418436729606 ) ) ;
#8656=CARTESIAN_POINT ( 'NONE',  ( 75.97499999726881015, 169.8198683612136222, 4.815267126137181997 ) ) ;
#8660=LINE ( 'NONE', #8491, #12339 ) ;
#8662=CARTESIAN_POINT ( 'NONE',  ( 71.67499999726881299, 168.2552932293087906, -9.630534252274387086 ) ) ;
#8664=CARTESIAN_POINT ( 'NONE',  ( 67.78867513459482552, 155.0000000000000000, 15.00000000000001243 ) ) ;
#8666=CARTESIAN_POINT ( 'NONE',  ( 42.78867513459481842, 155.0000000000000000, -15.00000000000002487 ) ) ;
#8671=CARTESIAN_POINT ( 'NONE',  ( 84.37499999726881583, 155.0000000000000000, 15.58253174999999402 ) ) ;
#8674=CARTESIAN_POINT ( 'NONE',  ( 40.62499999726880873, 138.6155565068815463, -3.929120461958505118E-15 ) ) ;
#8676=CARTESIAN_POINT ( 'NONE',  ( 125.5000000000000000, 155.0000000000000000, -6.938893903907228378E-15 ) ) ;
#8679=CARTESIAN_POINT ( 'NONE',  ( 60.77499999726881441, 140.1801316387863778, 4.815267126137185549 ) ) ;
#8684=CARTESIAN_POINT ( 'NONE',  ( 55.38867513459481984, 169.2658477444273331, 4.635254915624208216 ) ) ;
#8687=CARTESIAN_POINT ( 'NONE',  ( 57.99999999453763166, 155.0000000000000000, -14.50000000000000711 ) ) ;
#8691=CARTESIAN_POINT ( 'NONE',  ( 32.50000000000000000, 155.0000000000000000, -6.938893903907228378E-15 ) ) ;
#8693=DIRECTION ( 'NONE',  ( 1.000000000000000000, 0.000000000000000000, 0.000000000000000000 ) ) ;
#8694=EDGE_LOOP ( 'NONE', ( #9272, #24493, #28193, #7365 ) ) ;
#8695=EDGE_CURVE ( 'NONE', #8859, #30928, #5427, .T. ) ;
#8698=CARTESIAN_POINT ( 'NONE',  ( 50.01132485994283172, 167.7597621252805880, -9.270509831248443078 ) ) ;
#8703=( BOUNDED_CURVE ( )  B_SPLINE_CURVE ( 2, ( #2046, #163, #12597, #8005, #30669, #33556, #33390, #5438, #12435, #10564, #20441 ),
 .UNSPECIFIED., .F., .T. ) 
 B_SPLINE_CURVE_WITH_KNOTS ( ( 3, 2, 2, 2, 2, 3 ),
 ( 0.6428571428571426827, 0.6464285714285712414, 0.6499999999999998002, 0.6535714285714284699, 0.6571428571428570287, 0.6607142857142855874 ),
 .UNSPECIFIED. ) 
 CURVE ( )  GEOMETRIC_REPRESENTATION_ITEM ( )  RATIONAL_B_SPLINE_CURVE ( ( 1.000000000000001554, 0.9510565162951518658, 1.000000000000000000, 0.9510565162951534202, 1.000000000000000000, 0.9510565162951534202, 1.000000000000000000, 0.9510565162951534202, 1.000000000000000000, 0.9510565162951534202, 1.000000000000000000 ) ) 
 REPRESENTATION_ITEM ( '' )  );
#8706=CARTESIAN_POINT ( 'NONE',  ( 47.27499999726880731, 149.9369285172503510, -15.58253175000000823 ) ) ;
#8708=CARTESIAN_POINT ( 'NONE',  ( 54.22499999726881015, 149.9369285172503510, 15.58253174999999580 ) ) ;
#8714=CARTESIAN_POINT ( 'NONE',  ( 58.07499999726880446, 168.2552932293087906, 9.630534252274372875 ) ) ;
#8716=CARTESIAN_POINT ( 'NONE',  ( 72.78867513459482552, 155.0000000000000000, -15.00000000000002487 ) ) ;
#8718=CARTESIAN_POINT ( 'NONE',  ( 76.59999999999999432, 159.7113355953771077, -14.50000000000000888 ) ) ;
#8722=CARTESIAN_POINT ( 'NONE',  ( 33.38867513459482694, 169.2658477444273331, 4.635254915624208216 ) ) ;
#8723=CARTESIAN_POINT ( 'NONE',  ( 45.37499999726880873, 155.0000000000000000, -15.58253175000000823 ) ) ;
#8725=CARTESIAN_POINT ( 'NONE',  ( 78.82499999726881867, 141.7447067706911810, -9.630534252274385310 ) ) ;
#8728=CARTESIAN_POINT ( 'NONE',  ( 39.39999999453763024, 141.2096805137202580, 4.480746418436733158 ) ) ;
#8730=CARTESIAN_POINT ( 'NONE',  ( 40.01132485994281041, 167.7597621252805880, -9.270509831248443078 ) ) ;
#8732=ORIENTED_EDGE ( 'NONE', *, *, #31571, .F. ) ;
#8736=EDGE_LOOP ( 'NONE', ( #19997, #5391 ) ) ;
#8748=CARTESIAN_POINT ( 'NONE',  ( 39.72499999726881015, 169.8198683612136222, 4.815267126137181997 ) ) ;
#8751=CARTESIAN_POINT ( 'NONE',  ( 40.27499999726881441, 160.0630714827496206, 15.58253174999999402 ) ) ;
#8754=CARTESIAN_POINT ( 'NONE',  ( 54.20000000000000284, 142.6655632788954620, -8.961492836873480528 ) ) ;
#8757=CARTESIAN_POINT ( 'NONE',  ( 54.92499999726881299, 145.8408176439707802, -12.60653300113719588 ) ) ;
#8759=ORIENTED_EDGE ( 'NONE', *, *, #11483, .T. ) ;
#8762=CARTESIAN_POINT ( 'NONE',  ( 67.32499999726881867, 164.1591823560292198, -12.60653300113719766 ) ) ;
#8763=CARTESIAN_POINT ( 'NONE',  ( 75.47499999726881015, 160.0630714827496206, -15.58253175000000823 ) ) ;
#8766=CARTESIAN_POINT ( 'NONE',  ( 53.78867513459483263, 155.0000000000000000, 15.00000000000001243 ) ) ;
#8767=ORIENTED_EDGE ( 'NONE', *, *, #9576, .F. ) ;
#8776=ORIENTED_EDGE ( 'NONE', *, *, #6265, .T. ) ;
#8777=ORIENTED_EDGE ( 'NONE', *, *, #30012, .T. ) ;
#8781=CARTESIAN_POINT ( 'NONE',  ( 84.42499999726881299, 141.7447067706911810, 9.630534252274376428 ) ) ;
#8783=CARTESIAN_POINT ( 'NONE',  ( 69.38867513459481984, 169.2658477444273331, 4.635254915624208216 ) ) ;
#8785=CARTESIAN_POINT ( 'NONE',  ( 72.42499999726881299, 141.7447067706911810, 9.630534252274376428 ) ) ;
#8787=DIRECTION ( 'NONE',  ( 0.000000000000000000, 0.000000000000000000, -1.000000000000000000 ) ) ;
#8789=CARTESIAN_POINT ( 'NONE',  ( 32.99999999999999289, 170.2462022514548323, -7.872454543227099337E-15 ) ) ;
#8797=CARTESIAN_POINT ( 'NONE',  ( 47.42499999726880588, 168.2552932293087906, -9.630534252274387086 ) ) ;
#8804=CARTESIAN_POINT ( 'NONE',  ( 84.39999999453762314, 168.7903194862797420, -4.480746418436745593 ) ) ;
#8808=VERTEX_POINT ( 'NONE', #29639 ) ;
#8811=CARTESIAN_POINT ( 'NONE',  ( 72.57499999726880446, 145.8408176439707802, 12.60653300113718345 ) ) ;
#8813=ORIENTED_EDGE ( 'NONE', *, *, #13334, .F. ) ;
#8814=CARTESIAN_POINT ( 'NONE',  ( 74.87499999726880162, 138.6155565068815747, -3.929120461958505118E-15 ) ) ;
#8820=CARTESIAN_POINT ( 'NONE',  ( 68.97499999726881015, 140.1801316387863778, -4.815267126137194431 ) ) ;
#8822=CARTESIAN_POINT ( 'NONE',  ( 41.78867513459481842, 155.0000000000000000, 15.00000000000001243 ) ) ;
#8830=CARTESIAN_POINT ( 'NONE',  ( 82.27499999726880731, 160.0630714827496206, 15.58253174999999402 ) ) ;
#8834=CARTESIAN_POINT ( 'NONE',  ( 46.52499999726881441, 140.1801316387863778, 4.815267126137185549 ) ) ;
#8844=DIRECTION ( 'NONE',  ( 0.000000000000000000, 0.000000000000000000, -1.000000000000000000 ) ) ;
#8847=CARTESIAN_POINT ( 'NONE',  ( 66.19999999453763451, 163.5228861582408797, -11.73074641843674470 ) ) ;
#8851=CARTESIAN_POINT ( 'NONE',  ( 67.71132485994280614, 155.0000000000000000, -15.00000000000002487 ) ) ;
#8853=CARTESIAN_POINT ( 'NONE',  ( 45.31132485994280756, 140.7341522555726669, -4.635254915624220651 ) ) ;
#8857=DIRECTION ( 'NONE',  ( 0.000000000000000000, -1.000000000000000000, 6.454785026890489601E-15 ) ) ;
#8859=VERTEX_POINT ( 'NONE', #27244 ) ;
#8860=AXIS2_PLACEMENT_3D ( 'NONE', #4439, #17049, #12275 ) ;
#8863=LINE ( 'NONE', #19263, #29208 ) ;
#8864=EDGE_CURVE ( 'NONE', #8437, #28846, #11741, .T. ) ;
#8867=CARTESIAN_POINT ( 'NONE',  ( 47.67499999726881299, 168.2552932293087906, -9.630534252274387086 ) ) ;
#8868=VERTEX_POINT ( 'NONE', #9191 ) ;
#8869=CARTESIAN_POINT ( 'NONE',  ( 57.72499999726881015, 169.8198683612136222, 4.815267126137181997 ) ) ;
#8872=CARTESIAN_POINT ( 'NONE',  ( 0.000000000000000000, 0.000000000000000000, 0.000000000000000000 ) ) ;
#8875=CARTESIAN_POINT ( 'NONE',  ( 61.57499999726881157, 164.1591823560292198, -12.60653300113719766 ) ) ;
#8881=CARTESIAN_POINT ( 'NONE',  ( 75.00000000000000000, 170.2462022514548323, -7.872454543227099337E-15 ) ) ;
#8886=CARTESIAN_POINT ( 'NONE',  ( 45.07499999726880446, 141.7447067706911810, -9.630534252274385310 ) ) ;
#8888=CARTESIAN_POINT ( 'NONE',  ( 75.82499999726881867, 168.2552932293087906, 9.630534252274372875 ) ) ;
#8891=CARTESIAN_POINT ( 'NONE',  ( 50.49999999453762456, 170.2462022514548323, -7.872454543227099337E-15 ) ) ;
#8894=CARTESIAN_POINT ( 'NONE',  ( 40.61132485994281893, 159.8737954434936341, 14.99999999999998934 ) ) ;
#8914=CARTESIAN_POINT ( 'NONE',  ( 37.32499999726881157, 164.1591823560292198, -12.60653300113719766 ) ) ;
#8919=CARTESIAN_POINT ( 'NONE',  ( 41.87499999726880162, 171.3844434931184253, -7.942151717890132712E-15 ) ) ;
#8922=CARTESIAN_POINT ( 'NONE',  ( 55.60000000000000853, 150.2886644046228639, 14.49999999999999645 ) ) ;
#8927=EDGE_CURVE ( 'NONE', #18104, #10467, #20304, .T. ) ;
#8928=CARTESIAN_POINT ( 'NONE',  ( 58.62499999726880162, 138.6155565068815463, -3.929120461958505118E-15 ) ) ;
#8933=CARTESIAN_POINT ( 'NONE',  ( 80.07499999726879025, 168.2552932293087906, 9.630534252274372875 ) ) ;
#8938=VERTEX_POINT ( 'NONE', #275 ) ;
#8953=CARTESIAN_POINT ( 'NONE',  ( 82.12499999726881583, 155.0000000000000000, 15.58253174999999402 ) ) ;
#8954=VERTEX_POINT ( 'NONE', #9693 ) ;
#8956=CARTESIAN_POINT ( 'NONE',  ( 75.12499999726881583, 155.0000000000000000, -15.58253175000000823 ) ) ;
#8958=CARTESIAN_POINT ( 'NONE',  ( 75.48867513459482836, 167.7597621252805880, 9.270509831248428867 ) ) ;
#8960=CARTESIAN_POINT ( 'NONE',  ( 38.00000000000000711, 139.7537977485451393, -4.138211985947621020E-15 ) ) ;
#8965=EDGE_CURVE ( 'NONE', #30277, #31940, #3789, .T. ) ;
#8968=CYLINDRICAL_SURFACE ( 'NONE', #15876, 15.00000000000001776 ) ;
#8969=CARTESIAN_POINT ( 'NONE',  ( 52.12499999726881583, 155.0000000000000000, 15.58253174999999402 ) ) ;
#8975=EDGE_CURVE ( 'NONE', #33178, #33078, #4882, .T. ) ;
#8980=CARTESIAN_POINT ( 'NONE',  ( 86.29999999453764303, 167.3344367211045096, -8.961492836873482304 ) ) ;
#8985=ORIENTED_EDGE ( 'NONE', *, *, #18490, .F. ) ;
#8988=CARTESIAN_POINT ( 'NONE',  ( 74.07499999726880446, 168.2552932293087906, 9.630534252274372875 ) ) ;
#8990=VERTEX_POINT ( 'NONE', #15140 ) ;
#8991=CARTESIAN_POINT ( 'NONE',  ( 85.37499999726881583, 155.0000000000000000, -15.58253175000000823 ) ) ;
#8997=CARTESIAN_POINT ( 'NONE',  ( 67.27499999726879309, 149.9369285172503510, -15.58253175000000823 ) ) ;
#9000=LINE ( 'NONE', #378, #33555 ) ;
#9006=CARTESIAN_POINT ( 'NONE',  ( 38.21132485994280614, 170.7719333635740497, -7.904646289410545231E-15 ) ) ;
#9009=CARTESIAN_POINT ( 'NONE',  ( 47.72499999726881015, 169.8198683612136222, 4.815267126137181997 ) ) ;
#9011=CARTESIAN_POINT ( 'NONE',  ( 33.82499999726880446, 168.2552932293087906, 9.630534252274372875 ) ) ;
#9013=CARTESIAN_POINT ( 'NONE',  ( 82.68867513459481700, 150.1262045565064795, -15.00000000000009592 ) ) ;
#9021=CARTESIAN_POINT ( 'NONE',  ( 68.79999999453762882, 163.5228861582408797, 11.73074641843673049 ) ) ;
#9022=EDGE_LOOP ( 'NONE', ( #26538, #12636, #11622, #20941 ) ) ;
#9027=VERTEX_POINT ( 'NONE', #25190 ) ;
#9029=ORIENTED_EDGE ( 'NONE', *, *, #23556, .T. ) ;
#9030=CARTESIAN_POINT ( 'NONE',  ( 87.49999999999995737, 164.4872682688857708, -12.40341692595884027 ) ) ;
#9036=CARTESIAN_POINT ( 'NONE',  ( 52.47499999726881015, 149.9369285172503510, 15.58253174999999580 ) ) ;
#9037=ORIENTED_EDGE ( 'NONE', *, *, #629, .F. ) ;
#9038=CARTESIAN_POINT ( 'NONE',  ( 57.82499999726879736, 168.2552932293087906, 9.630534252274372875 ) ) ;
#9041=CARTESIAN_POINT ( 'NONE',  ( 117.5000000000000142, 155.0000000000000000, -6.938893903907228378E-15 ) ) ;
#9043=CARTESIAN_POINT ( 'NONE',  ( 63.07499999726881867, 141.7447067706911810, -9.630534252274385310 ) ) ;
#9045=CARTESIAN_POINT ( 'NONE',  ( 46.98867513459482836, 163.8167787843871110, -12.13525491562423397 ) ) ;
#9048=CARTESIAN_POINT ( 'NONE',  ( 82.79999999999999716, 167.3344367211045096, -8.961492836873482304 ) ) ;
#9049=CARTESIAN_POINT ( 'NONE',  ( 39.88867513459481984, 150.1262045565064227, 15.00000000000001599 ) ) ;
#9053=CARTESIAN_POINT ( 'NONE',  ( 43.67499999726881299, 168.2552932293087906, -9.630534252274385310 ) ) ;
#9055=CARTESIAN_POINT ( 'NONE',  ( 83.32499999726880446, 164.1591823560292198, -12.60653300113719766 ) ) ;
#9059=CARTESIAN_POINT ( 'NONE',  ( 48.69999999453762030, 167.3344367211045096, 8.961492836873468093 ) ) ;
#9079=CARTESIAN_POINT ( 'NONE',  ( 39.12499999726880873, 155.0000000000000000, -15.58253175000000823 ) ) ;
#9082=CARTESIAN_POINT ( 'NONE',  ( 43.47499999726881015, 160.0630714827496206, -15.58253175000000823 ) ) ;
#9083=FACE_OUTER_BOUND ( 'NONE', #24775, .T. ) ;
#9085=CARTESIAN_POINT ( 'NONE',  ( 58.59999999999999432, 159.7113355953771077, -14.50000000000000888 ) ) ;
#9086=DIRECTION ( 'NONE',  ( 0.000000000000000000, -0.7071067811865411334, 0.7071067811865540120 ) ) ;
#9089=DIRECTION ( 'NONE',  ( 0.000000000000000000, 0.000000000000000000, -1.000000000000000000 ) ) ;
#9092=CARTESIAN_POINT ( 'NONE',  ( 56.82499999726880446, 141.7447067706911810, -9.630534252274385310 ) ) ;
#9097=CARTESIAN_POINT ( 'NONE',  ( 81.77499999726880731, 169.8198683612136222, -4.815267126137197984 ) ) ;
#9113=VERTEX_POINT ( 'NONE', #14214 ) ;
#9118=AXIS2_PLACEMENT_3D ( 'NONE', #21479, #3582, #8857 ) ;
#9119=CARTESIAN_POINT ( 'NONE',  ( 83.42499999726882720, 168.2552932293087906, -9.630534252274387086 ) ) ;
#9122=CARTESIAN_POINT ( 'NONE',  ( 77.92499999726881299, 164.1591823560292198, 12.60653300113718167 ) ) ;
#9128=CARTESIAN_POINT ( 'NONE',  ( 37.20000000000000995, 167.3344367211045096, 8.961492836873468093 ) ) ;
#9135=CARTESIAN_POINT ( 'NONE',  ( 53.12499999726881583, 155.0000000000000000, -15.58253175000000823 ) ) ;
#9145=CARTESIAN_POINT ( 'NONE',  ( 86.09999999453764019, 159.7113355953771077, -14.50000000000000888 ) ) ;
#9154=CARTESIAN_POINT ( 'NONE',  ( 71.27499999726880731, 149.9369285172503510, -15.58253175000000823 ) ) ;
#9159=CARTESIAN_POINT ( 'NONE',  ( 83.17499999726882720, 145.8408176439707802, -12.60653300113719588 ) ) ;
#9165=CARTESIAN_POINT ( 'NONE',  ( 125.5000000000000000, 231.4735983853260279, 73.43303922622204993 ) ) ;
#9168=CARTESIAN_POINT ( 'NONE',  ( 72.07499999726879025, 168.2552932293087906, 9.630534252274372875 ) ) ;
#9183=CARTESIAN_POINT ( 'NONE',  ( 46.22499999726880304, 149.9369285172503510, 15.58253174999999580 ) ) ;
#9191=CARTESIAN_POINT ( 'NONE',  ( 46.71132485994281325, 155.0000000000000000, 15.00000000000001243 ) ) ;
#9194=CARTESIAN_POINT ( 'NONE',  ( 66.49999999453763166, 170.2462022514548323, -7.872454543227099337E-15 ) ) ;
#9200=CARTESIAN_POINT ( 'NONE',  ( 75.91132485994280898, 163.8167787843871110, -12.13525491562423397 ) ) ;
#9202=AXIS2_PLACEMENT_3D ( 'NONE', #14484, #24884, #1545 ) ;
#9203=CARTESIAN_POINT ( 'NONE',  ( 77.59999999453762598, 141.2096805137202580, -4.480746418436742040 ) ) ;
#9207=CARTESIAN_POINT ( 'NONE',  ( 125.5000000000000000, 48.99999999999998579, -1.387778780781445676E-14 ) ) ;
#9208=DIRECTION ( 'NONE',  ( 1.000000000000000000, 0.000000000000000000, 0.000000000000000000 ) ) ;
#9213=CARTESIAN_POINT ( 'NONE',  ( 51.27499999726880731, 149.9369285172503510, -15.58253175000000823 ) ) ;
#9220=CARTESIAN_POINT ( 'NONE',  ( 60.87499999726879452, 138.6155565068815463, -3.929120461958505118E-15 ) ) ;
#9225=CARTESIAN_POINT ( 'NONE',  ( 81.90000000000000568, 141.2096805137202580, 4.480746418436733158 ) ) ;
#9230=CARTESIAN_POINT ( 'NONE',  ( 43.57499999726881157, 164.1591823560292198, -12.60653300113719766 ) ) ;
#9232=CARTESIAN_POINT ( 'NONE',  ( 81.22499999726882436, 160.0630714827496206, -15.58253175000000823 ) ) ;
#9234=DIRECTION ( 'NONE',  ( 1.000000000000000000, 0.000000000000000000, 0.000000000000000000 ) ) ;
#9235=CARTESIAN_POINT ( 'NONE',  ( 47.39999999453763024, 141.2096805137202580, 4.480746418436733158 ) ) ;
#9238=CARTESIAN_POINT ( 'NONE',  ( 60.91132485994280898, 146.1832212156128890, 12.13525491562421976 ) ) ;
#9245=CYLINDRICAL_SURFACE ( 'NONE', #31751, 100.0000000000000000 ) ;
#9250=CARTESIAN_POINT ( 'NONE',  ( 33.87499999726880873, 171.3844434931184253, -7.942151717890134290E-15 ) ) ;
#9251=ORIENTED_EDGE ( 'NONE', *, *, #10224, .T. ) ;
#9252=CARTESIAN_POINT ( 'NONE',  ( 37.92499999726881299, 164.1591823560292198, 12.60653300113718167 ) ) ;
#9254=CARTESIAN_POINT ( 'NONE',  ( 53.71132485994279904, 155.0000000000000000, -15.00000000000002487 ) ) ;
#9256=CARTESIAN_POINT ( 'NONE',  ( 38.27499999726881441, 160.0630714827496206, 15.58253174999999402 ) ) ;
#9260=CARTESIAN_POINT ( 'NONE',  ( 64.10000000000000853, 141.2096805137202580, -4.480746418436742040 ) ) ;
#9265=CARTESIAN_POINT ( 'NONE',  ( 64.22499999726881015, 149.9369285172503510, 15.58253174999999580 ) ) ;
#9269=CARTESIAN_POINT ( 'NONE',  ( 85.97499999726882436, 169.8198683612136222, 4.815267126137181997 ) ) ;
#9272=ORIENTED_EDGE ( 'NONE', *, *, #324, .F. ) ;
#9277=DIRECTION ( 'NONE',  ( 1.000000000000000000, 0.000000000000000000, 0.000000000000000000 ) ) ;
#9286=CARTESIAN_POINT ( 'NONE',  ( 86.62499999726881583, 138.6155565068815747, -3.929120461958505118E-15 ) ) ;
#9289=CARTESIAN_POINT ( 'NONE',  ( 79.52499999726880731, 169.8198683612136222, -4.815267126137197984 ) ) ;
#9295=CARTESIAN_POINT ( 'NONE',  ( 43.30000000000000426, 163.5228861582408797, 11.73074641843673049 ) ) ;
#9297=EDGE_CURVE ( 'NONE', #10467, #24797, #3979, .T. ) ;
#9298=EDGE_CURVE ( 'NONE', #33078, #17976, #19010, .T. ) ;
#9300=LINE ( 'NONE', #19692, #24955 ) ;
#9301=CARTESIAN_POINT ( 'NONE',  ( 32.50000000000000000, 155.0000000000000000, -15.00000000000002487 ) ) ;
#9302=CARTESIAN_POINT ( 'NONE',  ( 52.22499999726881725, 149.9369285172503510, 15.58253174999999580 ) ) ;
#9303=CARTESIAN_POINT ( 'NONE',  ( 65.77499999726880731, 169.8198683612136222, -4.815267126137197984 ) ) ;
#9310=CARTESIAN_POINT ( 'NONE',  ( 87.19999999453763451, 146.4771138417591203, 11.73074641843673227 ) ) ;
#9319=VERTEX_POINT ( 'NONE', #21816 ) ;
#9320=CARTESIAN_POINT ( 'NONE',  ( 71.07499999726880446, 141.7447067706911810, -9.630534252274385310 ) ) ;
#9324=CARTESIAN_POINT ( 'NONE',  ( 81.57499999726880446, 164.1591823560292198, -12.60653300113719766 ) ) ;
#9333=CARTESIAN_POINT ( 'NONE',  ( 89.50000000000001421, 155.0000000000000000, -13.00000000000002487 ) ) ;
#9334=( BOUNDED_CURVE ( )  B_SPLINE_CURVE ( 2, ( #10668, #10993, #18659, #15928, #14345, #13541, #31447, #8115, #16892, #29855, #31604 ),
 .UNSPECIFIED., .F., .F. ) 
 B_SPLINE_CURVE_WITH_KNOTS ( ( 3, 2, 2, 2, 2, 3 ),
 ( 0.2678571428571428492, 0.2714285714285714080, 0.2750000000000000222, 0.2785714285714285809, 0.2821428571428571397, 0.2857142857142856984 ),
 .UNSPECIFIED. ) 
 CURVE ( )  GEOMETRIC_REPRESENTATION_ITEM ( )  RATIONAL_B_SPLINE_CURVE ( ( 1.000000000000000000, 0.9510565162951534202, 1.000000000000000000, 0.9510565162951534202, 1.000000000000000000, 0.9510565162951534202, 1.000000000000000000, 0.9510565162951534202, 1.000000000000000000, 0.9510565162951534202, 1.000000000000000000 ) ) 
 REPRESENTATION_ITEM ( '' )  );
#9342=CARTESIAN_POINT ( 'NONE',  ( 43.42499999726881299, 168.2552932293087906, -9.630534252274385310 ) ) ;
#9343=CARTESIAN_POINT ( 'NONE',  ( 87.50000000000001421, 147.9321341023432126, -13.35674708564858015 ) ) ;
#9353=CARTESIAN_POINT ( 'NONE',  ( 65.89999999453762314, 150.2886644046228639, -14.50000000000000888 ) ) ;
#9361=CARTESIAN_POINT ( 'NONE',  ( 76.21132485994282035, 170.7719333635740497, -7.904646289410545231E-15 ) ) ;
#9365=EDGE_LOOP ( 'NONE', ( #7502, #18839, #16239, #6084, #1870, #29008, #12527, #13312, #10938, #5541, #33543, #33429, #29833, #11724, #15393, #26125, #12298, #16778, #16949, #13713, #11286, #6160, #601, #25340, #3369, #2550, #22571, #32522, #27843, #17883, #21588, #8813, #27892, #14407, #26210, #8170, #16942, #661, #27002, #29566, #7122, #11047, #27758, #1571, #15872, #6739, #12639, #6849, #33474, #14907, #10443, #20362, #26381, #20308, #29860, #28330, #24613, #32742 ) ) ;
#9366=CARTESIAN_POINT ( 'NONE',  ( 42.08867513459482979, 142.2402378747194405, 9.270509831248432420 ) ) ;
#9369=ORIENTED_EDGE ( 'NONE', *, *, #22678, .T. ) ;
#9373=CARTESIAN_POINT ( 'NONE',  ( 58.57499999726881157, 145.8408176439707802, 12.60653300113718345 ) ) ;
#9379=CARTESIAN_POINT ( 'NONE',  ( 57.11132485994280472, 140.7341522555726669, 4.635254915624211769 ) ) ;
#9381=CARTESIAN_POINT ( 'NONE',  ( 62.07499999726881157, 168.2552932293087906, 9.630534252274372875 ) ) ;
#9383=CARTESIAN_POINT ( 'NONE',  ( 125.5000000000000000, 80.04668119422552763, -74.95331880577366235 ) ) ;
#9386=CARTESIAN_POINT ( 'NONE',  ( 80.10000000000000853, 141.2096805137202580, -4.480746418436742040 ) ) ;
#9391=CARTESIAN_POINT ( 'NONE',  ( 41.77499999726881441, 169.8198683612136222, -4.815267126137197984 ) ) ;
#9394=CARTESIAN_POINT ( 'NONE',  ( 84.62499999726880162, 138.6155565068815463, -3.929120461958505118E-15 ) ) ;
#9398=CARTESIAN_POINT ( 'NONE',  ( 48.99999999453763166, 155.0000000000000000, 14.49999999999999467 ) ) ;
#9401=EDGE_CURVE ( 'NONE', #18094, #9027, #22488, .T. ) ;
#9403=CARTESIAN_POINT ( 'NONE',  ( 61.21132485994281325, 139.2280666364260071, -4.041636747397287284E-15 ) ) ;
#9417=CYLINDRICAL_SURFACE ( 'NONE', #29847, 15.00000000000001776 ) ;
#9419=CARTESIAN_POINT ( 'NONE',  ( 35.32499999726881157, 164.1591823560292198, -12.60653300113719766 ) ) ;
#9420=CARTESIAN_POINT ( 'NONE',  ( 117.5000000000000142, 155.0000000000000000, -6.938893903907228378E-15 ) ) ;
#9424=CARTESIAN_POINT ( 'NONE',  ( 40.67499999726880588, 141.7447067706911810, 9.630534252274376428 ) ) ;
#9430=CARTESIAN_POINT ( 'NONE',  ( 61.19999999999999574, 167.3344367211045096, 8.961492836873468093 ) ) ;
#9431=DIRECTION ( 'NONE',  ( 1.000000000000000000, 0.000000000000000000, 0.000000000000000000 ) ) ;
#9438=CARTESIAN_POINT ( 'NONE',  ( 63.62499999726879452, 171.3844434931184253, -7.942151717890132712E-15 ) ) ;
#9442=CARTESIAN_POINT ( 'NONE',  ( 85.87499999726881583, 171.3844434931184253, -7.942151717890132712E-15 ) ) ;
#9445=ORIENTED_EDGE ( 'NONE', *, *, #15182, .T. ) ;
#9457=( BOUNDED_CURVE ( )  B_SPLINE_CURVE ( 2, ( #11759, #25380, #27432, #2051, #33221, #20269, #1538, #33043, #9713, #30675, #1370 ),
 .UNSPECIFIED., .F., .F. ) 
 B_SPLINE_CURVE_WITH_KNOTS ( ( 3, 2, 2, 2, 2, 3 ),
 ( 0.3749999999999998890, 0.3785714285714284477, 0.3821428571428570620, 0.3857142857142856762, 0.3892857142857142905, 0.3928571428571428492 ),
 .UNSPECIFIED. ) 
 CURVE ( )  GEOMETRIC_REPRESENTATION_ITEM ( )  RATIONAL_B_SPLINE_CURVE ( ( 1.000000000000001554, 0.9510565162951518658, 1.000000000000000000, 0.9510565162951534202, 1.000000000000000000, 0.9510565162951534202, 1.000000000000000000, 0.9510565162951534202, 1.000000000000000000, 0.9510565162951534202, 1.000000000000000000 ) ) 
 REPRESENTATION_ITEM ( '' )  );
#9461=CARTESIAN_POINT ( 'NONE',  ( 83.02499999726879309, 149.9369285172503510, -15.58253175000000823 ) ) ;
#9464=CARTESIAN_POINT ( 'NONE',  ( 75.32499999726881867, 164.1591823560292198, -12.60653300113719766 ) ) ;
#9467=CARTESIAN_POINT ( 'NONE',  ( 38.79999999999999716, 167.3344367211045096, -8.961492836873482304 ) ) ;
#9469=DIRECTION ( 'NONE',  ( 0.000000000000000000, 0.000000000000000000, -1.000000000000000000 ) ) ;
#9470=CARTESIAN_POINT ( 'NONE',  ( 78.28867513459482552, 139.2280666364260071, -4.041636747397287284E-15 ) ) ;
#9472=CARTESIAN_POINT ( 'NONE',  ( 50.52499999726880731, 140.1801316387863778, 4.815267126137185549 ) ) ;
#9473=CARTESIAN_POINT ( 'NONE',  ( 65.17499999726881299, 145.8408176439707802, -12.60653300113719588 ) ) ;
#9489=MECHANICAL_DESIGN_GEOMETRIC_PRESENTATION_REPRESENTATION('',(#26347),#21455);
#9490=EDGE_LOOP ( 'NONE', ( #23028, #18342, #11789, #2259 ) ) ;
#9491=CARTESIAN_POINT ( 'NONE',  ( 68.77499999726880731, 140.1801316387863778, 4.815267126137185549 ) ) ;
#9495=CARTESIAN_POINT ( 'NONE',  ( 81.17499999726882720, 145.8408176439707802, -12.60653300113719588 ) ) ;
#9508=CARTESIAN_POINT ( 'NONE',  ( 67.78867513459482552, 155.0000000000000000, 15.00000000000001243 ) ) ;
#9512=CARTESIAN_POINT ( 'NONE',  ( 47.22499999726881015, 160.0630714827496206, -15.58253175000000823 ) ) ;
#9514=CARTESIAN_POINT ( 'NONE',  ( 33.22499999726881725, 160.0630714827496206, -15.58253175000000823 ) ) ;
#9524=CARTESIAN_POINT ( 'NONE',  ( 70.49999999453763166, 170.2462022514548323, -7.872454543227099337E-15 ) ) ;
#9525=ORIENTED_EDGE ( 'NONE', *, *, #10237, .T. ) ;
#9532=ORIENTED_EDGE ( 'NONE', *, *, #19724, .F. ) ;
#9540=CARTESIAN_POINT ( 'NONE',  ( 58.37499999726881583, 155.0000000000000000, 15.58253174999999402 ) ) ;
#9541=VERTEX_POINT ( 'NONE', #24382 ) ;
#9543=DIRECTION ( 'NONE',  ( 1.000000000000000000, 0.000000000000000000, 0.000000000000000000 ) ) ;
#9545=DIRECTION ( 'NONE',  ( 1.000000000000000000, 0.000000000000000000, 0.000000000000000000 ) ) ;
#9547=CARTESIAN_POINT ( 'NONE',  ( 68.27499999726879309, 160.0630714827496206, 15.58253174999999402 ) ) ;
#9553=CARTESIAN_POINT ( 'NONE',  ( 78.30000000000001137, 146.4771138417591203, -11.73074641843674470 ) ) ;
#9557=DIRECTION ( 'NONE',  ( 0.000000000000000000, 0.000000000000000000, -1.000000000000000000 ) ) ;
#9558=CARTESIAN_POINT ( 'NONE',  ( 50.97499999726881725, 140.1801316387863778, -4.815267126137194431 ) ) ;
#9560=CARTESIAN_POINT ( 'NONE',  ( 81.32499999726880446, 164.1591823560292198, -12.60653300113719766 ) ) ;
#9563=CARTESIAN_POINT ( 'NONE',  ( 49.29999999453762172, 142.6655632788954620, 8.961492836873471646 ) ) ;
#9569=ORIENTED_EDGE ( 'NONE', *, *, #12085, .F. ) ;
#9576=EDGE_CURVE ( 'NONE', #19849, #1328, #32730, .T. ) ;
#9581=CARTESIAN_POINT ( 'NONE',  ( 35.37499999726881583, 155.0000000000000000, -15.58253175000000823 ) ) ;
#9583=CARTESIAN_POINT ( 'NONE',  ( 46.42499999726880588, 141.7447067706911810, 9.630534252274376428 ) ) ;
#9585=DIRECTION ( 'NONE',  ( 0.000000000000000000, 0.000000000000000000, -1.000000000000000000 ) ) ;
#9587=CARTESIAN_POINT ( 'NONE',  ( 49.57499999726881157, 164.1591823560292198, -12.60653300113719766 ) ) ;
#9592=CARTESIAN_POINT ( 'NONE',  ( 59.50000000000000000, 155.0000000000000000, 14.49999999999999467 ) ) ;
#9601=CARTESIAN_POINT ( 'NONE',  ( 61.22499999726880304, 160.0630714827496206, -15.58253175000000823 ) ) ;
#9605=CARTESIAN_POINT ( 'NONE',  ( 84.17499999726882720, 164.1591823560292198, 12.60653300113718167 ) ) ;
#9612=CARTESIAN_POINT ( 'NONE',  ( 32.50000000000000000, 155.0000000000000000, -6.938893903907228378E-15 ) ) ;
#9621=ORIENTED_EDGE ( 'NONE', *, *, #3053, .F. ) ;
#9626=CARTESIAN_POINT ( 'NONE',  ( 77.22499999726881015, 160.0630714827496206, -15.58253175000000823 ) ) ;
#9629=CARTESIAN_POINT ( 'NONE',  ( 87.50000000000005684, 169.6253155642411343, -5.351338237494227101 ) ) ;
#9633=CARTESIAN_POINT ( 'NONE',  ( 39.50000000000000000, 155.0000000000000000, 14.49999999999999467 ) ) ;
#9639=CARTESIAN_POINT ( 'NONE',  ( 49.72499999726881725, 169.8198683612136222, 4.815267126137181997 ) ) ;
#9640=CARTESIAN_POINT ( 'NONE',  ( 61.07499999726881867, 141.7447067706911810, -9.630534252274385310 ) ) ;
#9648=( BOUNDED_CURVE ( )  B_SPLINE_CURVE ( 2, ( #29871, #3460, #16910, #6184, #27306, #9250, #16575, #19644, #30033, #14693, #23211, #4472, #33606, #2437, #9932, #20145, #25257, #4812, #25424, #17250, #9581, #12142, #12485, #30719, #30541, #10285, #27638, #27805, #20315, #12818, #1923, #25597, #20664, #25085, #17590, #25766, #22874, #22704, #9762, #23040, #14861, #1743, #10108, #19974, #33436, #20486, #30889, #17420, #2263, #31058, #33265, #33093, #7204, #7554, #12309, #15374, #7379, #4307, #28155, #27981, #17758, #4648, #12645, #15032, #2098, #17941, #22537, #15206, #28329, #4987, #32922, #30376, #7038, #21149, #3254, #13154, #10773, #28498, #18268, #15871, #8053, #13317, #24036, #2775, #12992, #20820, #7887, #23386, #13642, #13480, #5482, #50, #31709, #25931, #5316, #28990, #28657, #10446, #23546, #26589, #15705, #21485, #5151, #5803, #26107, #15539, #215, #31223, #18769, #10612, #5649, #23873, #20987, #704, #31383, #18437, #28826, #545, #26266, #7717, #2605, #370, #11106, #2934, #23709, #31547, #8215, #21313, #8381, #18603, #16037, #26428, #10937, #3091, #29152, #18103, #16199, #13981, #18929, #8706, #32537, #27102, #29325, #8867, #6140, #3419, #22149, #16533, #5973, #4090, #19096, #14480, #17040, #24545, #1043, #26930, #19428, #6307, #31869, #24207, #3764, #14149, #11598, #11435, #24877, #8534, #29484, #1199, #27434, #3588, #6492, #1540, #16361, #32204, #11937, #1373, #24377, #26755, #21812, #9213, #13814, #870, #19265, #29658, #11266, #19603, #16702, #21648, #32043, #21986, #32372, #9036, #29831, #16871, #27264, #3921, #14320, #24717, #11761, #29995, #6652, #2053, #1881, #4942, #22320, #32880, #14993, #17894, #6996, #30678, #25722, #30164, #22658, #30846, #17546, #27766, #14818, #28108, #19931, #20447, #4610, #25051, #4769, #15163, #25556, #22494, #7342, #30329, #12266, #2220, #32706, #30499, #12604, #9888, #25382, #17382, #17721, #12441, #28288, #4430, #22832, #17207, #22999, #2395, #25216, #27940, #15328, #33046, #27594, #1704, #9540, #4261, #9373, #33399, #20106, #14655, #10070, #6822, #9715, #20271, #7162, #33224, #7510, #19769, #12101, #26545, #33563, #10896, #31174, #20620, #5272, #2562, #23831, #25893, #10728, #28947, #9, #5761, #23345, #18058, #18230, #10404, #12781, #31019, #20777, #8010, #26068, #26220, #5604, #15503, #23172, #12950, #16154, #7845, #13112, #18562, #170, #15666, #23667, #502, #28788, #28620, #327, #2738, #28453, #23503, #31669, #10570, #20948, #31342, #5112, #21110, #18395, #5445, #15830, #18728, #31509, #29112, #10242, #2888, #13275, #8177, #15997, #26389, #3048, #13433, #7676, #21273, #8337, #32160, #16489, #16658, #29784, #5931, #3216, #3376, #29953, #31997, #3546, #8997, #24326, #27055, #6609, #6449, #19053, #23998, #13770, #3879, #660, #3718, #26888, #21445, #24167, #14106, #24501, #19222, #8820, #13938, #18885, #29619, #16830, #6091, #11219, #1160, #11394, #13602, #29280, #6267, #16993, #27224, #21601, #16323, #11553, #14272, #997, #21771, #829, #21941, #32331, #1336, #19386, #11723, #24672, #8662, #29443, #22109, #32496, #9168, #19561, #11063, #31827, #8493, #26714, #27847, #20188, #25301, #4520, #14910, #12356, #1965, #22752, #33145, #9808, #30587, #7252, #5923, #21764, #31662, #29272, #12814, #3043, #654, #26539, #26382, #10281, #8814, #8329, #11055, #11387, #16317, #26708, #31988, #23991, #823, #23823, #16148, #8656, #25761, #21436, #19047, #13763, #8487, #21267, #11214, #3370, #32154, #18722, #24158, #23206, #13428, #31821, #494, #18878, #19214, #29107, #31054, #5598, #10891, #8171, #29613, #29436, #21596, #18554, #16482, #20659, #5754, #6085, #3209, #28939, #13597, #6261, #26880, #2433, #33602, #24320, #3538, #15991, #13931, #989, #27725, #29776, #14608, #32829, #3873, #9664, #27218, #21932, #22103, #9495, #14266, #16650, #6945, #9324, #32996, #29947, #27380, #24666, #14437, #30279, #17334, #11717, #1329, #30111, #19882, #32490, #6775, #20056, #4384, #9159, #3711, #19554, #14770, #11888, #14100, #4046, #6603, #32325, #25162, #16986, #24494, #22609, #24830, #30456, #1828, #19716, #1494, #22275, #4210, #32659, #27049, #8991, #11547, #17160, #27546, #25004, #1155, #19379, #1656, #12050, #12221, #22438, #6441, #16823, #15476, #30813, #10205, #18534, #12916, #2708, #28259, #28916, #13086, #26363 ),
 .UNSPECIFIED., .F., .T. ) 
 B_SPLINE_CURVE_WITH_KNOTS ( ( 3, 2, 2, 2, 2, 2, 2, 2, 2, 2, 2, 2, 2, 2, 2, 2, 2, 2, 2, 2, 2, 2, 2, 2, 2, 2, 2, 2, 2, 2, 2, 2, 2, 2, 2, 2, 2, 2, 2, 2, 2, 2, 2, 2, 2, 2, 2, 2, 2, 2, 2, 2, 2, 2, 2, 2, 2, 2, 2, 2, 2, 2, 2, 2, 2, 2, 2, 2, 2, 2, 2, 2, 2, 2, 2, 2, 2, 2, 2, 2, 2, 2, 2, 2, 2, 2, 2, 2, 2, 2, 2, 2, 2, 2, 2, 2, 2, 2, 2, 2, 2, 2, 2, 2, 2, 2, 2, 2, 2, 2, 2, 2, 2, 2, 2, 2, 2, 2, 2, 2, 2, 2, 2, 2, 2, 2, 2, 2, 2, 2, 2, 2, 2, 2, 2, 2, 2, 2, 2, 2, 2, 2, 2, 2, 2, 2, 2, 2, 2, 2, 2, 2, 2, 2, 2, 2, 2, 2, 2, 2, 2, 2, 2, 2, 2, 2, 2, 2, 2, 2, 2, 2, 2, 2, 2, 2, 2, 2, 2, 2, 2, 2, 2, 2, 2, 2, 2, 2, 2, 2, 2, 2, 2, 2, 2, 2, 2, 2, 2, 2, 2, 2, 2, 2, 2, 2, 2, 2, 2, 2, 2, 2, 2, 2, 2, 2, 2, 2, 2, 2, 2, 2, 2, 2, 2, 2, 2, 2, 2, 2, 2, 2, 2, 2, 2, 2, 2, 2, 2, 2, 2, 2, 2, 2, 2, 2, 2, 2, 2, 2, 2, 2, 2, 2, 2, 2, 2, 2, 2, 2, 2, 2, 2, 2, 2, 2, 2, 2, 2, 2, 2, 3 ),
 ( 0.000000000000000000, 0.003571428571428571317, 0.007142857142857142634, 0.01071428571428571438, 0.01428571428571428527, 0.01785714285714285615, 0.02142857142857142877, 0.02500000000000000139, 0.02857142857142857054, 0.03214285714285713969, 0.03571428571428571230, 0.03928571428571428492, 0.04285714285714285754, 0.04642857142857143016, 0.05000000000000000278, 0.05357142857142856845, 0.05714285714285714107, 0.06071428571428571369, 0.06428571428571427937, 0.06785714285714285199, 0.07142857142857142461, 0.07499999999999999722, 0.07857142857142856984, 0.08214285714285714246, 0.08571428571428571508, 0.08928571428571428770, 0.09285714285714286031, 0.09642857142857143293, 0.1000000000000000056, 0.1035714285714285782, 0.1071428571428571369, 0.1107142857142857095, 0.1142857142857142821, 0.1178571428571428548, 0.1214285714285714274, 0.1250000000000000000, 0.1285714285714285587, 0.1321428571428571452, 0.1357142857142857040, 0.1392857142857142905, 0.1428571428571428492, 0.1464285714285714357, 0.1499999999999999944, 0.1535714285714285809, 0.1571428571428571397, 0.1607142857142857262, 0.1642857142857142849, 0.1678571428571428437, 0.1714285714285714302, 0.1749999999999999889, 0.1785714285714285754, 0.1821428571428571341, 0.1857142857142857206, 0.1892857142857142794, 0.1928571428571428659, 0.1964285714285714246, 0.2000000000000000111, 0.2035714285714285698, 0.2071428571428571563, 0.2107142857142857151, 0.2142857142857142738, 0.2178571428571428603, 0.2214285714285714191, 0.2250000000000000056, 0.2285714285714285643, 0.2321428571428571508, 0.2357142857142857095, 0.2392857142857142960, 0.2428571428571428548, 0.2464285714285714413, 0.2500000000000000000, 0.2535714285714285587, 0.2571428571428571175, 0.2607142857142857317, 0.2642857142857142905, 0.2678571428571428492, 0.2714285714285714080, 0.2749999999999999667, 0.2785714285714285809, 0.2821428571428571397, 0.2857142857142856984, 0.2892857142857143127, 0.2928571428571428714, 0.2964285714285714302, 0.2999999999999999889, 0.3035714285714285476, 0.3071428571428571619, 0.3107142857142857206, 0.3142857142857142794, 0.3178571428571428381, 0.3214285714285714524, 0.3249999999999999556, 0.3285714285714285698, 0.3321428571428571286, 0.3357142857142856873, 0.3392857142857143016, 0.3428571428571428603, 0.3464285714285714191, 0.3499999999999999778, 0.3535714285714285920, 0.3571428571428571508, 0.3607142857142857095, 0.3642857142857142683, 0.3678571428571428825, 0.3714285714285714413, 0.3750000000000000555, 0.3785714285714285587, 0.3821428571428571175, 0.3857142857142857317, 0.3892857142857142905, 0.3928571428571428492, 0.3964285714285714080, 0.4000000000000000222, 0.4035714285714285809, 0.4071428571428571397, 0.4107142857142856984, 0.4142857142857143127, 0.4178571428571428714, 0.4214285714285714302, 0.4250000000000000444, 0.4285714285714285476, 0.4321428571428571619, 0.4357142857142857206, 0.4392857142857142794, 0.4428571428571428381, 0.4464285714285714524, 0.4500000000000000111, 0.4535714285714285698, 0.4571428571428571286, 0.4607142857142856873, 0.4642857142857143016, 0.4678571428571428603, 0.4714285714285714191, 0.4750000000000000333, 0.4785714285714285920, 0.4821428571428571508, 0.4857142857142857095, 0.4892857142857142683, 0.4928571428571428825, 0.4964285714285714413, 0.5000000000000000000, 0.5035714285714285587, 0.5071428571428571175, 0.5107142857142856762, 0.5142857142857142350, 0.5178571428571429047, 0.5214285714285714635, 0.5250000000000000222, 0.5285714285714285809, 0.5321428571428571397, 0.5357142857142856984, 0.5392857142857142572, 0.5428571428571428159, 0.5464285714285713746, 0.5499999999999999334, 0.5535714285714286031, 0.5571428571428571619, 0.5607142857142857206, 0.5642857142857142794, 0.5678571428571428381, 0.5714285714285713969, 0.5749999999999999556, 0.5785714285714286254, 0.5821428571428571841, 0.5857142857142857428, 0.5892857142857143016, 0.5928571428571428603, 0.5964285714285714191, 0.5999999999999999778, 0.6035714285714285365, 0.6071428571428570953, 0.6107142857142857650, 0.6142857142857143238, 0.6178571428571428825, 0.6214285714285714413, 0.6250000000000000000, 0.6285714285714285587, 0.6321428571428571175, 0.6357142857142856762, 0.6392857142857142350, 0.6428571428571429047, 0.6464285714285714635, 0.6499999999999999112, 0.6535714285714285809, 0.6571428571428571397, 0.6607142857142856984, 0.6642857142857142572, 0.6678571428571428159, 0.6714285714285713746, 0.6750000000000000444, 0.6785714285714286031, 0.6821428571428571619, 0.6857142857142857206, 0.6892857142857142794, 0.6928571428571428381, 0.6964285714285713969, 0.6999999999999999556, 0.7035714285714286254, 0.7071428571428571841, 0.7107142857142857428, 0.7142857142857143016, 0.7178571428571428603, 0.7214285714285714191, 0.7249999999999999778, 0.7285714285714285365, 0.7321428571428570953, 0.7357142857142857650, 0.7392857142857143238, 0.7428571428571428825, 0.7464285714285714413, 0.7500000000000001110, 0.7535714285714285587, 0.7571428571428571175, 0.7607142857142856762, 0.7642857142857142350, 0.7678571428571429047, 0.7714285714285714635, 0.7750000000000000222, 0.7785714285714285809, 0.7821428571428571397, 0.7857142857142856984, 0.7892857142857142572, 0.7928571428571428159, 0.7964285714285713746, 0.8000000000000000444, 0.8035714285714286031, 0.8071428571428571619, 0.8107142857142857206, 0.8142857142857142794, 0.8178571428571428381, 0.8214285714285713969, 0.8249999999999999556, 0.8285714285714286254, 0.8321428571428571841, 0.8357142857142857428, 0.8392857142857143016, 0.8428571428571428603, 0.8464285714285714191, 0.8500000000000000888, 0.8535714285714285365, 0.8571428571428570953, 0.8607142857142857650, 0.8642857142857143238, 0.8678571428571428825, 0.8714285714285714413, 0.8750000000000000000, 0.8785714285714285587, 0.8821428571428571175, 0.8857142857142856762, 0.8892857142857142350, 0.8928571428571429047, 0.8964285714285714635, 0.9000000000000000222, 0.9035714285714285809, 0.9071428571428571397, 0.9107142857142856984, 0.9142857142857142572, 0.9178571428571428159, 0.9214285714285713746, 0.9250000000000000444, 0.9285714285714286031, 0.9321428571428571619, 0.9357142857142857206, 0.9392857142857142794, 0.9428571428571428381, 0.9464285714285713969, 0.9500000000000000666, 0.9535714285714286254, 0.9571428571428571841, 0.9607142857142857428, 0.9642857142857143016, 0.9665075840475536584 ),
 .UNSPECIFIED. ) 
 CURVE ( )  GEOMETRIC_REPRESENTATION_ITEM ( )  RATIONAL_B_SPLINE_CURVE ( ( 1.000000000000000000, 0.9510565162951535312, 1.000000000000000000, 0.9510565162951535312, 1.000000000000000000, 0.9510565162951535312, 1.000000000000000000, 0.9510565162951535312, 1.000000000000000000, 0.9510565162951535312, 1.000000000000000000, 0.9510565162951535312, 1.000000000000000000, 0.9510565162951535312, 1.000000000000000000, 0.9510565162951535312, 1.000000000000000000, 0.9510565162951535312, 1.000000000000000000, 0.9510565162951535312, 1.000000000000000000, 0.9510565162951535312, 1.000000000000000000, 0.9510565162951535312, 1.000000000000000000, 0.9510565162951535312, 1.000000000000000000, 0.9510565162951535312, 1.000000000000000000, 0.9510565162951535312, 1.000000000000000000, 0.9510565162951535312, 1.000000000000000000, 0.9510565162951535312, 1.000000000000000000, 0.9510565162951535312, 1.000000000000000000, 0.9510565162951535312, 1.000000000000000000, 0.9510565162951535312, 1.000000000000000000, 0.9510565162951535312, 1.000000000000000000, 0.9510565162951535312, 1.000000000000000000, 0.9510565162951535312, 1.000000000000000000, 0.9510565162951535312, 1.000000000000000000, 0.9510565162951535312, 1.000000000000000000, 0.9510565162951535312, 1.000000000000000000, 0.9510565162951535312, 1.000000000000000000, 0.9510565162951535312, 1.000000000000000000, 0.9510565162951535312, 1.000000000000000000, 0.9510565162951535312, 1.000000000000000000, 0.9510565162951535312, 1.000000000000000000, 0.9510565162951535312, 1.000000000000000000, 0.9510565162951535312, 1.000000000000000000, 0.9510565162951535312, 1.000000000000000000, 0.9510565162951535312, 1.000000000000000000, 0.9510565162951535312, 1.000000000000000000, 0.9510565162951535312, 1.000000000000000000, 0.9510565162951535312, 1.000000000000000000, 0.9510565162951535312, 1.000000000000000000, 0.9510565162951535312, 1.000000000000000000, 0.9510565162951535312, 1.000000000000000000, 0.9510565162951535312, 1.000000000000000000, 0.9510565162951535312, 1.000000000000000000, 0.9510565162951535312, 1.000000000000000000, 0.9510565162951535312, 1.000000000000000000, 0.9510565162951535312, 1.000000000000000000, 0.9510565162951535312, 1.000000000000000000, 0.9510565162951535312, 1.000000000000000000, 0.9510565162951535312, 1.000000000000000000, 0.9510565162951535312, 1.000000000000000000, 0.9510565162951535312, 1.000000000000000000, 0.9510565162951535312, 1.000000000000000000, 0.9510565162951535312, 1.000000000000000000, 0.9510565162951535312, 1.000000000000000000, 0.9510565162951535312, 1.000000000000000000, 0.9510565162951535312, 1.000000000000000000, 0.9510565162951535312, 1.000000000000000000, 0.9510565162951535312, 1.000000000000000000, 0.9510565162951535312, 1.000000000000000000, 0.9510565162951535312, 1.000000000000000000, 0.9510565162951535312, 1.000000000000000000, 0.9510565162951535312, 1.000000000000000000, 0.9510565162951535312, 1.000000000000000000, 0.9510565162951535312, 1.000000000000000000, 0.9510565162951535312, 1.000000000000000000, 0.9510565162951535312, 1.000000000000000000, 0.9510565162951535312, 1.000000000000000000, 0.9510565162951535312, 1.000000000000000000, 0.9510565162951535312, 1.000000000000000000, 0.9510565162951535312, 1.000000000000000000, 0.9510565162951535312, 1.000000000000000000, 0.9510565162951535312, 1.000000000000000000, 0.9510565162951535312, 1.000000000000000000, 0.9510565162951535312, 1.000000000000000000, 0.9510565162951535312, 1.000000000000000000, 0.9510565162951535312, 1.000000000000000000, 0.9510565162951535312, 1.000000000000000000, 0.9510565162951535312, 1.000000000000000000, 0.9510565162951535312, 1.000000000000000000, 0.9510565162951535312, 1.000000000000000000, 0.9510565162951535312, 1.000000000000000000, 0.9510565162951535312, 1.000000000000000000, 0.9510565162951535312, 1.000000000000000000, 0.9510565162951535312, 1.000000000000000000, 0.9510565162951535312, 1.000000000000000000, 0.9510565162951535312, 1.000000000000000000, 0.9510565162951535312, 1.000000000000000000, 0.9510565162951535312, 1.000000000000000000, 0.9510565162951535312, 1.000000000000000000, 0.9510565162951535312, 1.000000000000000000, 0.9510565162951535312, 1.000000000000000000, 0.9510565162951535312, 1.000000000000000000, 0.9510565162951535312, 1.000000000000000000, 0.9510565162951535312, 1.000000000000000000, 0.9510565162951535312, 1.000000000000000000, 0.9510565162951535312, 1.000000000000000000, 0.9510565162951535312, 1.000000000000000000, 0.9510565162951535312, 1.000000000000000000, 0.9510565162951535312, 1.000000000000000000, 0.9510565162951535312, 1.000000000000000000, 0.9510565162951535312, 1.000000000000000000, 0.9510565162951535312, 1.000000000000000000, 0.9510565162951535312, 1.000000000000000000, 0.9510565162951535312, 1.000000000000000000, 0.9510565162951535312, 1.000000000000000000, 0.9510565162951535312, 1.000000000000000000, 0.9510565162951535312, 1.000000000000000000, 0.9510565162951535312, 1.000000000000000000, 0.9510565162951535312, 1.000000000000000000, 0.9510565162951535312, 1.000000000000000000, 0.9510565162951535312, 1.000000000000000000, 0.9510565162951535312, 1.000000000000000000, 0.9510565162951535312, 1.000000000000000000, 0.9510565162951535312, 1.000000000000000000, 0.9510565162951535312, 1.000000000000000000, 0.9510565162951535312, 1.000000000000000000, 0.9510565162951535312, 1.000000000000000000, 0.9510565162951535312, 1.000000000000000000, 0.9510565162951535312, 1.000000000000000000, 0.9510565162951535312, 1.000000000000000000, 0.9510565162951535312, 1.000000000000000000, 0.9510565162951535312, 1.000000000000000000, 0.9510565162951535312, 1.000000000000000000, 0.9510565162951535312, 1.000000000000000000, 0.9510565162951535312, 1.000000000000000000, 0.9510565162951535312, 1.000000000000000000, 0.9510565162951535312, 1.000000000000000000, 0.9510565162951535312, 1.000000000000000000, 0.9510565162951535312, 1.000000000000000000, 0.9510565162951535312, 1.000000000000000000, 0.9510565162951535312, 1.000000000000000000, 0.9510565162951535312, 1.000000000000000000, 0.9510565162951535312, 1.000000000000000000, 0.9510565162951535312, 1.000000000000000000, 0.9510565162951535312, 1.000000000000000000, 0.9510565162951535312, 1.000000000000000000, 0.9510565162951535312, 1.000000000000000000, 0.9510565162951535312, 1.000000000000000000, 0.9510565162951535312, 1.000000000000000000, 0.9510565162951535312, 1.000000000000000000, 0.9510565162951535312, 1.000000000000000000, 0.9510565162951535312, 1.000000000000000000, 0.9510565162951535312, 1.000000000000000000, 0.9510565162951535312, 1.000000000000000000, 0.9510565162951535312, 1.000000000000000000, 0.9510565162951535312, 1.000000000000000000, 0.9510565162951535312, 1.000000000000000000, 0.9510565162951535312, 1.000000000000000000, 0.9510565162951535312, 1.000000000000000000, 0.9510565162951535312, 1.000000000000000000, 0.9510565162951535312, 1.000000000000000000, 0.9510565162951535312, 1.000000000000000000, 0.9510565162951535312, 1.000000000000000000, 0.9510565162951535312, 1.000000000000000000, 0.9510565162951535312, 1.000000000000000000, 0.9510565162951535312, 1.000000000000000000, 0.9510565162951535312, 1.000000000000000000, 0.9510565162951535312, 1.000000000000000000, 0.9510565162951535312, 1.000000000000000000, 0.9510565162951535312, 1.000000000000000000, 0.9510565162951535312, 1.000000000000000000, 0.9510565162951535312, 1.000000000000000000, 0.9510565162951535312, 1.000000000000000000, 0.9510565162951535312, 1.000000000000000000, 0.9510565162951535312, 1.000000000000000000, 0.9510565162951535312, 1.000000000000000000, 0.9510565162951535312, 1.000000000000000000, 0.9510565162951535312, 1.000000000000000000, 0.9510565162951535312, 1.000000000000000000, 0.9510565162951535312, 1.000000000000000000, 0.9510565162951535312, 1.000000000000000000, 0.9510565162951535312, 1.000000000000000000, 0.9510565162951535312, 1.000000000000000000, 0.9510565162951535312, 1.000000000000000000, 0.9510565162951535312, 1.000000000000000000, 0.9510565162951535312, 1.000000000000000000, 0.9510565162951535312, 1.000000000000000000, 0.9510565162951535312, 1.000000000000000000, 0.9510565162951535312, 1.000000000000000000, 0.9510565162951535312, 1.000000000000000000, 0.9510565162951535312, 1.000000000000000000, 0.9510565162951535312, 1.000000000000000000, 0.9510565162951535312, 1.000000000000000000, 0.9510565162951535312, 1.000000000000000000, 0.9510565162951535312, 1.000000000000000000, 0.9510565162951535312, 1.000000000000000000, 0.9510565162951535312, 1.000000000000000000, 0.9510565162951535312, 1.000000000000000000, 0.9510565162951535312, 1.000000000000000000, 0.9510565162951535312, 1.000000000000000000, 0.9510565162951535312, 1.000000000000000000, 0.9510565162951535312, 1.000000000000000000, 0.9510565162951535312, 1.000000000000000000, 0.9510565162951535312, 1.000000000000000000, 0.9510565162951535312, 1.000000000000000000, 0.9510565162951535312, 1.000000000000000000, 0.9510565162951535312, 1.000000000000000000, 0.9510565162951535312, 1.000000000000000000, 0.9510565162951535312, 1.000000000000000000, 0.9510565162951535312, 1.000000000000000000, 0.9510565162951535312, 1.000000000000000000, 0.9510565162951535312, 1.000000000000000000, 0.9510565162951535312, 1.000000000000000000, 0.9510565162951535312, 1.000000000000000000, 0.9510565162951535312, 1.000000000000000000, 0.9510565162951535312, 1.000000000000000000, 0.9510565162951535312, 1.000000000000000000, 0.9510565162951535312, 1.000000000000000000, 0.9510565162951535312, 1.000000000000000000, 0.9510565162951535312, 1.000000000000000000, 0.9510565162951535312, 1.000000000000000000, 0.9510565162951535312, 1.000000000000000000, 0.9510565162951535312, 1.000000000000000000, 0.9510565162951535312, 1.000000000000000000, 0.9510565162951535312, 1.000000000000000000, 0.9510565162951535312, 1.000000000000000000, 0.9510565162951535312, 1.000000000000000000, 0.9510565162951535312, 1.000000000000000000, 0.9510565162951535312, 1.000000000000000000, 0.9510565162951535312, 1.000000000000000000, 0.9510565162951535312, 1.000000000000000000, 0.9510565162951535312, 1.000000000000000000, 0.9510565162951535312, 1.000000000000000000, 0.9510565162951535312, 1.000000000000000000, 0.9510565162951535312, 1.000000000000000000, 0.9510565162951535312, 1.000000000000000000, 0.9510565162951535312, 1.000000000000000000, 0.9510565162951535312, 1.000000000000000000, 0.9510565162951535312, 1.000000000000000000, 0.9510565162951535312, 1.000000000000000000, 0.9510565162951535312, 1.000000000000000000, 0.9510565162951535312, 1.000000000000000000, 0.9510565162951535312, 1.000000000000000000, 0.9510565162951535312, 1.000000000000000000, 0.9510565162951535312, 1.000000000000000000, 0.9510565162951535312, 1.000000000000000000, 0.9510565162951535312, 1.000000000000000000, 0.9510565162951535312, 1.000000000000000000, 0.9510565162951535312, 1.000000000000000000, 0.9510565162951535312, 1.000000000000000000, 0.9510565162951535312, 1.000000000000000000, 0.9510565162951535312, 1.000000000000000000, 0.9510565162951535312, 1.000000000000000000, 0.9510565162951535312, 1.000000000000000000, 0.9510565162951535312, 1.000000000000000000, 0.9510565162951535312, 1.000000000000000000, 0.9510565162951535312, 1.000000000000000000, 0.9510565162951535312, 1.000000000000000000, 0.9510565162951535312, 1.000000000000000000, 0.9510565162951535312, 1.000000000000000000, 0.9510565162951535312, 1.000000000000000000, 0.9510565162951535312, 1.000000000000000000, 0.9510565162951535312, 1.000000000000000000, 0.9510565162951535312, 1.000000000000000000, 0.9510565162951535312, 1.000000000000000000, 0.9510565162951535312, 1.000000000000000000, 0.9510565162951535312, 1.000000000000000000, 0.9510565162951535312, 1.000000000000000000, 0.9510565162951535312, 1.000000000000000000, 0.9510565162951535312, 1.000000000000000000, 0.9510565162951535312, 1.000000000000000000, 0.9510565162951535312, 1.000000000000000000, 0.9510565162951535312, 1.000000000000000000, 0.9510565162951535312, 1.000000000000000000, 0.9510565162951535312, 1.000000000000000000, 0.9510565162951535312, 1.000000000000000000, 0.9510565162951535312, 1.000000000000000000, 0.9510565162951535312, 1.000000000000000000, 0.9510565162951535312, 1.000000000000000000, 0.9510565162951535312, 1.000000000000000000, 0.9695511069847947416, 0.9769881597858905975 ) ) 
 REPRESENTATION_ITEM ( '' )  );
#9650=CARTESIAN_POINT ( 'NONE',  ( 82.71132485994282035, 155.0000000000000000, 15.00000000000001243 ) ) ;
#9656=FACE_BOUND ( 'NONE', #8736, .T. ) ;
#9659=ORIENTED_EDGE ( 'NONE', *, *, #13733, .F. ) ;
#9660=CARTESIAN_POINT ( 'NONE',  ( 77.17499999726881299, 145.8408176439707802, -12.60653300113719588 ) ) ;
#9663=VECTOR ( 'NONE', #30220, 1000.000000000000000 ) ;
#9664=CARTESIAN_POINT ( 'NONE',  ( 80.77499999726880731, 140.1801316387863778, 4.815267126137185549 ) ) ;
#9667=CARTESIAN_POINT ( 'NONE',  ( 56.02499999726880731, 160.0630714827496206, 15.58253174999999402 ) ) ;
#9683=CARTESIAN_POINT ( 'NONE',  ( 51.02499999726880731, 149.9369285172503510, -15.58253175000000823 ) ) ;
#9685=CARTESIAN_POINT ( 'NONE',  ( 87.50000000000000000, 160.9457742543943652, -14.40357817542362540 ) ) ;
#9692=CYLINDRICAL_SURFACE ( 'NONE', #25171, 15.00000000000001776 ) ;
#9693=CARTESIAN_POINT ( 'NONE',  ( 41.71132485994280614, 155.0000000000000000, -15.00000000000002487 ) ) ;
#9696=CARTESIAN_POINT ( 'NONE',  ( 71.59999999453762598, 141.2096805137202580, -4.480746418436742040 ) ) ;
#9703=ORIENTED_EDGE ( 'NONE', *, *, #22723, .F. ) ;
#9708=AXIS2_PLACEMENT_3D ( 'NONE', #1657, #27050, #22104 ) ;
#9709=CARTESIAN_POINT ( 'NONE',  ( 58.38867513459481984, 140.7341522555726669, -4.635254915624220651 ) ) ;
#9711=ORIENTED_EDGE ( 'NONE', *, *, #33130, .T. ) ;
#9713=CARTESIAN_POINT ( 'NONE',  ( 55.51132485994280330, 146.1832212156128890, -12.13525491562423042 ) ) ;
#9715=CARTESIAN_POINT ( 'NONE',  ( 59.17499999726881299, 145.8408176439707802, -12.60653300113719588 ) ) ;
#9716=AXIS2_PLACEMENT_3D ( 'NONE', #30775, #2158, #28216 ) ;
#9719=CARTESIAN_POINT ( 'NONE',  ( 66.81132485994281467, 150.1262045565066785, 15.00000000000020250 ) ) ;
#9720=CARTESIAN_POINT ( 'NONE',  ( 56.91132485994280898, 146.1832212156128890, 12.13525491562421976 ) ) ;
#9722=CARTESIAN_POINT ( 'NONE',  ( 67.07499999726880446, 141.7447067706911810, -9.630534252274385310 ) ) ;
#9724=CARTESIAN_POINT ( 'NONE',  ( 70.28867513459482552, 139.2280666364260071, -4.041636747397287284E-15 ) ) ;
#9725=EDGE_CURVE ( 'NONE', #534, #14229, #20109, .T. ) ;
#9728=CARTESIAN_POINT ( 'NONE',  ( 77.50000000000001421, 155.0000000000000000, 14.49999999999999467 ) ) ;
#9733=CARTESIAN_POINT ( 'NONE',  ( 48.48867513459482836, 142.2402378747194405, -9.270509831248439525 ) ) ;
#9734=CARTESIAN_POINT ( 'NONE',  ( 51.57499999726881157, 164.1591823560292198, -12.60653300113719766 ) ) ;
#9736=CARTESIAN_POINT ( 'NONE',  ( 81.72499999726881015, 169.8198683612136222, 4.815267126137181997 ) ) ;
#9738=TOROIDAL_SURFACE ( 'NONE', #23338, 70.00000000000001421, 30.00000000000000000 ) ;
#9739=CARTESIAN_POINT ( 'NONE',  ( 42.21132485994281325, 170.7719333635740497, -7.904646289410545231E-15 ) ) ;
#9742=CARTESIAN_POINT ( 'NONE',  ( 53.69999999453762030, 142.6655632788954620, -8.961492836873480528 ) ) ;
#9762=CARTESIAN_POINT ( 'NONE',  ( 37.17499999726881299, 145.8408176439707802, -12.60653300113719588 ) ) ;
#9763=ORIENTED_EDGE ( 'NONE', *, *, #4596, .T. ) ;
#9764=CARTESIAN_POINT ( 'NONE',  ( 45.22499999726881015, 160.0630714827496206, -15.58253175000000823 ) ) ;
#9766=CARTESIAN_POINT ( 'NONE',  ( 54.41132485994280188, 167.7597621252805880, 9.270509831248428867 ) ) ;
#9768=CARTESIAN_POINT ( 'NONE',  ( 49.67499999726879878, 168.2552932293087906, -9.630534252274385310 ) ) ;
#9772=CARTESIAN_POINT ( 'NONE',  ( 60.70000000000000284, 163.5228861582408797, -11.73074641843674470 ) ) ;
#9774=CARTESIAN_POINT ( 'NONE',  ( 64.61132485994281183, 159.8737954434938615, 14.99999999999982592 ) ) ;
#9779=CARTESIAN_POINT ( 'NONE',  ( 66.62499999726881583, 138.6155565068815463, -3.929120461958505118E-15 ) ) ;
#9783=CARTESIAN_POINT ( 'NONE',  ( 87.17499999726881299, 145.8408176439707802, -12.60653300113719588 ) ) ;
#9787=DIRECTION ( 'NONE',  ( -1.000000000000000000, -0.000000000000000000, -0.000000000000000000 ) ) ;
#9795=ADVANCED_FACE ( 'NONE', ( #14658 ), #7482, .T. ) ;
#9801=EDGE_CURVE ( 'NONE', #3092, #26053, #14821, .T. ) ;
#9808=CARTESIAN_POINT ( 'NONE',  ( 73.57499999726880446, 164.1591823560292198, -12.60653300113719766 ) ) ;
#9809=CARTESIAN_POINT ( 'NONE',  ( 82.52499999726880731, 140.1801316387863778, 4.815267126137185549 ) ) ;
#9810=DIRECTION ( 'NONE',  ( 1.000000000000000000, 0.000000000000000000, 0.000000000000000000 ) ) ;
#9811=( BOUNDED_CURVE ( )  B_SPLINE_CURVE ( 2, ( #9650, #25149, #1989, #25323, #17485, #21799, #14137, #30445, #1815, #17824, #7105 ),
 .UNSPECIFIED., .F., .T. ) 
 B_SPLINE_CURVE_WITH_KNOTS ( ( 3, 2, 2, 2, 2, 3 ),
 ( 0.8750000000000001110, 0.8785714285714286698, 0.8821428571428572285, 0.8857142857142856762, 0.8892857142857142350, 0.8928571428571429047 ),
 .UNSPECIFIED. ) 
 CURVE ( )  GEOMETRIC_REPRESENTATION_ITEM ( )  RATIONAL_B_SPLINE_CURVE ( ( 0.9999999999999984457, 0.9510565162951549745, 1.000000000000000000, 0.9510565162951534202, 1.000000000000000000, 0.9510565162951534202, 1.000000000000000000, 0.9510565162951534202, 1.000000000000000000, 0.9510565162951534202, 1.000000000000000000 ) ) 
 REPRESENTATION_ITEM ( '' )  );
#9813=CARTESIAN_POINT ( 'NONE',  ( 117.5000000000000142, 155.0000000000000000, 70.00000000000000000 ) ) ;
#9815=CARTESIAN_POINT ( 'NONE',  ( 44.50000000000000000, 155.0000000000000000, -14.50000000000000711 ) ) ;
#9818=CARTESIAN_POINT ( 'NONE',  ( 127.5000000000000000, 80.04668119422552763, -74.95331880577366235 ) ) ;
#9820=CARTESIAN_POINT ( 'NONE',  ( 58.52499999726881441, 140.1801316387863778, 4.815267126137185549 ) ) ;
#9821=CARTESIAN_POINT ( 'NONE',  ( 63.77499999726880731, 169.8198683612136222, -4.815267126137197984 ) ) ;
#9825=EDGE_CURVE ( 'NONE', #10137, #18787, #1884, .T. ) ;
#9837=EDGE_LOOP ( 'NONE', ( #13347, #23624, #16572, #4687 ) ) ;
#9840=CARTESIAN_POINT ( 'NONE',  ( 79.47499999726881015, 160.0630714827496206, -15.58253175000000823 ) ) ;
#9843=CARTESIAN_POINT ( 'NONE',  ( 72.22499999726881015, 149.9369285172503510, 15.58253174999999580 ) ) ;
#9846=CARTESIAN_POINT ( 'NONE',  ( 64.62499999726881583, 138.6155565068815463, -3.929120461958505118E-15 ) ) ;
#9849=ORIENTED_EDGE ( 'NONE', *, *, #32645, .F. ) ;
#9856=CARTESIAN_POINT ( 'NONE',  ( 45.08867513459482268, 167.7597621252805880, -9.270509831248443078 ) ) ;
#9860=LINE ( 'NONE', #33533, #12772 ) ;
#9861=CARTESIAN_POINT ( 'NONE',  ( 39.92499999726881299, 164.1591823560292198, 12.60653300113718167 ) ) ;
#9863=CARTESIAN_POINT ( 'NONE',  ( 81.98867513459481415, 146.1832212156128890, 12.13525491562421976 ) ) ;
#9866=LINE ( 'NONE', #30999, #7262 ) ;
#9867=CARTESIAN_POINT ( 'NONE',  ( 54.18867513459482410, 140.7341522555726669, 4.635254915624211769 ) ) ;
#9871=CARTESIAN_POINT ( 'NONE',  ( 73.69999999453762030, 142.6655632788954620, -8.961492836873480528 ) ) ;
#9877=ORIENTED_EDGE ( 'NONE', *, *, #16132, .T. ) ;
#9884=ORIENTED_EDGE ( 'NONE', *, *, #31661, .T. ) ;
#9888=CARTESIAN_POINT ( 'NONE',  ( 56.67499999726881299, 141.7447067706911810, 9.630534252274376428 ) ) ;
#9891=CARTESIAN_POINT ( 'NONE',  ( 66.71132485994280614, 155.0000000000000000, 15.00000000000001243 ) ) ;
#9896=CARTESIAN_POINT ( 'NONE',  ( 68.07499999726881867, 168.2552932293087906, 9.630534252274372875 ) ) ;
#9900=FACE_OUTER_BOUND ( 'NONE', #8178, .T. ) ;
#9903=CARTESIAN_POINT ( 'NONE',  ( 87.20000000000000284, 167.3344367211045096, 8.961492836873468093 ) ) ;
#9907=CARTESIAN_POINT ( 'NONE',  ( 125.5000000000000000, 261.0000000000000000, 0.000000000000000000 ) ) ;
#9908=CARTESIAN_POINT ( 'NONE',  ( 48.77499999726880731, 140.1801316387863778, 4.815267126137185549 ) ) ;
#9913=CARTESIAN_POINT ( 'NONE',  ( 55.89999999453761603, 150.2886644046228639, -14.50000000000000888 ) ) ;
#9918=LINE ( 'NONE', #4801, #23209 ) ;
#9932=CARTESIAN_POINT ( 'NONE',  ( 34.77499999726880731, 140.1801316387863778, 4.815267126137185549 ) ) ;
#9934=CARTESIAN_POINT ( 'NONE',  ( 43.32499999726881157, 164.1591823560292198, -12.60653300113719766 ) ) ;
#9939=CARTESIAN_POINT ( 'NONE',  ( 48.17499999726881299, 164.1591823560292198, 12.60653300113718167 ) ) ;
#9940=DIRECTION ( 'NONE',  ( 0.000000000000000000, 0.000000000000000000, -1.000000000000000000 ) ) ;
#9942=CARTESIAN_POINT ( 'NONE',  ( 58.21132485994281325, 170.7719333635740497, -7.904646289410545231E-15 ) ) ;
#9943=CARTESIAN_POINT ( 'NONE',  ( 68.59999999999996589, 159.7113355953771077, -14.50000000000000888 ) ) ;
#9948=CARTESIAN_POINT ( 'NONE',  ( 34.67499999726880588, 141.7447067706911810, 9.630534252274376428 ) ) ;
#9950=CARTESIAN_POINT ( 'NONE',  ( 62.72499999726881015, 140.1801316387863778, -4.815267126137194431 ) ) ;
#9955=CARTESIAN_POINT ( 'NONE',  ( 87.47499999726883857, 160.0630714827496206, -15.58253175000000823 ) ) ;
#9959=DIRECTION ( 'NONE',  ( 0.000000000000000000, 0.000000000000000000, -1.000000000000000000 ) ) ;
#9968=AXIS2_PLACEMENT_3D ( 'NONE', #24694, #17361, #27914 ) ;
#9970=VERTEX_POINT ( 'NONE', #5447 ) ;
#9971=CARTESIAN_POINT ( 'NONE',  ( 70.01132485994281751, 167.7597621252805880, -9.270509831248443078 ) ) ;
#9980=CARTESIAN_POINT ( 'NONE',  ( 82.22499999726882436, 149.9369285172503510, 15.58253174999999580 ) ) ;
#9981=DIRECTION ( 'NONE',  ( -1.000000000000000000, 0.000000000000000000, 0.000000000000000000 ) ) ;
#9986=CARTESIAN_POINT ( 'NONE',  ( 43.70000000000000284, 146.4771138417591203, 11.73074641843673227 ) ) ;
#9989=VECTOR ( 'NONE', #22301, 1000.000000000000000 ) ;
#9993=CARTESIAN_POINT ( 'NONE',  ( 54.72499999726881015, 140.1801316387863778, -4.815267126137194431 ) ) ;
#9994=CARTESIAN_POINT ( 'NONE',  ( 72.07499999726880446, 168.2552932293087906, 9.630534252274372875 ) ) ;
#10011=CIRCLE ( 'NONE', #8374, 2.149999999999974598 ) ;
#10012=FACE_OUTER_BOUND ( 'NONE', #7039, .T. ) ;
#10017=CARTESIAN_POINT ( 'NONE',  ( 76.87499999726881583, 138.6155565068815463, -3.929120461958505118E-15 ) ) ;
#10020=( BOUNDED_CURVE ( )  B_SPLINE_CURVE ( 2, ( #8038, #5471, #3404, #856, #15857, #18913, #357, #18589, #16183, #26250, #8520 ),
 .UNSPECIFIED., .F., .T. ) 
 B_SPLINE_CURVE_WITH_KNOTS ( ( 3, 2, 2, 2, 2, 3 ),
 ( 0.7678571428571427937, 0.7714285714285713524, 0.7749999999999999112, 0.7785714285714285809, 0.7821428571428571397, 0.7857142857142856984 ),
 .UNSPECIFIED. ) 
 CURVE ( )  GEOMETRIC_REPRESENTATION_ITEM ( )  RATIONAL_B_SPLINE_CURVE ( ( 1.000000000000001554, 0.9510565162951518658, 1.000000000000000000, 0.9510565162951534202, 1.000000000000000000, 0.9510565162951534202, 1.000000000000000000, 0.9510565162951534202, 1.000000000000000000, 0.9510565162951534202, 1.000000000000000000 ) ) 
 REPRESENTATION_ITEM ( '' )  );
#10021=CARTESIAN_POINT ( 'NONE',  ( 70.52499999726880731, 140.1801316387863778, 4.815267126137185549 ) ) ;
#10025=CARTESIAN_POINT ( 'NONE',  ( 65.92499999726881299, 164.1591823560292198, 12.60653300113718167 ) ) ;
#10033=CARTESIAN_POINT ( 'NONE',  ( 127.5000000000000000, 261.0000000000000000, -2.149999999999985256 ) ) ;
#10044=CARTESIAN_POINT ( 'NONE',  ( 40.82499999726880446, 141.7447067706911810, -9.630534252274387086 ) ) ;
#10053=CARTESIAN_POINT ( 'NONE',  ( 75.39999999453762314, 141.2096805137202580, 4.480746418436733158 ) ) ;
#10054=ORIENTED_EDGE ( 'NONE', *, *, #29938, .T. ) ;
#10058=CARTESIAN_POINT ( 'NONE',  ( 75.01132485994280330, 142.2402378747194405, 9.270509831248432420 ) ) ;
#10064=CARTESIAN_POINT ( 'NONE',  ( 32.50000000000000000, 155.0000000000000000, 15.00000000000001243 ) ) ;
#10065=CARTESIAN_POINT ( 'NONE',  ( 56.78867513459481842, 155.0000000000000000, -15.00000000000002487 ) ) ;
#10070=CARTESIAN_POINT ( 'NONE',  ( 58.97499999726881015, 140.1801316387863778, -4.815267126137194431 ) ) ;
#10076=CARTESIAN_POINT ( 'NONE',  ( 64.97499999726881015, 140.1801316387863778, -4.815267126137194431 ) ) ;
#10083=CARTESIAN_POINT ( 'NONE',  ( 86.40000000000001990, 150.2886644046228639, -14.50000000000000888 ) ) ;
#10087=CARTESIAN_POINT ( 'NONE',  ( 64.48867513459482836, 142.2402378747194405, -9.270509831248439525 ) ) ;
#10088=CARTESIAN_POINT ( 'NONE',  ( 48.67499999726881299, 141.7447067706911810, 9.630534252274376428 ) ) ;
#10093=CARTESIAN_POINT ( 'NONE',  ( 57.09999999453762598, 150.2886644046228639, 14.49999999999999645 ) ) ;
#10096=DIRECTION ( 'NONE',  ( 1.000000000000000000, 0.000000000000000000, 0.000000000000000000 ) ) ;
#10098=CYLINDRICAL_SURFACE ( 'NONE', #7996, 2.149999999999985256 ) ;
#10099=ORIENTED_EDGE ( 'NONE', *, *, #351, .T. ) ;
#10102=VERTEX_POINT ( 'NONE', #17724 ) ;
#10104=CYLINDRICAL_SURFACE ( 'NONE', #25211, 2.149999999999985256 ) ;
#10108=CARTESIAN_POINT ( 'NONE',  ( 37.57499999726881157, 164.1591823560292198, -12.60653300113719766 ) ) ;
#10110=CARTESIAN_POINT ( 'NONE',  ( 41.82499999726881157, 168.2552932293087906, 9.630534252274372875 ) ) ;
#10111=CARTESIAN_POINT ( 'NONE',  ( 39.71132485994280614, 155.0000000000000000, -15.00000000000002487 ) ) ;
#10114=CARTESIAN_POINT ( 'NONE',  ( 46.57499999726881157, 145.8408176439707802, 12.60653300113718345 ) ) ;
#10118=CARTESIAN_POINT ( 'NONE',  ( 67.39999999999997726, 159.7113355953771077, 14.49999999999999289 ) ) ;
#10125=EDGE_CURVE ( 'NONE', #29866, #12770, #25976, .T. ) ;
#10126=CARTESIAN_POINT ( 'NONE',  ( 72.92499999726881299, 145.8408176439707802, -12.60653300113719588 ) ) ;
#10129=CARTESIAN_POINT ( 'NONE',  ( 34.19999999453762740, 163.5228861582408797, -11.73074641843674470 ) ) ;
#10137=VERTEX_POINT ( 'NONE', #29445 ) ;
#10144=DIRECTION ( 'NONE',  ( 1.000000000000000000, 0.000000000000000000, 0.000000000000000000 ) ) ;
#10148=CARTESIAN_POINT ( 'NONE',  ( 80.82499999726880446, 141.7447067706911810, -9.630534252274385310 ) ) ;
#10152=CARTESIAN_POINT ( 'NONE',  ( 47.00000000000000000, 170.2462022514548323, -7.872454543227099337E-15 ) ) ;
#10156=AXIS2_PLACEMENT_3D ( 'NONE', #11584, #6642, #29648 ) ;
#10160=CARTESIAN_POINT ( 'NONE',  ( 54.22499999726881015, 149.9369285172503510, 15.58253174999999580 ) ) ;
#10161=CARTESIAN_POINT ( 'NONE',  ( 68.57499999726881867, 145.8408176439707802, 12.60653300113718345 ) ) ;
#10181=CARTESIAN_POINT ( 'NONE',  ( 78.87499999726878741, 138.6155565068815463, -3.929120461958505118E-15 ) ) ;
#10184=EDGE_CURVE ( 'NONE', #12765, #11884, #2711, .T. ) ;
#10186=CARTESIAN_POINT ( 'NONE',  ( 73.52499999726882152, 169.8198683612136222, -4.815267126137197984 ) ) ;
#10191=CARTESIAN_POINT ( 'NONE',  ( 66.72499999726881015, 140.1801316387863778, -4.815267126137194431 ) ) ;
#10205=CARTESIAN_POINT ( 'NONE',  ( 86.87499999726880162, 138.6155565068815747, -3.929120461958505118E-15 ) ) ;
#10207=CARTESIAN_POINT ( 'NONE',  ( 41.22499999726881015, 160.0630714827496206, -15.58253175000000823 ) ) ;
#10214=CARTESIAN_POINT ( 'NONE',  ( 125.5000000000000000, 157.1500000000010573, 105.9999999999999858 ) ) ;
#10218=CARTESIAN_POINT ( 'NONE',  ( 70.29999999453762882, 167.3344367211045096, -8.961492836873482304 ) ) ;
#10224=EDGE_CURVE ( 'NONE', #15702, #4983, #8369, .T. ) ;
#10231=EDGE_CURVE ( 'NONE', #3461, #18094, #6164, .T. ) ;
#10233=CARTESIAN_POINT ( 'NONE',  ( 56.08867513459481557, 142.2402378747194405, 9.270509831248432420 ) ) ;
#10237=EDGE_CURVE ( 'NONE', #32735, #5752, #26890, .T. ) ;
#10242=CARTESIAN_POINT ( 'NONE',  ( 65.17499999726881299, 145.8408176439707802, -12.60653300113719588 ) ) ;
#10247=DIRECTION ( 'NONE',  ( 0.000000000000000000, 0.000000000000000000, -1.000000000000000000 ) ) ;
#10250=CARTESIAN_POINT ( 'NONE',  ( 87.21132485994283456, 139.2280666364260071, -4.041636747397287284E-15 ) ) ;
#10255=CARTESIAN_POINT ( 'NONE',  ( 83.90000000000000568, 141.2096805137202580, 4.480746418436733158 ) ) ;
#10259=CARTESIAN_POINT ( 'NONE',  ( 64.28867513459482552, 139.2280666364260071, -4.041636747397287284E-15 ) ) ;
#10260=CARTESIAN_POINT ( 'NONE',  ( 52.97499999726881015, 140.1801316387863778, -4.815267126137194431 ) ) ;
#10263=CARTESIAN_POINT ( 'NONE',  ( 87.52499999726882152, 169.8198683612136222, -4.815267126137197984 ) ) ;
#10264=CARTESIAN_POINT ( 'NONE',  ( 78.31132485994280046, 169.2658477444273331, 4.635254915624208216 ) ) ;
#10265=CARTESIAN_POINT ( 'NONE',  ( 65.41132485994282320, 142.2402378747194405, -9.270509831248439525 ) ) ;
#10266=CARTESIAN_POINT ( 'NONE',  ( 56.39999999453762314, 168.7903194862797420, -4.480746418436745593 ) ) ;
#10268=( BOUNDED_CURVE ( )  B_SPLINE_CURVE ( 2, ( #14124, #9013, #19402, #26405, #8354, #18742, #29128, #25184, #9863, #22298, #4068 ),
 .UNSPECIFIED., .F., .F. ) 
 B_SPLINE_CURVE_WITH_KNOTS ( ( 3, 2, 2, 2, 2, 3 ),
 ( 0.08928571428571410729, 0.09285714285714277705, 0.09642857142857132191, 0.09999999999999988065, 0.1035714285714284255, 0.1071428571428569843 ),
 .UNSPECIFIED. ) 
 CURVE ( )  GEOMETRIC_REPRESENTATION_ITEM ( )  RATIONAL_B_SPLINE_CURVE ( ( 1.000000000000001110, 0.9510565162951523099, 1.000000000000000000, 0.9510565162951534202, 1.000000000000000000, 0.9510565162951534202, 1.000000000000000000, 0.9510565162951534202, 1.000000000000000000, 0.9510565162951549745, 0.9999999999999984457 ) ) 
 REPRESENTATION_ITEM ( '' )  );
#10271=CARTESIAN_POINT ( 'NONE',  ( 46.81132485994280756, 150.1262045565063659, 14.99999999999997158 ) ) ;
#10281=CARTESIAN_POINT ( 'NONE',  ( 74.77499999726880731, 140.1801316387863778, 4.815267126137185549 ) ) ;
#10285=CARTESIAN_POINT ( 'NONE',  ( 35.87499999726881583, 171.3844434931184253, -7.942151717890134290E-15 ) ) ;
#10286=VERTEX_POINT ( 'NONE', #12228 ) ;
#10287=CARTESIAN_POINT ( 'NONE',  ( 44.92499999726880588, 145.8408176439707802, -12.60653300113719588 ) ) ;
#10291=CARTESIAN_POINT ( 'NONE',  ( 46.37499999726880873, 155.0000000000000000, 15.58253174999999402 ) ) ;
#10294=DIRECTION ( 'NONE',  ( 0.000000000000000000, 1.000000000000000000, -1.290957005378097920E-14 ) ) ;
#10297=CARTESIAN_POINT ( 'NONE',  ( 67.29999999999999716, 163.5228861582408797, 11.73074641843673049 ) ) ;
#10299=CARTESIAN_POINT ( 'NONE',  ( 38.28867513459483263, 139.2280666364260071, -4.041636747397287284E-15 ) ) ;
#10301=CARTESIAN_POINT ( 'NONE',  ( 85.88867513459484826, 150.1262045565064795, 15.00000000000005507 ) ) ;
#10304=CARTESIAN_POINT ( 'NONE',  ( 72.82499999726879025, 141.7447067706911810, -9.630534252274385310 ) ) ;
#10307=CARTESIAN_POINT ( 'NONE',  ( 86.57499999726880446, 145.8408176439707802, 12.60653300113718345 ) ) ;
#10310=ORIENTED_EDGE ( 'NONE', *, *, #16236, .T. ) ;
#10319=CARTESIAN_POINT ( 'NONE',  ( 49.71132485994280614, 155.0000000000000000, -15.00000000000002487 ) ) ;
#10328=CARTESIAN_POINT ( 'NONE',  ( 84.72499999726882436, 140.1801316387863778, -4.815267126137194431 ) ) ;
#10332=CARTESIAN_POINT ( 'NONE',  ( 49.99999999999999289, 139.7537977485451393, -4.138211985947621020E-15 ) ) ;
#10336=CARTESIAN_POINT ( 'NONE',  ( 54.12499999726881583, 155.0000000000000000, 15.58253174999999402 ) ) ;
#10339=CARTESIAN_POINT ( 'NONE',  ( 57.82499999726880446, 168.2552932293087906, 9.630534252274372875 ) ) ;
#10340=CARTESIAN_POINT ( 'NONE',  ( 72.97499999726881015, 140.1801316387863778, -4.815267126137194431 ) ) ;
#10356=CARTESIAN_POINT ( 'NONE',  ( 76.37499999726881583, 155.0000000000000000, 15.58253174999999402 ) ) ;
#10360=CARTESIAN_POINT ( 'NONE',  ( 73.42499999726881299, 168.2552932293087906, -9.630534252274387086 ) ) ;
#10363=CARTESIAN_POINT ( 'NONE',  ( 62.42499999726881299, 141.7447067706911810, 9.630534252274376428 ) ) ;
#10378=CARTESIAN_POINT ( 'NONE',  ( 37.62499999726880873, 171.3844434931184253, -7.942151717890134290E-15 ) ) ;
#10380=LINE ( 'NONE', #13251, #18958 ) ;
#10381=EDGE_CURVE ( 'NONE', #22604, #15895, #19389, .T. ) ;
#10387=CARTESIAN_POINT ( 'NONE',  ( 78.39999999453763735, 168.7903194862797420, -4.480746418436745593 ) ) ;
#10393=ORIENTED_EDGE ( 'NONE', *, *, #20830, .F. ) ;
#10400=CARTESIAN_POINT ( 'NONE',  ( 56.48867513459482126, 142.2402378747194405, -9.270509831248439525 ) ) ;
#10404=CARTESIAN_POINT ( 'NONE',  ( 61.47499999726881015, 160.0630714827496206, -15.58253175000000823 ) ) ;
#10408=FACE_OUTER_BOUND ( 'NONE', #24029, .T. ) ;
#10418=CARTESIAN_POINT ( 'NONE',  ( 33.92499999726881299, 164.1591823560292198, 12.60653300113718167 ) ) ;
#10422=CARTESIAN_POINT ( 'NONE',  ( 64.58867513459482268, 146.1832212156128890, -12.13525491562423042 ) ) ;
#10423=CARTESIAN_POINT ( 'NONE',  ( 57.77499999726881441, 169.8198683612136222, -4.815267126137197984 ) ) ;
#10427=CARTESIAN_POINT ( 'NONE',  ( 42.31132485994280756, 169.2658477444273331, 4.635254915624208216 ) ) ;
#10429=CARTESIAN_POINT ( 'NONE',  ( 52.39999999453763024, 168.7903194862797420, -4.480746418436745593 ) ) ;
#10441=DIRECTION ( 'NONE',  ( 1.000000000000000000, 0.000000000000000000, 0.000000000000000000 ) ) ;
#10443=ORIENTED_EDGE ( 'NONE', *, *, #18983, .F. ) ;
#10446=CARTESIAN_POINT ( 'NONE',  ( 43.07499999726881867, 141.7447067706911810, -9.630534252274387086 ) ) ;
#10447=ORIENTED_EDGE ( 'NONE', *, *, #5025, .F. ) ;
#10448=CARTESIAN_POINT ( 'NONE',  ( 52.32499999726881157, 145.8408176439707802, 12.60653300113718345 ) ) ;
#10449=CYLINDRICAL_SURFACE ( 'NONE', #18628, 2.149999999999985256 ) ;
#10452=CARTESIAN_POINT ( 'NONE',  ( 51.77499999726881441, 169.8198683612136222, -4.815267126137197984 ) ) ;
#10457=CARTESIAN_POINT ( 'NONE',  ( 67.09999999999999432, 168.7903194862797420, 4.480746418436729606 ) ) ;
#10459=CARTESIAN_POINT ( 'NONE',  ( 38.48867513459482126, 142.2402378747194405, -9.270509831248439525 ) ) ;
#10466=CARTESIAN_POINT ( 'NONE',  ( 70.62499999726881583, 138.6155565068815463, -3.929120461958505118E-15 ) ) ;
#10467=VERTEX_POINT ( 'NONE', #25170 ) ;
#10470=CARTESIAN_POINT ( 'NONE',  ( 34.39999999453762314, 168.7903194862797420, -4.480746418436745593 ) ) ;
#10490=CARTESIAN_POINT ( 'NONE',  ( 84.82499999726880446, 141.7447067706911810, -9.630534252274385310 ) ) ;
#10491=DIRECTION ( 'NONE',  ( 0.000000000000000000, 0.000000000000000000, -1.000000000000000000 ) ) ;
#10495=CIRCLE ( 'NONE', #12640, 2.149999999999985256 ) ;
#10496=CARTESIAN_POINT ( 'NONE',  ( 46.40000000000000568, 150.2886644046228639, -14.50000000000000888 ) ) ;
#10501=CARTESIAN_POINT ( 'NONE',  ( 54.52499999726881441, 140.1801316387863778, 4.815267126137185549 ) ) ;
#10504=CARTESIAN_POINT ( 'NONE',  ( 56.92499999726881299, 145.8408176439707802, -12.60653300113719588 ) ) ;
#10505=CARTESIAN_POINT ( 'NONE',  ( 68.07499999726881867, 168.2552932293087906, 9.630534252274372875 ) ) ;
#10526=CARTESIAN_POINT ( 'NONE',  ( 72.82499999726879025, 141.7447067706911810, -9.630534252274387086 ) ) ;
#10529=CARTESIAN_POINT ( 'NONE',  ( 63.82499999726881867, 168.2552932293087906, 9.630534252274372875 ) ) ;
#10545=CARTESIAN_POINT ( 'NONE',  ( 39.62499999726880162, 171.3844434931184253, -7.942151717890134290E-15 ) ) ;
#10555=CARTESIAN_POINT ( 'NONE',  ( 78.99999999453763166, 155.0000000000000000, 14.49999999999999467 ) ) ;
#10559=CYLINDRICAL_SURFACE ( 'NONE', #8532, 15.00000000000001776 ) ;
#10564=CARTESIAN_POINT ( 'NONE',  ( 50.88867513459482694, 159.8737954434936057, -15.00000000000002665 ) ) ;
#10570=CARTESIAN_POINT ( 'NONE',  ( 64.07499999726881867, 168.2552932293087906, 9.630534252274372875 ) ) ;
#10571=ORIENTED_EDGE ( 'NONE', *, *, #32692, .T. ) ;
#10574=CARTESIAN_POINT ( 'NONE',  ( 32.50000000000000000, 155.0000000000000000, -15.00000000000002487 ) ) ;
#10578=CARTESIAN_POINT ( 'NONE',  ( 80.01132485994281751, 167.7597621252805880, -9.270509831248443078 ) ) ;
#10583=CARTESIAN_POINT ( 'NONE',  ( 84.60000000000000853, 159.7113355953771077, -14.50000000000000888 ) ) ;
#10584=CARTESIAN_POINT ( 'NONE',  ( 81.58867513459483689, 163.8167787843871110, 12.13525491562421621 ) ) ;
#10585=FACE_OUTER_BOUND ( 'NONE', #18134, .T. ) ;
#10588=CARTESIAN_POINT ( 'NONE',  ( 59.57499999726881157, 164.1591823560292198, -12.60653300113719766 ) ) ;
#10592=CARTESIAN_POINT ( 'NONE',  ( 86.82499999726879025, 141.7447067706911810, -9.630534252274385310 ) ) ;
#10593=CARTESIAN_POINT ( 'NONE',  ( 55.48867513459482836, 167.7597621252805880, 9.270509831248428867 ) ) ;
#10596=CARTESIAN_POINT ( 'NONE',  ( 61.69999999453762030, 142.6655632788954620, -8.961492836873480528 ) ) ;
#10599=CARTESIAN_POINT ( 'NONE',  ( 36.98867513459482126, 163.8167787843871110, -12.13525491562423397 ) ) ;
#10602=CARTESIAN_POINT ( 'NONE',  ( 59.61132485994281893, 150.1262045565063659, -14.99999999999998046 ) ) ;
#10607=CARTESIAN_POINT ( 'NONE',  ( 44.61132485994281893, 159.8737954434936057, 15.00000000000003730 ) ) ;
#10608=ORIENTED_EDGE ( 'NONE', *, *, #16895, .T. ) ;
#10612=CARTESIAN_POINT ( 'NONE',  ( 44.27499999726881441, 160.0630714827496206, 15.58253174999999224 ) ) ;
#10614=CARTESIAN_POINT ( 'NONE',  ( 52.02499999726880020, 160.0630714827496206, 15.58253174999999402 ) ) ;
#10619=CARTESIAN_POINT ( 'NONE',  ( 54.27499999726880020, 160.0630714827496206, 15.58253174999999402 ) ) ;
#10623=CARTESIAN_POINT ( 'NONE',  ( 66.70000000000000284, 163.5228861582408797, -11.73074641843674470 ) ) ;
#10627=CARTESIAN_POINT ( 'NONE',  ( 86.78867513459481131, 155.0000000000000000, -15.00000000000002487 ) ) ;
#10628=CARTESIAN_POINT ( 'NONE',  ( 35.17499999726881299, 145.8408176439707802, -12.60653300113719588 ) ) ;
#10630=CARTESIAN_POINT ( 'NONE',  ( 70.42499999726881299, 141.7447067706911810, 9.630534252274376428 ) ) ;
#10633=CARTESIAN_POINT ( 'NONE',  ( 41.39999999453762314, 141.2096805137202580, 4.480746418436733158 ) ) ;
#10636=EDGE_LOOP ( 'NONE', ( #27796, #3504 ) ) ;
#10645=DIRECTION ( 'NONE',  ( 0.000000000000000000, 0.7071067811865475727, 0.7071067811865475727 ) ) ;
#10651=ORIENTED_EDGE ( 'NONE', *, *, #8262, .T. ) ;
#10653=( BOUNDED_CURVE ( )  B_SPLINE_CURVE ( 2, ( #27456, #33069, #17742, #15687, #31202, #23192, #8034, #10265, #25913, #2586, #3073 ),
 .UNSPECIFIED., .F., .T. ) 
 B_SPLINE_CURVE_WITH_KNOTS ( ( 3, 2, 2, 2, 2, 3 ),
 ( 0.5535714285714283811, 0.5571428571428569398, 0.5607142857142854986, 0.5642857142857141683, 0.5678571428571427271, 0.5714285714285712858 ),
 .UNSPECIFIED. ) 
 CURVE ( )  GEOMETRIC_REPRESENTATION_ITEM ( )  RATIONAL_B_SPLINE_CURVE ( ( 1.000000000000003109, 0.9510565162951504226, 1.000000000000000000, 0.9510565162951534202, 1.000000000000000000, 0.9510565162951534202, 1.000000000000000000, 0.9510565162951534202, 1.000000000000000000, 0.9510565162951549745, 0.9999999999999984457 ) ) 
 REPRESENTATION_ITEM ( '' )  );
#10655=CARTESIAN_POINT ( 'NONE',  ( 34.37499999726881583, 155.0000000000000000, 15.58253174999999402 ) ) ;
#10656=CYLINDRICAL_SURFACE ( 'NONE', #17595, 2.149999999999985256 ) ;
#10659=CARTESIAN_POINT ( 'NONE',  ( 49.30000000000000426, 163.5228861582408797, 11.73074641843673049 ) ) ;
#10662=CARTESIAN_POINT ( 'NONE',  ( 49.92499999726881299, 164.1591823560292198, 12.60653300113718167 ) ) ;
#10665=CARTESIAN_POINT ( 'NONE',  ( 62.22499999726881015, 149.9369285172503510, 15.58253174999999580 ) ) ;
#10666=CARTESIAN_POINT ( 'NONE',  ( 68.17499999726881299, 164.1591823560292198, 12.60653300113718167 ) ) ;
#10668=CARTESIAN_POINT ( 'NONE',  ( 48.71132485994280614, 155.0000000000000000, 15.00000000000001243 ) ) ;
#10670=CARTESIAN_POINT ( 'NONE',  ( 35.58867513459482268, 163.8167787843871110, 12.13525491562421621 ) ) ;
#10679=ORIENTED_EDGE ( 'NONE', *, *, #31581, .F. ) ;
#10682=CARTESIAN_POINT ( 'NONE',  ( 78.72499999726881015, 140.1801316387863778, -4.815267126137194431 ) ) ;
#10686=CARTESIAN_POINT ( 'NONE',  ( 67.42499999726879878, 168.2552932293087906, -9.630534252274385310 ) ) ;
#10702=CARTESIAN_POINT ( 'NONE',  ( 46.28867513459482552, 139.2280666364260071, -4.041636747397287284E-15 ) ) ;
#10704=CARTESIAN_POINT ( 'NONE',  ( 44.52499999726881441, 140.1801316387863778, 4.815267126137185549 ) ) ;
#10711=CARTESIAN_POINT ( 'NONE',  ( 81.79999999453762882, 146.4771138417591203, -11.73074641843674470 ) ) ;
#10716=ORIENTED_EDGE ( 'NONE', *, *, #26464, .T. ) ;
#10718=AXIS2_PLACEMENT_3D ( 'NONE', #19425, #29323, #31707 ) ;
#10722=CARTESIAN_POINT ( 'NONE',  ( 86.78867513459481131, 155.0000000000000000, -15.00000000000002487 ) ) ;
#10728=CARTESIAN_POINT ( 'NONE',  ( 60.77499999726881441, 140.1801316387863778, 4.815267126137185549 ) ) ;
#10731=CYLINDRICAL_SURFACE ( 'NONE', #11927, 15.00000000000001776 ) ;
#10735=CARTESIAN_POINT ( 'NONE',  ( 87.31132485994280046, 140.7341522555726669, -4.635254915624220651 ) ) ;
#10737=CARTESIAN_POINT ( 'NONE',  ( 85.87499999726881583, 171.3844434931184253, -7.942151717890132712E-15 ) ) ;
#10742=CARTESIAN_POINT ( 'NONE',  ( 36.82499999726881157, 141.7447067706911810, -9.630534252274385310 ) ) ;
#10746=CARTESIAN_POINT ( 'NONE',  ( 64.68867513459485963, 150.1262045565065364, -15.00000000000012434 ) ) ;
#10747=CARTESIAN_POINT ( 'NONE',  ( 56.27499999726880020, 160.0630714827496206, 15.58253174999999402 ) ) ;
#10750=AXIS2_PLACEMENT_3D ( 'NONE', #8591, #6541, #9089 ) ;
#10754=CARTESIAN_POINT ( 'NONE',  ( 62.59999999453763309, 168.7903194862797420, 4.480746418436729606 ) ) ;
#10768=CARTESIAN_POINT ( 'NONE',  ( 44.21132485994281325, 170.7719333635740497, -7.904646289410545231E-15 ) ) ;
#10773=CARTESIAN_POINT ( 'NONE',  ( 40.97499999726881725, 140.1801316387863778, -4.815267126137194431 ) ) ;
#10776=CARTESIAN_POINT ( 'NONE',  ( 53.52499999726881441, 169.8198683612136222, -4.815267126137197984 ) ) ;
#10780=CARTESIAN_POINT ( 'NONE',  ( 52.37499999726881583, 155.0000000000000000, 15.58253174999999402 ) ) ;
#10785=CARTESIAN_POINT ( 'NONE',  ( 75.50000000000001421, 155.0000000000000000, 14.49999999999999467 ) ) ;
#10787=CARTESIAN_POINT ( 'NONE',  ( 38.18867513459482410, 140.7341522555726669, 4.635254915624211769 ) ) ;
#10790=CARTESIAN_POINT ( 'NONE',  ( 86.18867513459483121, 140.7341522555726669, 4.635254915624211769 ) ) ;
#10791=CARTESIAN_POINT ( 'NONE',  ( 40.47499999726881725, 149.9369285172503510, 15.58253174999999580 ) ) ;
#10794=CARTESIAN_POINT ( 'NONE',  ( 72.12499999726881583, 155.0000000000000000, 15.58253174999999402 ) ) ;
#10797=CARTESIAN_POINT ( 'NONE',  ( 40.89999999453763024, 159.7113355953771077, 14.49999999999999289 ) ) ;
#10808=ORIENTED_EDGE ( 'NONE', *, *, #26337, .T. ) ;
#10818=CARTESIAN_POINT ( 'NONE',  ( 34.52499999726880731, 140.1801316387863778, 4.815267126137185549 ) ) ;
#10820=CARTESIAN_POINT ( 'NONE',  ( 87.92499999726881299, 164.1591823560292198, 12.60653300113718167 ) ) ;
#10824=CARTESIAN_POINT ( 'NONE',  ( 51.00000000000000711, 170.2462022514548323, -7.872454543227099337E-15 ) ) ;
#10826=CARTESIAN_POINT ( 'NONE',  ( 84.11132485994279762, 169.2658477444273331, -4.635254915624224203 ) ) ;
#10827=ADVANCED_FACE ( 'NONE', ( #28908 ), #463, .T. ) ;
#10828=CARTESIAN_POINT ( 'NONE',  ( 51.72499999726881725, 169.8198683612136222, 4.815267126137181997 ) ) ;
#10831=CARTESIAN_POINT ( 'NONE',  ( 37.31132485994280756, 140.7341522555726669, -4.635254915624220651 ) ) ;
#10832=CARTESIAN_POINT ( 'NONE',  ( 64.82499999726881867, 141.7447067706911810, -9.630534252274387086 ) ) ;
#10833=CARTESIAN_POINT ( 'NONE',  ( 76.77499999726880731, 140.1801316387863778, 4.815267126137185549 ) ) ;
#10839=CARTESIAN_POINT ( 'NONE',  ( 85.58867513459482268, 163.8167787843871110, 12.13525491562421621 ) ) ;
#10840=ORIENTED_EDGE ( 'NONE', *, *, #15413, .T. ) ;
#10851=EDGE_LOOP ( 'NONE', ( #2768, #13759, #4344, #26480 ) ) ;
#10855=CARTESIAN_POINT ( 'NONE',  ( 80.52499999726880731, 140.1801316387863778, 4.815267126137185549 ) ) ;
#10856=CARTESIAN_POINT ( 'NONE',  ( 32.50000000000000000, 155.0000000000000000, -6.938893903907228378E-15 ) ) ;
#10857=DIRECTION ( 'NONE',  ( 0.000000000000000000, 0.000000000000000000, -1.000000000000000000 ) ) ;
#10859=CARTESIAN_POINT ( 'NONE',  ( 70.22499999726879594, 149.9369285172503510, 15.58253174999999580 ) ) ;
#10872=CARTESIAN_POINT ( 'NONE',  ( 59.88867513459482694, 150.1262045565063659, 14.99999999999997158 ) ) ;
#10873=CARTESIAN_POINT ( 'NONE',  ( 41.42499999726881299, 168.2552932293087906, -9.630534252274387086 ) ) ;
#10881=CARTESIAN_POINT ( 'NONE',  ( 76.49999999453761745, 170.2462022514548323, -7.872454543227099337E-15 ) ) ;
#10891=CARTESIAN_POINT ( 'NONE',  ( 78.07499999726881867, 168.2552932293087906, 9.630534252274372875 ) ) ;
#10896=CARTESIAN_POINT ( 'NONE',  ( 60.07499999726880446, 168.2552932293087906, 9.630534252274372875 ) ) ;
#10898=CARTESIAN_POINT ( 'NONE',  ( 35.71132485994280614, 155.0000000000000000, -15.00000000000002487 ) ) ;
#10906=CARTESIAN_POINT ( 'NONE',  ( 87.07499999726880446, 141.7447067706911810, -9.630534252274385310 ) ) ;
#10909=CARTESIAN_POINT ( 'NONE',  ( 40.82499999726880446, 141.7447067706911810, -9.630534252274385310 ) ) ;
#10914=CARTESIAN_POINT ( 'NONE',  ( 54.97499999726881015, 140.1801316387863778, -4.815267126137194431 ) ) ;
#10918=CARTESIAN_POINT ( 'NONE',  ( 55.18867513459483121, 169.2658477444273331, -4.635254915624224203 ) ) ;
#10921=CARTESIAN_POINT ( 'NONE',  ( 59.89999999453763024, 150.2886644046228639, -14.50000000000000888 ) ) ;
#10931=CARTESIAN_POINT ( 'NONE',  ( 50.21132485994281325, 170.7719333635740497, -7.904646289410545231E-15 ) ) ;
#10935=DIRECTION ( 'NONE',  ( 0.000000000000000000, 0.000000000000000000, -1.000000000000000000 ) ) ;
#10937=CARTESIAN_POINT ( 'NONE',  ( 46.57499999726881157, 145.8408176439707802, 12.60653300113718345 ) ) ;
#10938=ORIENTED_EDGE ( 'NONE', *, *, #16594, .F. ) ;
#10939=CARTESIAN_POINT ( 'NONE',  ( 49.42499999726879878, 168.2552932293087906, -9.630534252274385310 ) ) ;
#10942=CIRCLE ( 'NONE', #16365, 27.99999999999999645 ) ;
#10944=CARTESIAN_POINT ( 'NONE',  ( 56.57499999726881157, 145.8408176439707802, 12.60653300113718345 ) ) ;
#10947=CARTESIAN_POINT ( 'NONE',  ( 72.90000000000000568, 168.7903194862797420, -4.480746418436745593 ) ) ;
#10951=CARTESIAN_POINT ( 'NONE',  ( 33.18867513459482410, 169.2658477444273331, -4.635254915624224203 ) ) ;
#10952=CARTESIAN_POINT ( 'NONE',  ( 39.17499999726881299, 145.8408176439707802, -12.60653300113719588 ) ) ;
#10954=CARTESIAN_POINT ( 'NONE',  ( 75.02499999726879309, 149.9369285172503510, -15.58253175000000823 ) ) ;
#10955=ORIENTED_EDGE ( 'NONE', *, *, #33130, .F. ) ;
#10956=CARTESIAN_POINT ( 'NONE',  ( 48.31132485994280756, 169.2658477444273331, 4.635254915624208216 ) ) ;
#10957=CARTESIAN_POINT ( 'NONE',  ( 43.29999999453762172, 142.6655632788954620, 8.961492836873471646 ) ) ;
#10958=( BOUNDED_CURVE ( )  B_SPLINE_CURVE ( 2, ( #836, #21451, #8345, #23837, #29286, #19060, #11225, #3554, #5767, #16161, #29450 ),
 .UNSPECIFIED., .F., .T. ) 
 B_SPLINE_CURVE_WITH_KNOTS ( ( 3, 2, 2, 2, 2, 3 ),
 ( 0.07142857142857124420, 0.07499999999999981681, 0.07857142857142838943, 0.08214285714285696205, 0.08571428571428553467, 0.08928571428571410729 ),
 .UNSPECIFIED. ) 
 CURVE ( )  GEOMETRIC_REPRESENTATION_ITEM ( )  RATIONAL_B_SPLINE_CURVE ( ( 1.000000000000002220, 0.9510565162951514218, 1.000000000000000000, 0.9510565162951534202, 1.000000000000000000, 0.9510565162951534202, 1.000000000000000000, 0.9510565162951534202, 1.000000000000000000, 0.9510565162951545304, 0.9999999999999988898 ) ) 
 REPRESENTATION_ITEM ( '' )  );
#10959=CARTESIAN_POINT ( 'NONE',  ( 74.78867513459483973, 155.0000000000000000, -15.00000000000002487 ) ) ;
#10960=EDGE_CURVE ( 'NONE', #19681, #7672, #27260, .T. ) ;
#10976=CARTESIAN_POINT ( 'NONE',  ( 34.72499999726881015, 140.1801316387863778, -4.815267126137194431 ) ) ;
#10977=CARTESIAN_POINT ( 'NONE',  ( 87.32499999726880446, 164.1591823560292198, -12.60653300113719766 ) ) ;
#10982=CARTESIAN_POINT ( 'NONE',  ( 55.90000000000000568, 141.2096805137202580, 4.480746418436733158 ) ) ;
#10984=DIRECTION ( 'NONE',  ( 0.000000000000000000, -0.7071067811865411334, 0.7071067811865540120 ) ) ;
#10986=CARTESIAN_POINT ( 'NONE',  ( 60.32499999726881157, 145.8408176439707802, 12.60653300113718345 ) ) ;
#10990=CARTESIAN_POINT ( 'NONE',  ( 63.62499999726879452, 171.3844434931184253, -7.942151717890134290E-15 ) ) ;
#10991=CARTESIAN_POINT ( 'NONE',  ( 79.07499999726880446, 141.7447067706911810, -9.630534252274385310 ) ) ;
#10993=CARTESIAN_POINT ( 'NONE',  ( 48.81132485994281467, 150.1262045565064227, 15.00000000000001599 ) ) ;
#11001=LINE ( 'NONE', #5874, #4498 ) ;
#11013=CARTESIAN_POINT ( 'NONE',  ( 77.52499999726880731, 169.8198683612136222, -4.815267126137197984 ) ) ;
#11014=EDGE_LOOP ( 'NONE', ( #26751, #21186, #8759, #32483 ) ) ;
#11016=CARTESIAN_POINT ( 'NONE',  ( 87.50000000000001421, 155.0000000000000000, -6.938893903907228378E-15 ) ) ;
#11018=UNCERTAINTY_MEASURE_WITH_UNIT (LENGTH_MEASURE( 1.000000000000000082E-05 ), #11061, 'distance_accuracy_value', 'NONE');
#11019=CARTESIAN_POINT ( 'NONE',  ( 72.22499999726881015, 149.9369285172503510, 15.58253174999999580 ) ) ;
#11024=CARTESIAN_POINT ( 'NONE',  ( 35.00000000000000000, 170.2462022514548323, -7.872454543227099337E-15 ) ) ;
#11031=CARTESIAN_POINT ( 'NONE',  ( 72.71132485994280614, 155.0000000000000000, 15.00000000000001243 ) ) ;
#11033=CARTESIAN_POINT ( 'NONE',  ( 45.82499999726881157, 168.2552932293087906, 9.630534252274372875 ) ) ;
#11040=CARTESIAN_POINT ( 'NONE',  ( 80.69999999453764872, 167.3344367211045096, 8.961492836873468093 ) ) ;
#11047=ORIENTED_EDGE ( 'NONE', *, *, #11642, .F. ) ;
#11050=ORIENTED_EDGE ( 'NONE', *, *, #25161, .F. ) ;
#11055=CARTESIAN_POINT ( 'NONE',  ( 75.07499999726880446, 141.7447067706911810, -9.630534252274387086 ) ) ;
#11056=CARTESIAN_POINT ( 'NONE',  ( 53.21132485994280614, 139.2280666364260071, -4.041636747397287284E-15 ) ) ;
#11061=( LENGTH_UNIT ( ) NAMED_UNIT ( * ) SI_UNIT ( .MILLI., .METRE. ) );
#11063=CARTESIAN_POINT ( 'NONE',  ( 72.27499999726880731, 160.0630714827496206, 15.58253174999999224 ) ) ;
#11064=ORIENTED_EDGE ( 'NONE', *, *, #6797, .T. ) ;
#11072=CARTESIAN_POINT ( 'NONE',  ( 87.67499999726882720, 168.2552932293087906, -9.630534252274385310 ) ) ;
#11076=CARTESIAN_POINT ( 'NONE',  ( 36.22499999726881015, 149.9369285172503510, 15.58253174999999580 ) ) ;
#11081=CARTESIAN_POINT ( 'NONE',  ( 59.27499999726882152, 149.9369285172503510, -15.58253175000000823 ) ) ;
#11088=CARTESIAN_POINT ( 'NONE',  ( 62.19999999453763451, 163.5228861582408797, -11.73074641843674470 ) ) ;
#11089=VERTEX_POINT ( 'NONE', #20153 ) ;
#11091=CARTESIAN_POINT ( 'NONE',  ( 32.50000000000000000, 155.0000000000000000, -6.938893903907228378E-15 ) ) ;
#11093=CARTESIAN_POINT ( 'NONE',  ( 70.88867513459481984, 159.8737954434938047, -14.99999999999988454 ) ) ;
#11097=EDGE_LOOP ( 'NONE', ( #21265, #12398, #23330, #13643 ) ) ;
#11099=CARTESIAN_POINT ( 'NONE',  ( 50.41132485994280898, 167.7597621252805880, 9.270509831248428867 ) ) ;
#11103=( BOUNDED_CURVE ( )  B_SPLINE_CURVE ( 2, ( #16932, #25282, #30403, #22732, #4672, #6722, #27328, #3992, #1436, #14389, #24611 ),
 .UNSPECIFIED., .F., .T. ) 
 B_SPLINE_CURVE_WITH_KNOTS ( ( 3, 2, 2, 2, 2, 3 ),
 ( 0.2678571428571425717, 0.2714285714285711304, 0.2749999999999996891, 0.2785714285714281924, 0.2821428571428568621, 0.2857142857142854209 ),
 .UNSPECIFIED. ) 
 CURVE ( )  GEOMETRIC_REPRESENTATION_ITEM ( )  RATIONAL_B_SPLINE_CURVE ( ( 1.000000000000003109, 0.9510565162951504226, 1.000000000000000000, 0.9510565162951534202, 1.000000000000000000, 0.9510565162951534202, 1.000000000000000000, 0.9510565162951534202, 1.000000000000000000, 0.9510565162951571949, 0.9999999999999962252 ) ) 
 REPRESENTATION_ITEM ( '' )  );
#11106=CARTESIAN_POINT ( 'NONE',  ( 45.57499999726881157, 164.1591823560292198, -12.60653300113719766 ) ) ;
#11108=CARTESIAN_POINT ( 'NONE',  ( 51.42499999726879878, 168.2552932293087906, -9.630534252274385310 ) ) ;
#11114=CARTESIAN_POINT ( 'NONE',  ( 53.57499999726881157, 164.1591823560292198, -12.60653300113719766 ) ) ;
#11119=CARTESIAN_POINT ( 'NONE',  ( 74.20000000000000284, 142.6655632788954620, -8.961492836873480528 ) ) ;
#11125=CARTESIAN_POINT ( 'NONE',  ( 35.87499999726881583, 171.3844434931184253, -7.942151717890132712E-15 ) ) ;
#11127=CARTESIAN_POINT ( 'NONE',  ( 76.82499999726881867, 141.7447067706911810, -9.630534252274385310 ) ) ;
#11128=ORIENTED_EDGE ( 'NONE', *, *, #24533, .T. ) ;
#11130=CARTESIAN_POINT ( 'NONE',  ( 42.59999999453763309, 168.7903194862797420, 4.480746418436729606 ) ) ;
#11142=CARTESIAN_POINT ( 'NONE',  ( 51.01132485994281751, 142.2402378747194405, 9.270509831248432420 ) ) ;
#11143=ORIENTED_EDGE ( 'NONE', *, *, #31007, .F. ) ;
#11147=ORIENTED_EDGE ( 'NONE', *, *, #9298, .T. ) ;
#11149=CARTESIAN_POINT ( 'NONE',  ( 36.97499999726881015, 140.1801316387863778, -4.815267126137194431 ) ) ;
#11154=CARTESIAN_POINT ( 'NONE',  ( 51.60000000000000853, 150.2886644046228639, 14.49999999999999645 ) ) ;
#11156=CARTESIAN_POINT ( 'NONE',  ( 76.88867513459484826, 159.8737954434940036, -14.99999999999976907 ) ) ;
#11157=CARTESIAN_POINT ( 'NONE',  ( 57.22499999726879594, 160.0630714827496206, -15.58253175000000823 ) ) ;
#11160=CARTESIAN_POINT ( 'NONE',  ( 62.42499999726881299, 141.7447067706911810, 9.630534252274376428 ) ) ;
#11161=CARTESIAN_POINT ( 'NONE',  ( 77.37499999726881583, 155.0000000000000000, -15.58253175000000823 ) ) ;
#11174=CARTESIAN_POINT ( 'NONE',  ( 63.31132485994281467, 140.7341522555726669, -4.635254915624220651 ) ) ;
#11178=CARTESIAN_POINT ( 'NONE',  ( 76.22499999726881015, 149.9369285172503510, 15.58253174999999580 ) ) ;
#11181=CARTESIAN_POINT ( 'NONE',  ( 72.62499999726880162, 138.6155565068815463, -3.929120461958505118E-15 ) ) ;
#11185=CARTESIAN_POINT ( 'NONE',  ( 34.50000000000000000, 155.0000000000000000, -14.50000000000000711 ) ) ;
#11193=CARTESIAN_POINT ( 'NONE',  ( 60.68867513459482410, 150.1262045565064795, -15.00000000000007638 ) ) ;
#11194=CARTESIAN_POINT ( 'NONE',  ( 45.12499999726880873, 155.0000000000000000, -15.58253175000000823 ) ) ;
#11201=CARTESIAN_POINT ( 'NONE',  ( 88.49999999453763166, 170.2462022514548323, -7.872454543227099337E-15 ) ) ;
#11207=VERTEX_POINT ( 'NONE', #26275 ) ;
#11212=VERTEX_POINT ( 'NONE', #3101 ) ;
#11214=CARTESIAN_POINT ( 'NONE',  ( 76.67499999726881299, 141.7447067706911810, 9.630534252274376428 ) ) ;
#11219=CARTESIAN_POINT ( 'NONE',  ( 69.57499999726881867, 164.1591823560292198, -12.60653300113719766 ) ) ;
#11225=CARTESIAN_POINT ( 'NONE',  ( 83.18867513459483121, 169.2658477444273331, -4.635254915624224203 ) ) ;
#11227=CARTESIAN_POINT ( 'NONE',  ( 84.77499999726880731, 140.1801316387863778, 4.815267126137185549 ) ) ;
#11229=CARTESIAN_POINT ( 'NONE',  ( 38.42499999726879878, 141.7447067706911810, 9.630534252274376428 ) ) ;
#11234=CARTESIAN_POINT ( 'NONE',  ( 63.87499999726881583, 171.3844434931184253, -7.942151717890132712E-15 ) ) ;
#11235=EDGE_CURVE ( 'NONE', #31983, #31659, #2363, .T. ) ;
#11237=EDGE_CURVE ( 'NONE', #18787, #4684, #18672, .T. ) ;
#11241=CLOSED_SHELL ( 'NONE', ( #7017, #11794, #16560, #28032, #31880, #27094, #24780, #14327, #4389, #29519, #4299, #1189, #1835, #3287, #32040, #19966, #16623, #17611, #2488, #3536, #10827, #11861, #22629, #16812, #4358, #29170, #28471, #255, #33179, #32462, #4919, #2724, #23128, #18553, #18048, #23740, #26182, #27715, #12938, #15012, #1872, #7231, #31939, #24110, #5110, #25367, #29791, #30597, #13674, #30019, #25165, #25779, #11665, #29561, #16242, #5301, #30778, #20136, #21393, #2689, #23564, #28065, #21192, #24974, #22991, #11423, #26249, #30629, #6187, #3755, #30202, #33263, #19062, #15787, #29881, #9795, #25796, #411, #23878, #4367, #5634, #26977, #24739, #31861, #22020, #19165, #18875, #28093, #22853, #15371, #33337, #5174, #988 ) ) ;
#11242=CARTESIAN_POINT ( 'NONE',  ( 55.08867513459482268, 167.7597621252805880, -9.270509831248443078 ) ) ;
#11245=CARTESIAN_POINT ( 'NONE',  ( 63.39999999453763024, 141.2096805137202580, 4.480746418436733158 ) ) ;
#11249=EDGE_CURVE ( 'NONE', #8868, #20312, #31234, .T. ) ;
#11252=CARTESIAN_POINT ( 'NONE',  ( 58.81132485994281467, 150.1262045565064795, 15.00000000000006395 ) ) ;
#11256=EDGE_CURVE ( 'NONE', #608, #6290, #16609, .T. ) ;
#11258=CARTESIAN_POINT ( 'NONE',  ( 49.81132485994280756, 159.8737954434936057, -15.00000000000002665 ) ) ;
#11266=CARTESIAN_POINT ( 'NONE',  ( 51.77499999726881441, 169.8198683612136222, -4.815267126137197984 ) ) ;
#11268=CARTESIAN_POINT ( 'NONE',  ( 60.12499999726880873, 155.0000000000000000, 15.58253174999999402 ) ) ;
#11270=CARTESIAN_POINT ( 'NONE',  ( 61.48867513459482836, 167.7597621252805880, 9.270509831248428867 ) ) ;
#11272=DIRECTION ( 'NONE',  ( 1.000000000000000000, 0.000000000000000000, 0.000000000000000000 ) ) ;
#11274=CARTESIAN_POINT ( 'NONE',  ( 58.77499999726881441, 140.1801316387863778, 4.815267126137185549 ) ) ;
#11276=CARTESIAN_POINT ( 'NONE',  ( 73.38867513459481984, 169.2658477444273331, 4.635254915624208216 ) ) ;
#11278=CARTESIAN_POINT ( 'NONE',  ( 74.80000000000001137, 167.3344367211045096, -8.961492836873482304 ) ) ;
#11279=CARTESIAN_POINT ( 'NONE',  ( 65.18867513459481700, 169.2658477444273331, -4.635254915624224203 ) ) ;
#11280=FACE_OUTER_BOUND ( 'NONE', #2511, .T. ) ;
#11283=CARTESIAN_POINT ( 'NONE',  ( 36.27499999726880731, 160.0630714827496206, 15.58253174999999402 ) ) ;
#11285=CARTESIAN_POINT ( 'NONE',  ( 76.52499999726880731, 140.1801316387863778, 4.815267126137185549 ) ) ;
#11286=ORIENTED_EDGE ( 'NONE', *, *, #23556, .F. ) ;
#11288=CARTESIAN_POINT ( 'NONE',  ( 42.99999999453763166, 155.0000000000000000, 14.49999999999999467 ) ) ;
#11293=EDGE_LOOP ( 'NONE', ( #2388, #4943 ) ) ;
#11294=( GEOMETRIC_REPRESENTATION_CONTEXT ( 3 ) GLOBAL_UNCERTAINTY_ASSIGNED_CONTEXT ( ( #11018 ) ) GLOBAL_UNIT_ASSIGNED_CONTEXT ( ( #11061, #29617, #21443 ) ) REPRESENTATION_CONTEXT ( 'NONE', 'WORKASPACE' ) );
#11300=( BOUNDED_CURVE ( )  B_SPLINE_CURVE ( 2, ( #15824, #3044, #8488, #13268, #21103, #21268, #5755, #21597, #10722 ),
 .UNSPECIFIED., .F., .T. ) 
 B_SPLINE_CURVE_WITH_KNOTS ( ( 3, 2, 2, 2, 3 ),
 ( 0.005159801592109723549, 0.007142857142857129624, 0.01071428571428571092, 0.01428571428571429047, 0.01785714285714287350 ),
 .UNSPECIFIED. ) 
 CURVE ( )  GEOMETRIC_REPRESENTATION_ITEM ( )  RATIONAL_B_SPLINE_CURVE ( ( 0.9758271243137095485, 0.9728238588305329060, 1.000000000000000000, 0.9510565162951534202, 1.000000000000000000, 0.9510565162951534202, 1.000000000000000000, 0.9510565162951523099, 1.000000000000001110 ) ) 
 REPRESENTATION_ITEM ( '' )  );
#11303=CARTESIAN_POINT ( 'NONE',  ( 50.81132485994280756, 150.1262045565064227, 15.00000000000001599 ) ) ;
#11309=CARTESIAN_POINT ( 'NONE',  ( 38.92499999726881299, 145.8408176439707802, -12.60653300113719588 ) ) ;
#11312=CARTESIAN_POINT ( 'NONE',  ( 33.37499999726880873, 155.0000000000000000, -15.58253175000000823 ) ) ;
#11316=CARTESIAN_POINT ( 'NONE',  ( 55.99999999999999289, 139.7537977485451393, -4.138211985947621020E-15 ) ) ;
#11320=CARTESIAN_POINT ( 'NONE',  ( 56.02499999726880731, 160.0630714827496206, 15.58253174999999402 ) ) ;
#11323=CARTESIAN_POINT ( 'NONE',  ( 36.91132485994280898, 146.1832212156128890, 12.13525491562421976 ) ) ;
#11324=CARTESIAN_POINT ( 'NONE',  ( 63.22499999726881015, 160.0630714827496206, -15.58253175000000823 ) ) ;
#11325=CARTESIAN_POINT ( 'NONE',  ( 78.57499999726881867, 145.8408176439707802, 12.60653300113718345 ) ) ;
#11345=EDGE_LOOP ( 'NONE', ( #27767, #21892, #27718, #9659 ) ) ;
#11346=VECTOR ( 'NONE', #3026, 1000.000000000000000 ) ;
#11347=CARTESIAN_POINT ( 'NONE',  ( 78.12499999726883004, 155.0000000000000000, 15.58253174999999402 ) ) ;
#11349=CARTESIAN_POINT ( 'NONE',  ( 69.28867513459483973, 170.7719333635740497, -7.904646289410545231E-15 ) ) ;
#11350=CARTESIAN_POINT ( 'NONE',  ( 70.82499999726883289, 141.7447067706911810, -9.630534252274385310 ) ) ;
#11352=CARTESIAN_POINT ( 'NONE',  ( 57.81132485994280756, 159.8737954434936057, -15.00000000000002665 ) ) ;
#11354=CARTESIAN_POINT ( 'NONE',  ( 37.29999999999999716, 163.5228861582408797, 11.73074641843673049 ) ) ;
#11356=CIRCLE ( 'NONE', #23856, 2.149999999999984812 ) ;
#11365=CARTESIAN_POINT ( 'NONE',  ( 46.62499999726880873, 138.6155565068815747, -3.929120461958505118E-15 ) ) ;
#11374=CARTESIAN_POINT ( 'NONE',  ( 87.69999999453764872, 142.6655632788954620, -8.961492836873480528 ) ) ;
#11381=ORIENTED_EDGE ( 'NONE', *, *, #11235, .T. ) ;
#11382=CARTESIAN_POINT ( 'NONE',  ( 68.97499999726881015, 140.1801316387863778, -4.815267126137194431 ) ) ;
#11387=CARTESIAN_POINT ( 'NONE',  ( 75.17499999726881299, 145.8408176439707802, -12.60653300113719588 ) ) ;
#11394=CARTESIAN_POINT ( 'NONE',  ( 69.77499999726880731, 169.8198683612136222, -4.815267126137197984 ) ) ;
#11401=EDGE_CURVE ( 'NONE', #22486, #24793, #23219, .T. ) ;
#11403=CARTESIAN_POINT ( 'NONE',  ( 85.27499999726879309, 149.9369285172503510, -15.58253175000000823 ) ) ;
#11405=CARTESIAN_POINT ( 'NONE',  ( 38.52499999726881441, 140.1801316387863778, 4.815267126137185549 ) ) ;
#11406=CARTESIAN_POINT ( 'NONE',  ( 81.38867513459483405, 169.2658477444273331, 4.635254915624208216 ) ) ;
#11418=CARTESIAN_POINT ( 'NONE',  ( 64.59999999453764019, 168.7903194862797420, 4.480746418436729606 ) ) ;
#11423=ADVANCED_FACE ( 'NONE', ( #18612 ), #5492, .T. ) ;
#11424=CARTESIAN_POINT ( 'NONE',  ( 75.81132485994281467, 159.8737954434936057, -15.00000000000002665 ) ) ;
#11435=CARTESIAN_POINT ( 'NONE',  ( 49.67499999726880588, 168.2552932293087906, -9.630534252274387086 ) ) ;
#11436=ORIENTED_EDGE ( 'NONE', *, *, #27207, .T. ) ;
#11437=CARTESIAN_POINT ( 'NONE',  ( 55.82499999726880446, 168.2552932293087906, 9.630534252274372875 ) ) ;
#11442=CARTESIAN_POINT ( 'NONE',  ( 59.47499999726879594, 160.0630714827496206, -15.58253175000000823 ) ) ;
#11446=CARTESIAN_POINT ( 'NONE',  ( 74.60000000000000853, 159.7113355953771077, -14.50000000000000888 ) ) ;
#11447=CARTESIAN_POINT ( 'NONE',  ( 62.71132485994281325, 155.0000000000000000, 15.00000000000001243 ) ) ;
#11451=CARTESIAN_POINT ( 'NONE',  ( 47.07499999726880446, 141.7447067706911810, -9.630534252274385310 ) ) ;
#11453=CARTESIAN_POINT ( 'NONE',  ( 74.02499999726879309, 160.0630714827496206, 15.58253174999999402 ) ) ;
#11454=VERTEX_POINT ( 'NONE', #24555 ) ;
#11456=CARTESIAN_POINT ( 'NONE',  ( 47.09999999453762598, 150.2886644046228639, 14.49999999999999645 ) ) ;
#11470=AXIS2_PLACEMENT_3D ( 'NONE', #3380, #18887, #1164 ) ;
#11476=DIRECTION ( 'NONE',  ( 0.000000000000000000, 0.000000000000000000, -1.000000000000000000 ) ) ;
#11478=CARTESIAN_POINT ( 'NONE',  ( 40.32499999726881157, 145.8408176439707802, 12.60653300113718345 ) ) ;
#11480=CARTESIAN_POINT ( 'NONE',  ( 42.97499999726881015, 140.1801316387863778, -4.815267126137194431 ) ) ;
#11483=EDGE_CURVE ( 'NONE', #20312, #9970, #15324, .T. ) ;
#11484=CARTESIAN_POINT ( 'NONE',  ( 57.10000000000000142, 168.7903194862797420, 4.480746418436729606 ) ) ;
#11485=CARTESIAN_POINT ( 'NONE',  ( 63.18867513459480989, 169.2658477444273331, -4.635254915624224203 ) ) ;
#11487=CARTESIAN_POINT ( 'NONE',  ( 65.78867513459482552, 155.0000000000000000, 15.00000000000001243 ) ) ;
#11489=CARTESIAN_POINT ( 'NONE',  ( 54.62499999726880162, 138.6155565068815463, -3.929120461958505118E-15 ) ) ;
#11493=AXIS2_PLACEMENT_3D ( 'NONE', #3184, #13575, #27316 ) ;
#11494=CARTESIAN_POINT ( 'NONE',  ( 68.02499999726880731, 160.0630714827496206, 15.58253174999999224 ) ) ;
#11495=CARTESIAN_POINT ( 'NONE',  ( 75.77499999726880731, 169.8198683612136222, -4.815267126137197984 ) ) ;
#11499=ORIENTED_EDGE ( 'NONE', *, *, #14170, .T. ) ;
#11508=CARTESIAN_POINT ( 'NONE',  ( 62.91132485994280188, 146.1832212156128890, 12.13525491562421976 ) ) ;
#11513=CARTESIAN_POINT ( 'NONE',  ( 86.92499999726881299, 145.8408176439707802, -12.60653300113719588 ) ) ;
#11517=CARTESIAN_POINT ( 'NONE',  ( 78.02499999726879309, 160.0630714827496206, 15.58253174999999402 ) ) ;
#11521=CARTESIAN_POINT ( 'NONE',  ( 34.10000000000000142, 141.2096805137202580, -4.480746418436742040 ) ) ;
#11528=CARTESIAN_POINT ( 'NONE',  ( 50.02499999726880020, 160.0630714827496206, 15.58253174999999224 ) ) ;
#11529=( BOUNDED_CURVE ( )  B_SPLINE_CURVE ( 2, ( #18489, #5369, #28871, #33657, #10826, #21201, #21362, #5529, #8261, #2984, #20878 ),
 .UNSPECIFIED., .F., .T. ) 
 B_SPLINE_CURVE_WITH_KNOTS ( ( 3, 2, 2, 2, 2, 3 ),
 ( 0.8928571428571429047, 0.8964285714285714635, 0.9000000000000000222, 0.9035714285714286920, 0.9071428571428572507, 0.9107142857142858094 ),
 .UNSPECIFIED. ) 
 CURVE ( )  GEOMETRIC_REPRESENTATION_ITEM ( )  RATIONAL_B_SPLINE_CURVE ( ( 1.000000000000000000, 0.9510565162951534202, 1.000000000000000000, 0.9510565162951534202, 1.000000000000000000, 0.9510565162951534202, 1.000000000000000000, 0.9510565162951534202, 1.000000000000000000, 0.9510565162951518658, 1.000000000000001554 ) ) 
 REPRESENTATION_ITEM ( '' )  );
#11536=CARTESIAN_POINT ( 'NONE',  ( 86.59999999453762598, 168.7903194862797420, 4.480746418436729606 ) ) ;
#11543=VERTEX_POINT ( 'NONE', #18777 ) ;
#11544=CARTESIAN_POINT ( 'NONE',  ( 73.77499999726882152, 169.8198683612136222, -4.815267126137197984 ) ) ;
#11546=ORIENTED_EDGE ( 'NONE', *, *, #8965, .T. ) ;
#11547=CARTESIAN_POINT ( 'NONE',  ( 85.47499999726881015, 160.0630714827496206, -15.58253175000000823 ) ) ;
#11553=CARTESIAN_POINT ( 'NONE',  ( 70.57499999726881867, 145.8408176439707802, 12.60653300113718345 ) ) ;
#11567=CARTESIAN_POINT ( 'NONE',  ( 46.42499999726880588, 141.7447067706911810, 9.630534252274376428 ) ) ;
#11568=CARTESIAN_POINT ( 'NONE',  ( 35.98867513459482126, 146.1832212156128890, 12.13525491562421976 ) ) ;
#11578=CARTESIAN_POINT ( 'NONE',  ( 63.99999999453763166, 155.0000000000000000, -14.50000000000000711 ) ) ;
#11584=CARTESIAN_POINT ( 'NONE',  ( 32.50000000000000000, 155.0000000000000000, -6.938893903907228378E-15 ) ) ;
#11585=ORIENTED_EDGE ( 'NONE', *, *, #26380, .T. ) ;
#11586=CIRCLE ( 'NONE', #30635, 2.149999999999984812 ) ;
#11595=LINE ( 'NONE', #3919, #14515 ) ;
#11598=CARTESIAN_POINT ( 'NONE',  ( 49.57499999726881157, 164.1591823560292198, -12.60653300113719766 ) ) ;
#11600=CARTESIAN_POINT ( 'NONE',  ( 59.32499999726881157, 164.1591823560292198, -12.60653300113719766 ) ) ;
#11605=CARTESIAN_POINT ( 'NONE',  ( 62.77499999726882152, 140.1801316387863778, 4.815267126137185549 ) ) ;
#11607=CARTESIAN_POINT ( 'NONE',  ( 73.68867513459484542, 159.8737954434932647, 15.00000000000027001 ) ) ;
#11608=EDGE_CURVE ( 'NONE', #18797, #24401, #25782, .T. ) ;
#11611=CARTESIAN_POINT ( 'NONE',  ( 82.10000000000000853, 141.2096805137202580, -4.480746418436742040 ) ) ;
#11613=CYLINDRICAL_SURFACE ( 'NONE', #31649, 98.00000000000000000 ) ;
#11617=CARTESIAN_POINT ( 'NONE',  ( 41.47499999726880304, 160.0630714827496206, -15.58253175000000823 ) ) ;
#11620=CARTESIAN_POINT ( 'NONE',  ( 79.52499999726880731, 169.8198683612136222, -4.815267126137197984 ) ) ;
#11622=ORIENTED_EDGE ( 'NONE', *, *, #32787, .T. ) ;
#11626=CARTESIAN_POINT ( 'NONE',  ( 48.19999999453762740, 163.5228861582408797, -11.73074641843674470 ) ) ;
#11639=FACE_OUTER_BOUND ( 'NONE', #29563, .T. ) ;
#11642=EDGE_CURVE ( 'NONE', #19014, #26053, #30760, .T. ) ;
#11643=DIRECTION ( 'NONE',  ( 1.000000000000000000, 0.000000000000000000, 0.000000000000000000 ) ) ;
#11647=CARTESIAN_POINT ( 'NONE',  ( 36.32499999726881157, 145.8408176439707802, 12.60653300113718345 ) ) ;
#11650=AXIS2_PLACEMENT_3D ( 'NONE', #29778, #16150, #3540 ) ;
#11651=CARTESIAN_POINT ( 'NONE',  ( 41.07499999726881157, 141.7447067706911810, -9.630534252274385310 ) ) ;
#11654=CARTESIAN_POINT ( 'NONE',  ( 52.20000000000000284, 142.6655632788954620, -8.961492836873480528 ) ) ;
#11655=CARTESIAN_POINT ( 'NONE',  ( 62.98867513459482836, 163.8167787843871110, -12.13525491562423397 ) ) ;
#11659=CARTESIAN_POINT ( 'NONE',  ( 57.82499999726879736, 168.2552932293087906, 9.630534252274372875 ) ) ;
#11661=ORIENTED_EDGE ( 'NONE', *, *, #27899, .F. ) ;
#11663=CARTESIAN_POINT ( 'NONE',  ( 83.67499999726884141, 168.2552932293087906, -9.630534252274385310 ) ) ;
#11665=ADVANCED_FACE ( 'NONE', ( #4098 ), #32716, .T. ) ;
#11667=CARTESIAN_POINT ( 'NONE',  ( 127.5000000000000000, 155.0000000000000000, -100.0000000000000284 ) ) ;
#11675=EDGE_CURVE ( 'NONE', #17109, #317, #27906, .T. ) ;
#11679=ORIENTED_EDGE ( 'NONE', *, *, #2441, .F. ) ;
#11684=CARTESIAN_POINT ( 'NONE',  ( 85.02499999726880731, 149.9369285172503510, -15.58253175000000823 ) ) ;
#11686=CARTESIAN_POINT ( 'NONE',  ( 69.61132485994282604, 150.1262045565062806, -14.99999999999993072 ) ) ;
#11688=CARTESIAN_POINT ( 'NONE',  ( 74.42499999726881299, 141.7447067706911810, 9.630534252274376428 ) ) ;
#11689=DIRECTION ( 'NONE',  ( 0.000000000000000000, 0.000000000000000000, -1.000000000000000000 ) ) ;
#11693=CARTESIAN_POINT ( 'NONE',  ( 34.30000000000000426, 146.4771138417591203, -11.73074641843674470 ) ) ;
#11699=CARTESIAN_POINT ( 'NONE',  ( 52.72499999726881015, 140.1801316387863778, -4.815267126137194431 ) ) ;
#11701=DIRECTION ( 'NONE',  ( 0.000000000000000000, 0.000000000000000000, -1.000000000000000000 ) ) ;
#11706=CARTESIAN_POINT ( 'NONE',  ( 84.69999999453763451, 167.3344367211045096, 8.961492836873468093 ) ) ;
#11710=DIRECTION ( 'NONE',  ( 0.000000000000000000, 0.000000000000000000, -1.000000000000000000 ) ) ;
#11714=CARTESIAN_POINT ( 'NONE',  ( 74.77499999726880731, 140.1801316387863778, 4.815267126137185549 ) ) ;
#11716=ORIENTED_EDGE ( 'NONE', *, *, #2237, .F. ) ;
#11717=CARTESIAN_POINT ( 'NONE',  ( 82.37499999726881583, 155.0000000000000000, 15.58253174999999402 ) ) ;
#11723=CARTESIAN_POINT ( 'NONE',  ( 71.47499999726881015, 160.0630714827496206, -15.58253175000000823 ) ) ;
#11724=ORIENTED_EDGE ( 'NONE', *, *, #25101, .F. ) ;
#11727=( BOUNDED_CURVE ( )  B_SPLINE_CURVE ( 2, ( #15389, #23890, #17956, #5497, #31561, #20836, #12834, #28346, #23724, #2789, #26442 ),
 .UNSPECIFIED., .F., .T. ) 
 B_SPLINE_CURVE_WITH_KNOTS ( ( 3, 2, 2, 2, 2, 3 ),
 ( 0.5357142857142856984, 0.5392857142857143682, 0.5428571428571428159, 0.5464285714285713746, 0.5499999999999998224, 0.5535714285714284921 ),
 .UNSPECIFIED. ) 
 CURVE ( )  GEOMETRIC_REPRESENTATION_ITEM ( )  RATIONAL_B_SPLINE_CURVE ( ( 0.9999999999999984457, 0.9510565162951549745, 1.000000000000000000, 0.9510565162951534202, 1.000000000000000000, 0.9510565162951534202, 1.000000000000000000, 0.9510565162951534202, 1.000000000000000000, 0.9510565162951549745, 0.9999999999999984457 ) ) 
 REPRESENTATION_ITEM ( '' )  );
#11731=CARTESIAN_POINT ( 'NONE',  ( 38.11132485994280472, 169.2658477444273331, -4.635254915624224203 ) ) ;
#11733=CARTESIAN_POINT ( 'NONE',  ( 44.02499999726881441, 160.0630714827496206, 15.58253174999999402 ) ) ;
#11735=CARTESIAN_POINT ( 'NONE',  ( 34.22499999726881015, 149.9369285172503510, 15.58253174999999580 ) ) ;
#11740=LINE ( 'NONE', #16850, #25771 ) ;
#11741=LINE ( 'NONE', #6632, #12509 ) ;
#11744=CARTESIAN_POINT ( 'NONE',  ( 65.79999999453762882, 146.4771138417591203, -11.73074641843674470 ) ) ;
#11755=CARTESIAN_POINT ( 'NONE',  ( 41.88867513459481984, 150.1262045565064227, 15.00000000000001599 ) ) ;
#11759=CARTESIAN_POINT ( 'NONE',  ( 54.71132485994280614, 155.0000000000000000, 15.00000000000001243 ) ) ;
#11761=CARTESIAN_POINT ( 'NONE',  ( 53.17499999726881299, 145.8408176439707802, -12.60653300113719588 ) ) ;
#11767=CARTESIAN_POINT ( 'NONE',  ( 57.77499999726881441, 169.8198683612136222, -4.815267126137197984 ) ) ;
#11769=CARTESIAN_POINT ( 'NONE',  ( 47.78867513459482552, 155.0000000000000000, 15.00000000000001243 ) ) ;
#11773=CARTESIAN_POINT ( 'NONE',  ( 80.69999999999998863, 163.5228861582408797, -11.73074641843674470 ) ) ;
#11778=CARTESIAN_POINT ( 'NONE',  ( 42.37499999726881583, 155.0000000000000000, 15.58253174999999402 ) ) ;
#11782=CARTESIAN_POINT ( 'NONE',  ( 80.42499999726879878, 141.7447067706911810, 9.630534252274376428 ) ) ;
#11785=CARTESIAN_POINT ( 'NONE',  ( 45.59999999453762598, 141.2096805137202580, -4.480746418436742040 ) ) ;
#11786=ORIENTED_EDGE ( 'NONE', *, *, #744, .T. ) ;
#11788=CARTESIAN_POINT ( 'NONE',  ( 66.31132485994281467, 169.2658477444273331, 4.635254915624208216 ) ) ;
#11789=ORIENTED_EDGE ( 'NONE', *, *, #12023, .T. ) ;
#11794=ADVANCED_FACE ( 'NONE', ( #27445 ), #24888, .F. ) ;
#11799=ORIENTED_EDGE ( 'NONE', *, *, #8695, .T. ) ;
#11806=EDGE_LOOP ( 'NONE', ( #29369, #7928, #25003, #31462 ) ) ;
#11807=CARTESIAN_POINT ( 'NONE',  ( 36.72499999726881015, 140.1801316387863778, -4.815267126137194431 ) ) ;
#11812=CARTESIAN_POINT ( 'NONE',  ( 43.37499999726881583, 155.0000000000000000, -15.58253175000000823 ) ) ;
#11816=CARTESIAN_POINT ( 'NONE',  ( 60.30000000000000426, 146.4771138417591203, -11.73074641843674470 ) ) ;
#11817=CARTESIAN_POINT ( 'NONE',  ( 62.88867513459482694, 159.8737954434937478, -14.99999999999993072 ) ) ;
#11819=VECTOR ( 'NONE', #27769, 1000.000000000000000 ) ;
#11820=CARTESIAN_POINT ( 'NONE',  ( 76.98867513459481415, 163.8167787843871110, -12.13525491562423397 ) ) ;
#11823=CARTESIAN_POINT ( 'NONE',  ( 66.32499999726881867, 145.8408176439707802, 12.60653300113718345 ) ) ;
#11829=CARTESIAN_POINT ( 'NONE',  ( 85.17499999726882720, 145.8408176439707802, -12.60653300113719588 ) ) ;
#11832=DIRECTION ( 'NONE',  ( 0.000000000000000000, -0.7071067811865506814, -0.7071067811865442421 ) ) ;
#11838=FACE_OUTER_BOUND ( 'NONE', #30847, .T. ) ;
#11842=CARTESIAN_POINT ( 'NONE',  ( 63.71132485994279904, 155.0000000000000000, -15.00000000000002487 ) ) ;
#11843=ORIENTED_EDGE ( 'NONE', *, *, #14170, .F. ) ;
#11850=CARTESIAN_POINT ( 'NONE',  ( 85.42499999726879878, 168.2552932293087906, -9.630534252274387086 ) ) ;
#11852=CARTESIAN_POINT ( 'NONE',  ( 69.68867513459484542, 159.8737954434934352, 15.00000000000015277 ) ) ;
#11853=CARTESIAN_POINT ( 'NONE',  ( 78.72499999726881015, 140.1801316387863778, -4.815267126137194431 ) ) ;
#11859=CARTESIAN_POINT ( 'NONE',  ( 39.10000000000000142, 168.7903194862797420, 4.480746418436729606 ) ) ;
#11861=ADVANCED_FACE ( 'NONE', ( #31349 ), #23178, .T. ) ;
#11863=CARTESIAN_POINT ( 'NONE',  ( 73.11132485994281183, 140.7341522555726669, 4.635254915624211769 ) ) ;
#11865=CARTESIAN_POINT ( 'NONE',  ( 54.02499999726880731, 160.0630714827496206, 15.58253174999999224 ) ) ;
#11866=CARTESIAN_POINT ( 'NONE',  ( 65.47499999726881015, 160.0630714827496206, -15.58253175000000823 ) ) ;
#11869=AXIS2_PLACEMENT_3D ( 'NONE', #8676, #5619, #26904 ) ;
#11870=EDGE_CURVE ( 'NONE', #28642, #5515, #507, .T. ) ;
#11876=CARTESIAN_POINT ( 'NONE',  ( 86.69999999453762030, 167.3344367211045096, 8.961492836873468093 ) ) ;
#11884=VERTEX_POINT ( 'NONE', #7852 ) ;
#11885=CARTESIAN_POINT ( 'NONE',  ( 69.87499999726880162, 171.3844434931184253, -7.942151717890132712E-15 ) ) ;
#11888=CARTESIAN_POINT ( 'NONE',  ( 83.57499999726880446, 164.1591823560292198, -12.60653300113719766 ) ) ;
#11889=DIRECTION ( 'NONE',  ( 1.000000000000000000, 0.000000000000000000, 0.000000000000000000 ) ) ;
#11900=CARTESIAN_POINT ( 'NONE',  ( 86.71132485994282035, 155.0000000000000000, 15.00000000000001243 ) ) ;
#11903=EDGE_CURVE ( 'NONE', #17109, #7326, #25899, .T. ) ;
#11905=CARTESIAN_POINT ( 'NONE',  ( 71.61132485994279762, 150.1262045565062806, -14.99999999999993072 ) ) ;
#11909=CARTESIAN_POINT ( 'NONE',  ( 46.82499999726880446, 141.7447067706911810, -9.630534252274385310 ) ) ;
#11910=CARTESIAN_POINT ( 'NONE',  ( 87.50000000000000000, 154.3213600469173912, -15.33101506908378475 ) ) ;
#11915=LINE ( 'NONE', #6467, #9989 ) ;
#11919=CARTESIAN_POINT ( 'NONE',  ( 69.59999999453762598, 141.2096805137202580, -4.480746418436742040 ) ) ;
#11925=CARTESIAN_POINT ( 'NONE',  ( 76.41132485994280898, 167.7597621252805880, 9.270509831248428867 ) ) ;
#11926=EDGE_LOOP ( 'NONE', ( #13475, #11786, #9251, #13878 ) ) ;
#11927=AXIS2_PLACEMENT_3D ( 'NONE', #5275, #13116, #10247 ) ;
#11931=CARTESIAN_POINT ( 'NONE',  ( 87.50000000000000000, 160.9457742543943652, -14.40357817542362540 ) ) ;
#11937=CARTESIAN_POINT ( 'NONE',  ( 50.77499999726880731, 140.1801316387863778, 4.815267126137185549 ) ) ;
#11941=DIRECTION ( 'NONE',  ( 0.000000000000000000, 0.000000000000000000, 1.000000000000000000 ) ) ;
#11945=CARTESIAN_POINT ( 'NONE',  ( 61.27499999726882152, 149.9369285172503510, -15.58253175000000823 ) ) ;
#11950=CARTESIAN_POINT ( 'NONE',  ( 80.39999999999999147, 150.2886644046228639, -14.50000000000000888 ) ) ;
#11954=CARTESIAN_POINT ( 'NONE',  ( 42.97499999726881015, 140.1801316387863778, -4.815267126137194431 ) ) ;
#11956=CARTESIAN_POINT ( 'NONE',  ( 86.12499999726881583, 155.0000000000000000, 15.58253174999999402 ) ) ;
#11957=CARTESIAN_POINT ( 'NONE',  ( 45.78867513459482552, 155.0000000000000000, 15.00000000000001243 ) ) ;
#11958=CARTESIAN_POINT ( 'NONE',  ( 46.89999999453763024, 159.7113355953771077, 14.49999999999999289 ) ) ;
#11961=DIRECTION ( 'NONE',  ( 0.000000000000000000, 0.000000000000000000, -1.000000000000000000 ) ) ;
#11962=CARTESIAN_POINT ( 'NONE',  ( 65.71132485994280614, 155.0000000000000000, -15.00000000000002487 ) ) ;
#11975=CARTESIAN_POINT ( 'NONE',  ( 35.52499999726880731, 169.8198683612136222, -4.815267126137197984 ) ) ;
#11977=DIRECTION ( 'NONE',  ( 0.000000000000000000, -1.000000000000000000, 0.000000000000000000 ) ) ;
#11979=CARTESIAN_POINT ( 'NONE',  ( 38.47499999726881015, 149.9369285172503510, 15.58253174999999580 ) ) ;
#11982=CARTESIAN_POINT ( 'NONE',  ( 58.31132485994280046, 169.2658477444273331, 4.635254915624208216 ) ) ;
#11983=CARTESIAN_POINT ( 'NONE',  ( 61.50000000000000000, 155.0000000000000000, 14.49999999999999467 ) ) ;
#11984=CARTESIAN_POINT ( 'NONE',  ( 63.81132485994282888, 159.8737954434934920, -15.00000000000012434 ) ) ;
#11986=LINE ( 'NONE', #12499, #9663 ) ;
#11989=EDGE_CURVE ( 'NONE', #14208, #16104, #7479, .T. ) ;
#11990=CARTESIAN_POINT ( 'NONE',  ( 64.32499999726881867, 145.8408176439707802, 12.60653300113718345 ) ) ;
#11994=CARTESIAN_POINT ( 'NONE',  ( 82.77499999726880731, 140.1801316387863778, 4.815267126137185549 ) ) ;
#12004=CARTESIAN_POINT ( 'NONE',  ( 65.78867513459482552, 155.0000000000000000, 15.00000000000001243 ) ) ;
#12011=CARTESIAN_POINT ( 'NONE',  ( 82.22499999726881015, 149.9369285172503510, 15.58253174999999580 ) ) ;
#12012=ORIENTED_EDGE ( 'NONE', *, *, #344, .F. ) ;
#12013=CARTESIAN_POINT ( 'NONE',  ( 69.08867513459482268, 167.7597621252805880, -9.270509831248443078 ) ) ;
#12015=CARTESIAN_POINT ( 'NONE',  ( 77.52499999726880731, 169.8198683612136222, -4.815267126137197984 ) ) ;
#12018=CARTESIAN_POINT ( 'NONE',  ( 87.50000000000000000, 170.2392927197263361, -2.713135339554590519 ) ) ;
#12019=AXIS2_PLACEMENT_3D ( 'NONE', #2857, #32421, #9086 ) ;
#12021=CARTESIAN_POINT ( 'NONE',  ( 41.89999999999999858, 141.2096805137202580, 4.480746418436733158 ) ) ;
#12023=EDGE_CURVE ( 'NONE', #24797, #28445, #10958, .T. ) ;
#12027=CARTESIAN_POINT ( 'NONE',  ( 50.92499999726880588, 145.8408176439707802, -12.60653300113719588 ) ) ;
#12028=CARTESIAN_POINT ( 'NONE',  ( 61.97499999726881015, 169.8198683612136222, 4.815267126137181997 ) ) ;
#12036=LINE ( 'NONE', #27711, #19916 ) ;
#12037=( BOUNDED_CURVE ( )  B_SPLINE_CURVE ( 2, ( #2362, #3022, #2862, #18203, #12753, #10702, #4913, #18030, #28759, #2533, #33532 ),
 .UNSPECIFIED., .F., .T. ) 
 B_SPLINE_CURVE_WITH_KNOTS ( ( 3, 2, 2, 2, 2, 3 ),
 ( 0.7321428571428569843, 0.7357142857142855430, 0.7392857142857141017, 0.7428571428571425495, 0.7464285714285712192, 0.7499999999999997780 ),
 .UNSPECIFIED. ) 
 CURVE ( )  GEOMETRIC_REPRESENTATION_ITEM ( )  RATIONAL_B_SPLINE_CURVE ( ( 1.000000000000001554, 0.9510565162951518658, 1.000000000000000000, 0.9510565162951534202, 1.000000000000000000, 0.9510565162951534202, 1.000000000000000000, 0.9510565162951534202, 1.000000000000000000, 0.9510565162951564178, 0.9999999999999970024 ) ) 
 REPRESENTATION_ITEM ( '' )  );
#12042=ORIENTED_EDGE ( 'NONE', *, *, #28275, .F. ) ;
#12046=CARTESIAN_POINT ( 'NONE',  ( 71.97499999726881015, 169.8198683612136222, 4.815267126137181997 ) ) ;
#12050=CARTESIAN_POINT ( 'NONE',  ( 86.17499999726881299, 164.1591823560292198, 12.60653300113718167 ) ) ;
#12069=CARTESIAN_POINT ( 'NONE',  ( 43.82499999726881157, 168.2552932293087906, 9.630534252274372875 ) ) ;
#12071=CARTESIAN_POINT ( 'NONE',  ( 87.50000000000004263, 146.7973767059698957, -12.63337674179619974 ) ) ;
#12080=CARTESIAN_POINT ( 'NONE',  ( 68.09999999453764019, 159.7113355953771077, -14.50000000000000888 ) ) ;
#12085=EDGE_CURVE ( 'NONE', #11089, #27429, #17931, .T. ) ;
#12087=EDGE_CURVE ( 'NONE', #7020, #3486, #8368, .T. ) ;
#12091=ORIENTED_EDGE ( 'NONE', *, *, #15560, .T. ) ;
#12093=FACE_OUTER_BOUND ( 'NONE', #3629, .T. ) ;
#12095=CYLINDRICAL_SURFACE ( 'NONE', #27967, 15.00000000000001776 ) ;
#12096=ORIENTED_EDGE ( 'NONE', *, *, #7853, .F. ) ;
#12099=FACE_OUTER_BOUND ( 'NONE', #23332, .T. ) ;
#12101=CARTESIAN_POINT ( 'NONE',  ( 59.77499999726881441, 169.8198683612136222, -4.815267126137197984 ) ) ;
#12109=CARTESIAN_POINT ( 'NONE',  ( 63.37499999726880873, 155.0000000000000000, -15.58253175000000823 ) ) ;
#12115=CARTESIAN_POINT ( 'NONE',  ( 81.20000000000000284, 167.3344367211045096, 8.961492836873468093 ) ) ;
#12120=CARTESIAN_POINT ( 'NONE',  ( 44.17499999726881299, 164.1591823560292198, 12.60653300113718167 ) ) ;
#12122=CARTESIAN_POINT ( 'NONE',  ( 80.52499999726880731, 140.1801316387863778, 4.815267126137185549 ) ) ;
#12124=FACE_OUTER_BOUND ( 'NONE', #21942, .T. ) ;
#12125=CARTESIAN_POINT ( 'NONE',  ( 47.89999999453762314, 150.2886644046228639, -14.50000000000000888 ) ) ;
#12130=CARTESIAN_POINT ( 'NONE',  ( 66.21132485994282035, 170.7719333635740497, -7.904646289410545231E-15 ) ) ;
#12135=CIRCLE ( 'NONE', #28459, 2.149999999999974598 ) ;
#12142=CARTESIAN_POINT ( 'NONE',  ( 35.47499999726880304, 160.0630714827496206, -15.58253175000000823 ) ) ;
#12143=ORIENTED_EDGE ( 'NONE', *, *, #32617, .F. ) ;
#12144=CARTESIAN_POINT ( 'NONE',  ( 44.52499999726881441, 140.1801316387863778, 4.815267126137185549 ) ) ;
#12148=CARTESIAN_POINT ( 'NONE',  ( 41.27499999726880731, 149.9369285172503510, -15.58253175000000823 ) ) ;
#12154=CARTESIAN_POINT ( 'NONE',  ( 62.50000000000000000, 155.0000000000000000, -14.50000000000000711 ) ) ;
#12163=CARTESIAN_POINT ( 'NONE',  ( 62.12499999726880873, 155.0000000000000000, 15.58253174999999402 ) ) ;
#12167=CARTESIAN_POINT ( 'NONE',  ( 82.47499999726881015, 149.9369285172503510, 15.58253174999999580 ) ) ;
#12169=DIRECTION ( 'NONE',  ( -1.000000000000000000, -0.000000000000000000, -0.000000000000000000 ) ) ;
#12184=ORIENTED_EDGE ( 'NONE', *, *, #19308, .T. ) ;
#12186=CARTESIAN_POINT ( 'NONE',  ( 34.21132485994281325, 170.7719333635740497, -7.904646289410545231E-15 ) ) ;
#12187=ORIENTED_EDGE ( 'NONE', *, *, #537, .T. ) ;
#12189=CARTESIAN_POINT ( 'NONE',  ( 76.22499999726882436, 149.9369285172503510, 15.58253174999999580 ) ) ;
#12191=( BOUNDED_CURVE ( )  B_SPLINE_CURVE ( 2, ( #12312, #7207, #19647, #29874, #3970, #24763, #6533, #30544, #30379, #1746, #22708 ),
 .UNSPECIFIED., .F., .F. ) 
 B_SPLINE_CURVE_WITH_KNOTS ( ( 3, 2, 2, 2, 2, 3 ),
 ( 0.8571428571428570953, 0.8607142857142856540, 0.8642857142857142128, 0.8678571428571427715, 0.8714285714285714413, 0.8750000000000000000 ),
 .UNSPECIFIED. ) 
 CURVE ( )  GEOMETRIC_REPRESENTATION_ITEM ( )  RATIONAL_B_SPLINE_CURVE ( ( 1.000000000000000000, 0.9510565162951534202, 1.000000000000000000, 0.9510565162951534202, 1.000000000000000000, 0.9510565162951534202, 1.000000000000000000, 0.9510565162951534202, 1.000000000000000000, 0.9510565162951534202, 1.000000000000000000 ) ) 
 REPRESENTATION_ITEM ( '' )  );
#12193=CARTESIAN_POINT ( 'NONE',  ( 87.50000000000005684, 169.5031880795791324, 4.588213833768849170 ) ) ;
#12195=CARTESIAN_POINT ( 'NONE',  ( 44.19999999999999574, 142.6655632788954620, -8.961492836873480528 ) ) ;
#12200=CARTESIAN_POINT ( 'NONE',  ( 49.62499999726880873, 171.3844434931184253, -7.942151717890134290E-15 ) ) ;
#12201=CARTESIAN_POINT ( 'NONE',  ( 63.97499999726881725, 169.8198683612136222, 4.815267126137181997 ) ) ;
#12203=CARTESIAN_POINT ( 'NONE',  ( 40.91132485994280188, 146.1832212156128890, 12.13525491562421976 ) ) ;
#12217=CARTESIAN_POINT ( 'NONE',  ( 75.57499999726881867, 164.1591823560292198, -12.60653300113719766 ) ) ;
#12221=CARTESIAN_POINT ( 'NONE',  ( 86.27499999726880731, 160.0630714827496206, 15.58253174999999224 ) ) ;
#12224=CARTESIAN_POINT ( 'NONE',  ( 54.12499999726881583, 155.0000000000000000, 15.58253174999999402 ) ) ;
#12228=CARTESIAN_POINT ( 'NONE',  ( 44.71132485994280614, 155.0000000000000000, 15.00000000000001243 ) ) ;
#12231=LINE ( 'NONE', #20069, #28358 ) ;
#12238=CARTESIAN_POINT ( 'NONE',  ( 44.62499999726880873, 138.6155565068815463, -3.929120461958505118E-15 ) ) ;
#12240=CARTESIAN_POINT ( 'NONE',  ( 125.5000000000000000, 155.0000000000000000, 112.0000000000000711 ) ) ;
#12250=CARTESIAN_POINT ( 'NONE',  ( 71.79999999453762882, 146.4771138417591203, -11.73074641843674470 ) ) ;
#12251=EDGE_LOOP ( 'NONE', ( #12143, #10679 ) ) ;
#12264=CARTESIAN_POINT ( 'NONE',  ( 65.71132485994280614, 155.0000000000000000, -15.00000000000002487 ) ) ;
#12266=CARTESIAN_POINT ( 'NONE',  ( 56.17499999726881299, 164.1591823560292198, 12.60653300113718167 ) ) ;
#12267=EDGE_LOOP ( 'NONE', ( #16031, #10054, #2931, #30752 ) ) ;
#12269=CARTESIAN_POINT ( 'NONE',  ( 125.5000000000000000, 78.52640161467553526, 73.43303922622362734 ) ) ;
#12271=CARTESIAN_POINT ( 'NONE',  ( 56.71132485994280614, 155.0000000000000000, 15.00000000000001243 ) ) ;
#12273=CARTESIAN_POINT ( 'NONE',  ( 63.57499999726881867, 164.1591823560292198, -12.60653300113719766 ) ) ;
#12275=DIRECTION ( 'NONE',  ( 0.000000000000000000, 0.000000000000000000, -1.000000000000000000 ) ) ;
#12280=CARTESIAN_POINT ( 'NONE',  ( 77.20000000000001705, 167.3344367211045096, 8.961492836873468093 ) ) ;
#12281=CARTESIAN_POINT ( 'NONE',  ( 32.50000000000000000, 155.0000000000000000, 15.00000000000001243 ) ) ;
#12284=CARTESIAN_POINT ( 'NONE',  ( 48.68867513459482410, 150.1262045565065364, -15.00000000000012434 ) ) ;
#12285=CARTESIAN_POINT ( 'NONE',  ( 51.47499999726881725, 160.0630714827496206, -15.58253175000000823 ) ) ;
#12288=CARTESIAN_POINT ( 'NONE',  ( 81.12499999726881583, 155.0000000000000000, -15.58253175000000823 ) ) ;
#12289=CARTESIAN_POINT ( 'NONE',  ( 52.61132485994279762, 159.8737954434937478, 14.99999999999991651 ) ) ;
#12291=CARTESIAN_POINT ( 'NONE',  ( 52.49999999453762456, 170.2462022514548323, -7.872454543227099337E-15 ) ) ;
#12292=VERTEX_POINT ( 'NONE', #24219 ) ;
#12294=EDGE_CURVE ( 'NONE', #27576, #12292, #20456, .T. ) ;
#12298=ORIENTED_EDGE ( 'NONE', *, *, #3497, .F. ) ;
#12306=DIRECTION ( 'NONE',  ( 1.000000000000000000, 0.000000000000000000, 0.000000000000000000 ) ) ;
#12309=CARTESIAN_POINT ( 'NONE',  ( 38.77499999726881441, 140.1801316387863778, 4.815267126137185549 ) ) ;
#12310=VERTEX_POINT ( 'NONE', #32057 ) ;
#12311=CARTESIAN_POINT ( 'NONE',  ( 47.32499999726881867, 164.1591823560292198, -12.60653300113719766 ) ) ;
#12312=CARTESIAN_POINT ( 'NONE',  ( 39.78867513459481842, 155.0000000000000000, 15.00000000000001243 ) ) ;
#12316=CARTESIAN_POINT ( 'NONE',  ( 46.97499999726881015, 140.1801316387863778, -4.815267126137194431 ) ) ;
#12319=CARTESIAN_POINT ( 'NONE',  ( 58.41132485994281609, 167.7597621252805880, 9.270509831248428867 ) ) ;
#12320=EDGE_CURVE ( 'NONE', #4513, #7333, #3917, .T. ) ;
#12322=CARTESIAN_POINT ( 'NONE',  ( 59.30000000000000426, 163.5228861582408797, 11.73074641843673049 ) ) ;
#12324=DIRECTION ( 'NONE',  ( 0.000000000000000000, 0.000000000000000000, -1.000000000000000000 ) ) ;
#12327=CARTESIAN_POINT ( 'NONE',  ( 34.37499999726881583, 155.0000000000000000, 15.58253174999999402 ) ) ;
#12329=CARTESIAN_POINT ( 'NONE',  ( 62.52499999726882152, 140.1801316387863778, 4.815267126137185549 ) ) ;
#12333=CARTESIAN_POINT ( 'NONE',  ( 79.87499999726880162, 171.3844434931184253, -7.942151717890132712E-15 ) ) ;
#12337=ORIENTED_EDGE ( 'NONE', *, *, #29099, .T. ) ;
#12339=VECTOR ( 'NONE', #21938, 1000.000000000000000 ) ;
#12352=CARTESIAN_POINT ( 'NONE',  ( 33.71132485994280614, 155.0000000000000000, -15.00000000000002487 ) ) ;
#12356=CARTESIAN_POINT ( 'NONE',  ( 73.17499999726881299, 145.8408176439707802, -12.60653300113719588 ) ) ;
#12357=CARTESIAN_POINT ( 'NONE',  ( 81.42499999726882720, 168.2552932293087906, -9.630534252274385310 ) ) ;
#12362=CARTESIAN_POINT ( 'NONE',  ( 43.50000000000000711, 155.0000000000000000, 14.49999999999999467 ) ) ;
#12368=CARTESIAN_POINT ( 'NONE',  ( 59.82499999726880446, 168.2552932293087906, 9.630534252274372875 ) ) ;
#12369=CARTESIAN_POINT ( 'NONE',  ( 64.87499999726881583, 138.6155565068815463, -3.929120461958505118E-15 ) ) ;
#12378=CARTESIAN_POINT ( 'NONE',  ( 68.01132485994283172, 167.7597621252805880, -9.270509831248443078 ) ) ;
#12382=AXIS2_PLACEMENT_3D ( 'NONE', #28230, #25667, #30271 ) ;
#12386=VERTEX_POINT ( 'NONE', #16213 ) ;
#12387=CARTESIAN_POINT ( 'NONE',  ( 77.97499999726881015, 169.8198683612136222, 4.815267126137181997 ) ) ;
#12393=CARTESIAN_POINT ( 'NONE',  ( 71.12499999726881583, 155.0000000000000000, -15.58253175000000823 ) ) ;
#12396=CARTESIAN_POINT ( 'NONE',  ( 61.42499999726882010, 168.2552932293087906, -9.630534252274385310 ) ) ;
#12398=ORIENTED_EDGE ( 'NONE', *, *, #20830, .T. ) ;
#12401=CARTESIAN_POINT ( 'NONE',  ( 127.5000000000000000, 48.99999999999998579, -1.387778780781445676E-14 ) ) ;
#12405=CYLINDRICAL_SURFACE ( 'NONE', #21817, 15.00000000000001776 ) ;
#12419=CARTESIAN_POINT ( 'NONE',  ( 35.08867513459482979, 167.7597621252805880, -9.270509831248443078 ) ) ;
#12422=CARTESIAN_POINT ( 'NONE',  ( 76.39999999453762314, 168.7903194862797420, -4.480746418436745593 ) ) ;
#12429=EDGE_LOOP ( 'NONE', ( #8362, #24236 ) ) ;
#12430=EDGE_CURVE ( 'NONE', #4983, #5638, #32180, .T. ) ;
#12432=AXIS2_PLACEMENT_3D ( 'NONE', #23312, #7983, #30991 ) ;
#12435=CARTESIAN_POINT ( 'NONE',  ( 50.98867513459482126, 163.8167787843871110, -12.13525491562423397 ) ) ;
#12439=CARTESIAN_POINT ( 'NONE',  ( 84.81132485994280046, 150.1262045565062806, 14.99999999999992006 ) ) ;
#12441=CARTESIAN_POINT ( 'NONE',  ( 57.07499999726880446, 141.7447067706911810, -9.630534252274387086 ) ) ;
#12446=CARTESIAN_POINT ( 'NONE',  ( 57.71132485994280614, 155.0000000000000000, -15.00000000000002487 ) ) ;
#12449=CARTESIAN_POINT ( 'NONE',  ( 64.87499999726881583, 138.6155565068815463, -3.929120461958505118E-15 ) ) ;
#12453=CARTESIAN_POINT ( 'NONE',  ( 87.29999999999999716, 163.5228861582408797, 11.73074641843673049 ) ) ;
#12458=CARTESIAN_POINT ( 'NONE',  ( 53.17499999726881299, 145.8408176439707802, -12.60653300113719588 ) ) ;
#12461=CARTESIAN_POINT ( 'NONE',  ( 83.12499999726881583, 155.0000000000000000, -15.58253175000000823 ) ) ;
#12462=CARTESIAN_POINT ( 'NONE',  ( 41.81132485994281467, 159.8737954434936057, -15.00000000000002665 ) ) ;
#12464=CARTESIAN_POINT ( 'NONE',  ( 54.99999999453762456, 155.0000000000000000, 14.49999999999999467 ) ) ;
#12465=ORIENTED_EDGE ( 'NONE', *, *, #10184, .F. ) ;
#12467=DIRECTION ( 'NONE',  ( 0.000000000000000000, 0.000000000000000000, -1.000000000000000000 ) ) ;
#12469=AXIS2_PLACEMENT_3D ( 'NONE', #4793, #17570, #14503 ) ;
#12476=EDGE_CURVE ( 'NONE', #3282, #30277, #4623, .T. ) ;
#12478=DIRECTION ( 'NONE',  ( -1.000000000000000000, 0.000000000000000000, 0.000000000000000000 ) ) ;
#12483=FACE_OUTER_BOUND ( 'NONE', #21176, .T. ) ;
#12485=CARTESIAN_POINT ( 'NONE',  ( 35.57499999726881157, 164.1591823560292198, -12.60653300113719766 ) ) ;
#12486=ORIENTED_EDGE ( 'NONE', *, *, #12087, .T. ) ;
#12487=CARTESIAN_POINT ( 'NONE',  ( 45.12499999726880873, 155.0000000000000000, -15.58253175000000823 ) ) ;
#12491=CARTESIAN_POINT ( 'NONE',  ( 44.97499999726881015, 140.1801316387863778, -4.815267126137194431 ) ) ;
#12495=CARTESIAN_POINT ( 'NONE',  ( 64.90000000000000568, 168.7903194862797420, -4.480746418436745593 ) ) ;
#12497=CARTESIAN_POINT ( 'NONE',  ( 64.21132485994282035, 170.7719333635740497, -7.904646289410545231E-15 ) ) ;
#12499=CARTESIAN_POINT ( 'NONE',  ( 32.50000000000000000, 155.0000000000000000, 15.00000000000001243 ) ) ;
#12500=CARTESIAN_POINT ( 'NONE',  ( 34.17499999726881299, 164.1591823560292198, 12.60653300113718167 ) ) ;
#12502=CARTESIAN_POINT ( 'NONE',  ( 63.32499999726881867, 164.1591823560292198, -12.60653300113719766 ) ) ;
#12504=ORIENTED_EDGE ( 'NONE', *, *, #21426, .F. ) ;
#12507=CARTESIAN_POINT ( 'NONE',  ( 35.59999999453762598, 141.2096805137202580, -4.480746418436742040 ) ) ;
#12509=VECTOR ( 'NONE', #32518, 1000.000000000000000 ) ;
#12516=CARTESIAN_POINT ( 'NONE',  ( 66.18867513459481700, 140.7341522555726669, 4.635254915624211769 ) ) ;
#12522=CARTESIAN_POINT ( 'NONE',  ( 70.41132485994282320, 167.7597621252805880, 9.270509831248428867 ) ) ;
#12527=ORIENTED_EDGE ( 'NONE', *, *, #8965, .F. ) ;
#12528=CARTESIAN_POINT ( 'NONE',  ( 80.81132485994281467, 150.1262045565062806, 14.99999999999992006 ) ) ;
#12529=CARTESIAN_POINT ( 'NONE',  ( 80.32499999726880446, 145.8408176439707802, 12.60653300113718345 ) ) ;
#12532=DIRECTION ( 'NONE',  ( 0.000000000000000000, 0.000000000000000000, -1.000000000000000000 ) ) ;
#12533=CARTESIAN_POINT ( 'NONE',  ( 42.19999999999999574, 142.6655632788954620, -8.961492836873480528 ) ) ;
#12538=CARTESIAN_POINT ( 'NONE',  ( 55.12499999726881583, 155.0000000000000000, -15.58253175000000823 ) ) ;
#12539=CARTESIAN_POINT ( 'NONE',  ( 69.47499999726881015, 160.0630714827496206, -15.58253175000000823 ) ) ;
#12541=CARTESIAN_POINT ( 'NONE',  ( 41.71132485994280614, 155.0000000000000000, -15.00000000000002487 ) ) ;
#12548=CARTESIAN_POINT ( 'NONE',  ( 74.08867513459483689, 142.2402378747194405, 9.270509831248432420 ) ) ;
#12557=CARTESIAN_POINT ( 'NONE',  ( 80.07499999726879025, 168.2552932293087906, 9.630534252274372875 ) ) ;
#12559=ORIENTED_EDGE ( 'NONE', *, *, #20142, .T. ) ;
#12560=CARTESIAN_POINT ( 'NONE',  ( 71.32499999726881867, 164.1591823560292198, -12.60653300113719766 ) ) ;
#12564=CARTESIAN_POINT ( 'NONE',  ( 60.92499999726882010, 145.8408176439707802, -12.60653300113719588 ) ) ;
#12569=DIRECTION ( 'NONE',  ( 0.000000000000000000, 0.7071067811865506814, 0.7071067811865442421 ) ) ;
#12578=CARTESIAN_POINT ( 'NONE',  ( 39.02499999726880731, 149.9369285172503510, -15.58253175000000823 ) ) ;
#12586=CARTESIAN_POINT ( 'NONE',  ( 75.49999999453763166, 139.7537977485451393, -4.138211985947621020E-15 ) ) ;
#12591=CARTESIAN_POINT ( 'NONE',  ( 74.91132485994280898, 146.1832212156128890, 12.13525491562421976 ) ) ;
#12592=ORIENTED_EDGE ( 'NONE', *, *, #5524, .T. ) ;
#12595=ORIENTED_EDGE ( 'NONE', *, *, #27207, .F. ) ;
#12597=CARTESIAN_POINT ( 'NONE',  ( 51.58867513459482268, 163.8167787843871110, 12.13525491562421621 ) ) ;
#12599=ORIENTED_EDGE ( 'NONE', *, *, #17904, .F. ) ;
#12601=CARTESIAN_POINT ( 'NONE',  ( 81.91132485994279477, 163.8167787843871110, -12.13525491562423397 ) ) ;
#12604=CARTESIAN_POINT ( 'NONE',  ( 56.57499999726881157, 145.8408176439707802, 12.60653300113718345 ) ) ;
#12610=CARTESIAN_POINT ( 'NONE',  ( 66.87499999726880162, 138.6155565068815463, -3.929120461958505118E-15 ) ) ;
#12617=CARTESIAN_POINT ( 'NONE',  ( 34.42499999726880588, 141.7447067706911810, 9.630534252274376428 ) ) ;
#12622=CARTESIAN_POINT ( 'NONE',  ( 51.87499999726880162, 171.3844434931184253, -7.942151717890132712E-15 ) ) ;
#12625=CARTESIAN_POINT ( 'NONE',  ( 52.01132485994281041, 167.7597621252805880, -9.270509831248443078 ) ) ;
#12627=CARTESIAN_POINT ( 'NONE',  ( 51.59999999453762598, 141.2096805137202580, -4.480746418436742040 ) ) ;
#12631=CARTESIAN_POINT ( 'NONE',  ( 60.31132485994280756, 169.2658477444273331, 4.635254915624208216 ) ) ;
#12632=VERTEX_POINT ( 'NONE', #31521 ) ;
#12636=ORIENTED_EDGE ( 'NONE', *, *, #16565, .T. ) ;
#12638=CARTESIAN_POINT ( 'NONE',  ( 49.78867513459482552, 155.0000000000000000, 15.00000000000001243 ) ) ;
#12639=ORIENTED_EDGE ( 'NONE', *, *, #1465, .F. ) ;
#12640=AXIS2_PLACEMENT_3D ( 'NONE', #13645, #26431, #5976 ) ;
#12645=CARTESIAN_POINT ( 'NONE',  ( 39.57499999726881157, 164.1591823560292198, -12.60653300113719766 ) ) ;
#12647=CARTESIAN_POINT ( 'NONE',  ( 42.52499999726880731, 140.1801316387863778, 4.815267126137185549 ) ) ;
#12651=CARTESIAN_POINT ( 'NONE',  ( 47.57499999726881867, 164.1591823560292198, -12.60653300113719766 ) ) ;
#12652=CARTESIAN_POINT ( 'NONE',  ( 78.71132485994280614, 155.0000000000000000, 15.00000000000001243 ) ) ;
#12657=CARTESIAN_POINT ( 'NONE',  ( 64.40000000000001990, 150.2886644046228639, -14.50000000000000888 ) ) ;
#12664=CARTESIAN_POINT ( 'NONE',  ( 72.62499999726880162, 138.6155565068815463, -3.929120461958505118E-15 ) ) ;
#12669=CARTESIAN_POINT ( 'NONE',  ( 34.09999999453762598, 159.7113355953771077, -14.50000000000000888 ) ) ;
#12673=CARTESIAN_POINT ( 'NONE',  ( 41.78867513459481842, 155.0000000000000000, 15.00000000000001243 ) ) ;
#12685=CARTESIAN_POINT ( 'NONE',  ( 70.61132485994282604, 159.8737954434936057, 15.00000000000001421 ) ) ;
#12689=ORIENTED_EDGE ( 'NONE', *, *, #21809, .F. ) ;
#12694=CARTESIAN_POINT ( 'NONE',  ( 84.12499999726881583, 155.0000000000000000, 15.58253174999999402 ) ) ;
#12698=AXIS2_PLACEMENT_3D ( 'NONE', #14439, #19884, #30458 ) ;
#12699=CARTESIAN_POINT ( 'NONE',  ( 45.20000000000000995, 167.3344367211045096, 8.961492836873468093 ) ) ;
#12701=CARTESIAN_POINT ( 'NONE',  ( 88.27499999726880731, 160.0630714827496206, 15.58253174999999402 ) ) ;
#12703=EDGE_CURVE ( 'NONE', #13382, #5796, #5227, .T. ) ;
#12704=CIRCLE ( 'NONE', #15429, 13.00000000000001776 ) ;
#12707=CARTESIAN_POINT ( 'NONE',  ( 58.62499999726880873, 138.6155565068815747, -3.929120461958505118E-15 ) ) ;
#12708=CARTESIAN_POINT ( 'NONE',  ( 70.17499999726881299, 164.1591823560292198, 12.60653300113718167 ) ) ;
#12710=FACE_BOUND ( 'NONE', #7555, .T. ) ;
#12713=EDGE_CURVE ( 'NONE', #14808, #20912, #772, .T. ) ;
#12727=ORIENTED_EDGE ( 'NONE', *, *, #22368, .T. ) ;
#12731=EDGE_LOOP ( 'NONE', ( #13426, #6545, #18129, #2043 ) ) ;
#12732=CARTESIAN_POINT ( 'NONE',  ( 77.77499999726880731, 169.8198683612136222, -4.815267126137197984 ) ) ;
#12735=CARTESIAN_POINT ( 'NONE',  ( 72.72499999726881015, 140.1801316387863778, -4.815267126137194431 ) ) ;
#12738=CARTESIAN_POINT ( 'NONE',  ( 62.72499999726881015, 140.1801316387863778, -4.815267126137194431 ) ) ;
#12753=CARTESIAN_POINT ( 'NONE',  ( 46.38867513459482694, 140.7341522555726669, -4.635254915624220651 ) ) ;
#12755=CARTESIAN_POINT ( 'NONE',  ( 36.92499999726880588, 145.8408176439707802, -12.60653300113719588 ) ) ;
#12764=CARTESIAN_POINT ( 'NONE',  ( 75.19999999453763451, 146.4771138417591203, 11.73074641843673227 ) ) ;
#12765=VERTEX_POINT ( 'NONE', #29293 ) ;
#12770=VERTEX_POINT ( 'NONE', #675 ) ;
#12772=VECTOR ( 'NONE', #28426, 1000.000000000000000 ) ;
#12775=DIRECTION ( 'NONE',  ( 0.000000000000000000, 0.000000000000000000, -1.000000000000000000 ) ) ;
#12776=DIRECTION ( 'NONE',  ( 0.000000000000000000, 1.000000000000000000, -6.454785026890489601E-15 ) ) ;
#12781=CARTESIAN_POINT ( 'NONE',  ( 61.57499999726881157, 164.1591823560292198, -12.60653300113719766 ) ) ;
#12784=( LENGTH_UNIT ( ) NAMED_UNIT ( * ) SI_UNIT ( .MILLI., .METRE. ) );
#12785=LINE ( 'NONE', #10574, #16905 ) ;
#12792=CARTESIAN_POINT ( 'NONE',  ( 34.12499999726881583, 155.0000000000000000, 15.58253174999999402 ) ) ;
#12796=CARTESIAN_POINT ( 'NONE',  ( 50.77499999726880731, 140.1801316387863778, 4.815267126137185549 ) ) ;
#12798=CARTESIAN_POINT ( 'NONE',  ( 32.50000000000000000, 155.0000000000000000, -6.938893903907228378E-15 ) ) ;
#12799=CARTESIAN_POINT ( 'NONE',  ( 78.11132485994281183, 169.2658477444273331, -4.635254915624224203 ) ) ;
#12801=CARTESIAN_POINT ( 'NONE',  ( 52.59999999453762598, 168.7903194862797420, 4.480746418436729606 ) ) ;
#12807=DIRECTION ( 'NONE',  ( 1.000000000000000000, 0.000000000000000000, 0.000000000000000000 ) ) ;
#12814=CARTESIAN_POINT ( 'NONE',  ( 74.27499999726880731, 160.0630714827496206, 15.58253174999999224 ) ) ;
#12818=CARTESIAN_POINT ( 'NONE',  ( 36.27499999726881441, 160.0630714827496206, 15.58253174999999224 ) ) ;
#12820=CARTESIAN_POINT ( 'NONE',  ( 47.12499999726880873, 155.0000000000000000, -15.58253175000000823 ) ) ;
#12823=EDGE_CURVE ( 'NONE', #22989, #30277, #16954, .T. ) ;
#12825=CARTESIAN_POINT ( 'NONE',  ( 48.37499999726880873, 155.0000000000000000, 15.58253174999999402 ) ) ;
#12829=CARTESIAN_POINT ( 'NONE',  ( 66.20000000000001705, 142.6655632788954620, -8.961492836873480528 ) ) ;
#12834=CARTESIAN_POINT ( 'NONE',  ( 57.18867513459483121, 169.2658477444273331, -4.635254915624224203 ) ) ;
#12837=CARTESIAN_POINT ( 'NONE',  ( 67.82499999726881867, 168.2552932293087906, 9.630534252274372875 ) ) ;
#12840=CARTESIAN_POINT ( 'NONE',  ( 35.09999999453762598, 150.2886644046228639, 14.49999999999999645 ) ) ;
#12855=ORIENTED_EDGE ( 'NONE', *, *, #3735, .T. ) ;
#12860=CARTESIAN_POINT ( 'NONE',  ( 81.51132485994280330, 146.1832212156128890, -12.13525491562423042 ) ) ;
#12862=CARTESIAN_POINT ( 'NONE',  ( 80.12499999726881583, 155.0000000000000000, 15.58253174999999402 ) ) ;
#12867=CARTESIAN_POINT ( 'NONE',  ( 48.30000000000000426, 146.4771138417591203, -11.73074641843674470 ) ) ;
#12872=CARTESIAN_POINT ( 'NONE',  ( 52.72499999726881015, 140.1801316387863778, -4.815267126137194431 ) ) ;
#12875=CARTESIAN_POINT ( 'NONE',  ( 59.92499999726881299, 164.1591823560292198, 12.60653300113718167 ) ) ;
#12876=CARTESIAN_POINT ( 'NONE',  ( 70.97499999726881015, 140.1801316387863778, -4.815267126137194431 ) ) ;
#12886=CARTESIAN_POINT ( 'NONE',  ( 34.08867513459483689, 142.2402378747194405, 9.270509831248432420 ) ) ;
#12893=CARTESIAN_POINT ( 'NONE',  ( 74.97499999726881015, 140.1801316387863778, -4.815267126137194431 ) ) ;
#12898=CARTESIAN_POINT ( 'NONE',  ( 68.52499999726880731, 140.1801316387863778, 4.815267126137185549 ) ) ;
#12901=CARTESIAN_POINT ( 'NONE',  ( 61.02499999726880020, 149.9369285172503510, -15.58253175000000823 ) ) ;
#12911=CARTESIAN_POINT ( 'NONE',  ( 45.58867513459481557, 163.8167787843871110, 12.13525491562421621 ) ) ;
#12916=CARTESIAN_POINT ( 'NONE',  ( 87.07499999726880446, 141.7447067706911810, -9.630534252274387086 ) ) ;
#12918=CARTESIAN_POINT ( 'NONE',  ( 39.22499999726881015, 160.0630714827496206, -15.58253175000000823 ) ) ;
#12923=DIRECTION ( 'NONE',  ( 0.4999999999999958367, 0.000000000000000000, -0.8660254037844410391 ) ) ;
#12928=CARTESIAN_POINT ( 'NONE',  ( 73.79999999453762882, 146.4771138417591203, -11.73074641843674470 ) ) ;
#12938=ADVANCED_FACE ( 'NONE', ( #14285 ), #1677, .T. ) ;
#12939=DIRECTION ( 'NONE',  ( 1.000000000000000000, 0.000000000000000000, 0.000000000000000000 ) ) ;
#12942=( BOUNDED_CURVE ( )  B_SPLINE_CURVE ( 2, ( #12352, #7595, #28021, #33307, #15415, #12186, #20363, #2475, #17977, #25638, #4686 ),
 .UNSPECIFIED., .F., .F. ) 
 B_SPLINE_CURVE_WITH_KNOTS ( ( 3, 2, 2, 2, 2, 3 ),
 ( 0.000000000000000000, 0.003571428571428599073, 0.007142857142857198145, 0.01071428571428579765, 0.01428571428571439629, 0.01785714285714299493 ),
 .UNSPECIFIED. ) 
 CURVE ( )  GEOMETRIC_REPRESENTATION_ITEM ( )  RATIONAL_B_SPLINE_CURVE ( ( 1.000000000000000000, 0.9510565162951534202, 1.000000000000000000, 0.9510565162951534202, 1.000000000000000000, 0.9510565162951534202, 1.000000000000000000, 0.9510565162951534202, 1.000000000000000000, 0.9510565162951515328, 1.000000000000001998 ) ) 
 REPRESENTATION_ITEM ( '' )  );
#12947=CARTESIAN_POINT ( 'NONE',  ( 81.81132485994281467, 159.8737954434937478, -14.99999999999993072 ) ) ;
#12950=CARTESIAN_POINT ( 'NONE',  ( 62.47499999726881015, 149.9369285172503510, 15.58253174999999580 ) ) ;
#12960=AXIS2_PLACEMENT_3D ( 'NONE', #9907, #27957, #19619 ) ;
#12963=CARTESIAN_POINT ( 'NONE',  ( 83.50000000000000000, 155.0000000000000000, 14.49999999999999467 ) ) ;
#12966=CARTESIAN_POINT ( 'NONE',  ( 47.88867513459484115, 150.1262045565062806, 14.99999999999992006 ) ) ;
#12967=CARTESIAN_POINT ( 'NONE',  ( 55.87499999726882294, 171.3844434931184253, -7.942151717890132712E-15 ) ) ;
#12970=CARTESIAN_POINT ( 'NONE',  ( 35.71132485994280614, 155.0000000000000000, -15.00000000000002487 ) ) ;
#12974=CARTESIAN_POINT ( 'NONE',  ( 55.79999999453762882, 146.4771138417591203, -11.73074641843674470 ) ) ;
#12989=ORIENTED_EDGE ( 'NONE', *, *, #31007, .T. ) ;
#12992=CARTESIAN_POINT ( 'NONE',  ( 41.77499999726881441, 169.8198683612136222, -4.815267126137197984 ) ) ;
#12994=CARTESIAN_POINT ( 'NONE',  ( 48.12499999726880873, 155.0000000000000000, 15.58253174999999402 ) ) ;
#12995=CARTESIAN_POINT ( 'NONE',  ( 127.5000000000000000, 81.56696077377769427, 76.47359838532574372 ) ) ;
#12998=CARTESIAN_POINT ( 'NONE',  ( 55.87499999726882294, 171.3844434931184253, -7.942151717890132712E-15 ) ) ;
#13002=VECTOR ( 'NONE', #8454, 1000.000000000000114 ) ;
#13004=CARTESIAN_POINT ( 'NONE',  ( 64.50000000000000000, 155.0000000000000000, -14.50000000000000711 ) ) ;
#13006=CARTESIAN_POINT ( 'NONE',  ( 38.68867513459483121, 150.1262045565064227, -15.00000000000002665 ) ) ;
#13012=CARTESIAN_POINT ( 'NONE',  ( 70.02499999726879309, 160.0630714827496206, 15.58253174999999402 ) ) ;
#13015=CARTESIAN_POINT ( 'NONE',  ( 35.49999999453762456, 139.7537977485451393, -4.138211985947621020E-15 ) ) ;
#13024=EDGE_LOOP ( 'NONE', ( #9532, #23621, #28052, #19248 ) ) ;
#13031=CARTESIAN_POINT ( 'NONE',  ( 56.71132485994280614, 155.0000000000000000, 15.00000000000001243 ) ) ;
#13034=CARTESIAN_POINT ( 'NONE',  ( 81.72499999726881015, 169.8198683612136222, 4.815267126137181997 ) ) ;
#13040=CARTESIAN_POINT ( 'NONE',  ( 49.70000000000000284, 146.4771138417591203, 11.73074641843673227 ) ) ;
#13044=CARTESIAN_POINT ( 'NONE',  ( 54.42499999726881299, 141.7447067706911810, 9.630534252274376428 ) ) ;
#13047=CARTESIAN_POINT ( 'NONE',  ( 55.72499999726881015, 169.8198683612136222, 4.815267126137181997 ) ) ;
#13048=CARTESIAN_POINT ( 'NONE',  ( 71.87499999726881583, 171.3844434931184253, -7.942151717890132712E-15 ) ) ;
#13053=CARTESIAN_POINT ( 'NONE',  ( 54.78867513459483263, 155.0000000000000000, -15.00000000000002487 ) ) ;
#13068=CARTESIAN_POINT ( 'NONE',  ( 68.42499999726881299, 141.7447067706911810, 9.630534252274376428 ) ) ;
#13071=CARTESIAN_POINT ( 'NONE',  ( 63.32499999726881867, 164.1591823560292198, -12.60653300113719766 ) ) ;
#13075=AXIS2_PLACEMENT_3D ( 'NONE', #14121, #27070, #843 ) ;
#13078=CARTESIAN_POINT ( 'NONE',  ( 89.50000000000001421, 155.0000000000000000, 13.00000000000001066 ) ) ;
#13086=CARTESIAN_POINT ( 'NONE',  ( 87.43602562408077006, 158.0897711082857882, -15.58253175000000468 ) ) ;
#13088=CARTESIAN_POINT ( 'NONE',  ( 38.32499999726881157, 145.8408176439707802, 12.60653300113718345 ) ) ;
#13095=CARTESIAN_POINT ( 'NONE',  ( 80.99999999453763166, 155.0000000000000000, 14.49999999999999467 ) ) ;
#13106=ORIENTED_EDGE ( 'NONE', *, *, #20817, .F. ) ;
#13112=CARTESIAN_POINT ( 'NONE',  ( 62.77499999726882152, 140.1801316387863778, 4.815267126137185549 ) ) ;
#13116=DIRECTION ( 'NONE',  ( 1.000000000000000000, 0.000000000000000000, 0.000000000000000000 ) ) ;
#13124=CARTESIAN_POINT ( 'NONE',  ( 85.59999999999999432, 150.2886644046228639, 14.49999999999999645 ) ) ;
#13125=CARTESIAN_POINT ( 'NONE',  ( 81.78867513459482552, 155.0000000000000000, 15.00000000000001243 ) ) ;
#13129=CARTESIAN_POINT ( 'NONE',  ( 55.17499999726881299, 145.8408176439707802, -12.60653300113719588 ) ) ;
#13136=CARTESIAN_POINT ( 'NONE',  ( 57.89999999453762314, 150.2886644046228639, -14.50000000000000888 ) ) ;
#13140=CARTESIAN_POINT ( 'NONE',  ( 37.68867513459483121, 159.8737954434936057, 15.00000000000001421 ) ) ;
#13144=( BOUNDED_CURVE ( )  B_SPLINE_CURVE ( 2, ( #14704, #11984, #33278, #25096, #30218, #12497, #4319, #25270, #1935, #9774, #27817 ),
 .UNSPECIFIED., .F., .T. ) 
 B_SPLINE_CURVE_WITH_KNOTS ( ( 3, 2, 2, 2, 2, 3 ),
 ( 0.5357142857142855874, 0.5392857142857141461, 0.5428571428571427049, 0.5464285714285711526, 0.5499999999999998224, 0.5535714285714283811 ),
 .UNSPECIFIED. ) 
 CURVE ( )  GEOMETRIC_REPRESENTATION_ITEM ( )  RATIONAL_B_SPLINE_CURVE ( ( 1.000000000000001554, 0.9510565162951518658, 1.000000000000000000, 0.9510565162951534202, 1.000000000000000000, 0.9510565162951534202, 1.000000000000000000, 0.9510565162951534202, 1.000000000000000000, 0.9510565162951564178, 0.9999999999999970024 ) ) 
 REPRESENTATION_ITEM ( '' )  );
#13149=CARTESIAN_POINT ( 'NONE',  ( 80.18867513459481700, 140.7341522555726669, 4.635254915624211769 ) ) ;
#13154=CARTESIAN_POINT ( 'NONE',  ( 40.87499999726880873, 138.6155565068815747, -3.929120461958505118E-15 ) ) ;
#13156=CARTESIAN_POINT ( 'NONE',  ( 53.02499999726881441, 149.9369285172503510, -15.58253175000000823 ) ) ;
#13161=CARTESIAN_POINT ( 'NONE',  ( 52.17499999726880588, 164.1591823560292198, 12.60653300113718167 ) ) ;
#13165=CARTESIAN_POINT ( 'NONE',  ( 65.50000000000000000, 155.0000000000000000, 14.49999999999999467 ) ) ;
#13170=CARTESIAN_POINT ( 'NONE',  ( 35.07499999726881157, 141.7447067706911810, -9.630534252274385310 ) ) ;
#13172=CARTESIAN_POINT ( 'NONE',  ( 68.82499999726880446, 141.7447067706911810, -9.630534252274385310 ) ) ;
#13176=CARTESIAN_POINT ( 'NONE',  ( 87.87499999726877320, 171.3844434931184253, -7.942151717890132712E-15 ) ) ;
#13187=CARTESIAN_POINT ( 'NONE',  ( 74.61132485994281183, 159.8737954434936057, 15.00000000000001421 ) ) ;
#13195=CARTESIAN_POINT ( 'NONE',  ( 34.47499999726881015, 149.9369285172503510, 15.58253174999999580 ) ) ;
#13200=CARTESIAN_POINT ( 'NONE',  ( 46.59999999999999432, 159.7113355953771077, -14.50000000000000888 ) ) ;
#13204=CARTESIAN_POINT ( 'NONE',  ( 52.22499999726881725, 149.9369285172503510, 15.58253174999999580 ) ) ;
#13207=CARTESIAN_POINT ( 'NONE',  ( 65.72499999726881015, 169.8198683612136222, 4.815267126137181997 ) ) ;
#13208=CARTESIAN_POINT ( 'NONE',  ( 71.57499999726881867, 164.1591823560292198, -12.60653300113719766 ) ) ;
#13212=CARTESIAN_POINT ( 'NONE',  ( 85.08867513459482268, 167.7597621252805880, -9.270509831248443078 ) ) ;
#13214=CIRCLE ( 'NONE', #9968, 2.149999999999984812 ) ;
#13217=CARTESIAN_POINT ( 'NONE',  ( 33.98867513459481415, 146.1832212156128890, 12.13525491562421976 ) ) ;
#13220=EDGE_CURVE ( 'NONE', #7971, #5638, #9860, .T. ) ;
#13225=DIRECTION ( 'NONE',  ( 0.000000000000000000, 0.000000000000000000, -1.000000000000000000 ) ) ;
#13229=VECTOR ( 'NONE', #14772, 1000.000000000000000 ) ;
#13230=CARTESIAN_POINT ( 'NONE',  ( 78.62499999726881583, 138.6155565068815747, -3.929120461958505118E-15 ) ) ;
#13232=CARTESIAN_POINT ( 'NONE',  ( 125.5000000000000000, 231.4735983853260279, 73.43303922622204993 ) ) ;
#13233=CARTESIAN_POINT ( 'NONE',  ( 71.22499999726879594, 160.0630714827496206, -15.58253175000000823 ) ) ;
#13239=DIRECTION ( 'NONE',  ( 0.000000000000000000, 0.7071067811865411334, -0.7071067811865540120 ) ) ;
#13242=CARTESIAN_POINT ( 'NONE',  ( 62.78867513459482552, 155.0000000000000000, -15.00000000000002487 ) ) ;
#13248=CARTESIAN_POINT ( 'NONE',  ( 59.78867513459481842, 155.0000000000000000, 15.00000000000001243 ) ) ;
#13249=CARTESIAN_POINT ( 'NONE',  ( 42.32499999726881157, 145.8408176439707802, 12.60653300113718345 ) ) ;
#13251=CARTESIAN_POINT ( 'NONE',  ( 32.50000000000000000, 155.0000000000000000, -15.00000000000002487 ) ) ;
#13257=CARTESIAN_POINT ( 'NONE',  ( 80.59999999453762598, 168.7903194862797420, 4.480746418436729606 ) ) ;
#13268=CARTESIAN_POINT ( 'NONE',  ( 87.28867513459482552, 170.7719333635740497, -7.904646289410545231E-15 ) ) ;
#13270=DIRECTION ( 'NONE',  ( -1.000000000000000000, 0.000000000000000000, 0.000000000000000000 ) ) ;
#13275=CARTESIAN_POINT ( 'NONE',  ( 65.37499999726881583, 155.0000000000000000, -15.58253175000000823 ) ) ;
#13282=CARTESIAN_POINT ( 'NONE',  ( 86.81132485994281467, 150.1262045565061385, 14.99999999999982947 ) ) ;
#13284=( BOUNDED_CURVE ( )  B_SPLINE_CURVE ( 2, ( #25920, #2592, #2765, #20652, #39, #18088, #12631, #20302, #23198, #20475, #31047 ),
 .UNSPECIFIED., .F., .T. ) 
 B_SPLINE_CURVE_WITH_KNOTS ( ( 3, 2, 2, 2, 2, 3 ),
 ( 0.4642857142857142461, 0.4678571428571428048, 0.4714285714285714191, 0.4749999999999999778, 0.4785714285714286476, 0.4821428571428572063 ),
 .UNSPECIFIED. ) 
 CURVE ( )  GEOMETRIC_REPRESENTATION_ITEM ( )  RATIONAL_B_SPLINE_CURVE ( ( 1.000000000000000666, 0.9510565162951526430, 1.000000000000000000, 0.9510565162951534202, 1.000000000000000000, 0.9510565162951534202, 1.000000000000000000, 0.9510565162951534202, 1.000000000000000000, 0.9510565162951526430, 1.000000000000000666 ) ) 
 REPRESENTATION_ITEM ( '' )  );
#13286=CYLINDRICAL_SURFACE ( 'NONE', #33141, 15.00000000000001776 ) ;
#13289=CARTESIAN_POINT ( 'NONE',  ( 41.52499999726881441, 169.8198683612136222, -4.815267126137197984 ) ) ;
#13292=CARTESIAN_POINT ( 'NONE',  ( 48.18867513459482410, 140.7341522555726669, 4.635254915624211769 ) ) ;
#13293=CARTESIAN_POINT ( 'NONE',  ( 55.37499999726881583, 155.0000000000000000, -15.58253175000000823 ) ) ;
#13297=CARTESIAN_POINT ( 'NONE',  ( 86.92499999726881299, 145.8408176439707802, -12.60653300113719588 ) ) ;
#13300=CARTESIAN_POINT ( 'NONE',  ( 58.59999999453763309, 168.7903194862797420, 4.480746418436729606 ) ) ;
#13303=DIRECTION ( 'NONE',  ( -1.000000000000000000, -0.000000000000000000, 0.000000000000000000 ) ) ;
#13305=CARTESIAN_POINT ( 'NONE',  ( 44.81132485994280756, 150.1262045565063943, 14.99999999999999289 ) ) ;
#13312=ORIENTED_EDGE ( 'NONE', *, *, #12823, .F. ) ;
#13317=CARTESIAN_POINT ( 'NONE',  ( 41.47499999726881015, 160.0630714827496206, -15.58253175000000823 ) ) ;
#13318=ORIENTED_EDGE ( 'NONE', *, *, #5380, .T. ) ;
#13319=CARTESIAN_POINT ( 'NONE',  ( 50.62499999726880162, 138.6155565068815463, -3.929120461958505118E-15 ) ) ;
#13324=CARTESIAN_POINT ( 'NONE',  ( 54.37499999726881583, 155.0000000000000000, 15.58253174999999402 ) ) ;
#13327=CARTESIAN_POINT ( 'NONE',  ( 44.18867513459481700, 140.7341522555726669, 4.635254915624211769 ) ) ;
#13329=CARTESIAN_POINT ( 'NONE',  ( 74.70000000000000284, 163.5228861582408797, -11.73074641843674470 ) ) ;
#13333=CARTESIAN_POINT ( 'NONE',  ( 40.17499999726881299, 164.1591823560292198, 12.60653300113718167 ) ) ;
#13334=EDGE_CURVE ( 'NONE', #9027, #31619, #14767, .T. ) ;
#13336=CARTESIAN_POINT ( 'NONE',  ( 70.12499999726881583, 155.0000000000000000, 15.58253174999999402 ) ) ;
#13339=CARTESIAN_POINT ( 'NONE',  ( 41.89999999453762314, 150.2886644046228639, -14.50000000000000888 ) ) ;
#13345=LINE ( 'NONE', #20853, #177 ) ;
#13347=ORIENTED_EDGE ( 'NONE', *, *, #10960, .T. ) ;
#13349=CARTESIAN_POINT ( 'NONE',  ( 73.91132485994280898, 163.8167787843871110, -12.13525491562423397 ) ) ;
#13357=CARTESIAN_POINT ( 'NONE',  ( 33.92499999726881299, 164.1591823560292198, 12.60653300113718167 ) ) ;
#13358=CARTESIAN_POINT ( 'NONE',  ( 36.57499999726881157, 145.8408176439707802, 12.60653300113718345 ) ) ;
#13362=CARTESIAN_POINT ( 'NONE',  ( 48.70000000000000284, 163.5228861582408797, -11.73074641843674470 ) ) ;
#13364=CYLINDRICAL_SURFACE ( 'NONE', #14523, 2.149999999999994138 ) ;
#13365=CARTESIAN_POINT ( 'NONE',  ( 50.42499999726880588, 141.7447067706911810, 9.630534252274376428 ) ) ;
#13368=CARTESIAN_POINT ( 'NONE',  ( 62.52499999726882152, 140.1801316387863778, 4.815267126137185549 ) ) ;
#13369=CARTESIAN_POINT ( 'NONE',  ( 79.47499999726881015, 160.0630714827496206, -15.58253175000000823 ) ) ;
#13373=CARTESIAN_POINT ( 'NONE',  ( 53.98867513459482126, 146.1832212156128890, 12.13525491562421976 ) ) ;
#13378=CARTESIAN_POINT ( 'NONE',  ( 34.28867513459483263, 139.2280666364260071, -4.041636747397287284E-15 ) ) ;
#13382=VERTEX_POINT ( 'NONE', #21744 ) ;
#13387=EDGE_LOOP ( 'NONE', ( #22557, #32290 ) ) ;
#13388=CARTESIAN_POINT ( 'NONE',  ( 80.22499999726881015, 149.9369285172503510, 15.58253174999999580 ) ) ;
#13392=CARTESIAN_POINT ( 'NONE',  ( 67.92499999726881299, 164.1591823560292198, 12.60653300113718167 ) ) ;
#13410=CARTESIAN_POINT ( 'NONE',  ( 47.22499999726881015, 160.0630714827496206, -15.58253175000000823 ) ) ;
#13417=CARTESIAN_POINT ( 'NONE',  ( 79.29999999453762882, 142.6655632788954620, 8.961492836873471646 ) ) ;
#13421=CARTESIAN_POINT ( 'NONE',  ( 49.18867513459482410, 169.2658477444273331, -4.635254915624224203 ) ) ;
#13426=ORIENTED_EDGE ( 'NONE', *, *, #1239, .F. ) ;
#13428=CARTESIAN_POINT ( 'NONE',  ( 77.27499999726882152, 149.9369285172503510, -15.58253175000000823 ) ) ;
#13433=CARTESIAN_POINT ( 'NONE',  ( 65.87499999726880162, 171.3844434931184253, -7.942151717890134290E-15 ) ) ;
#13437=( NAMED_UNIT ( * ) SI_UNIT ( $, .STERADIAN. ) SOLID_ANGLE_UNIT ( ) );
#13445=CARTESIAN_POINT ( 'NONE',  ( 86.97499999726882436, 140.1801316387863778, -4.815267126137194431 ) ) ;
#13449=CARTESIAN_POINT ( 'NONE',  ( 38.92499999726881299, 145.8408176439707802, -12.60653300113719588 ) ) ;
#13454=CARTESIAN_POINT ( 'NONE',  ( 54.77499999726881441, 140.1801316387863778, 4.815267126137185549 ) ) ;
#13462=CARTESIAN_POINT ( 'NONE',  ( 59.39999999453763024, 141.2096805137202580, 4.480746418436733158 ) ) ;
#13467=CARTESIAN_POINT ( 'NONE',  ( 72.21132485994282035, 170.7719333635740497, -7.904646289410545231E-15 ) ) ;
#13474=DIRECTION ( 'NONE',  ( 0.000000000000000000, 0.000000000000000000, -1.000000000000000000 ) ) ;
#13475=ORIENTED_EDGE ( 'NONE', *, *, #15983, .T. ) ;
#13480=CARTESIAN_POINT ( 'NONE',  ( 42.27499999726880731, 160.0630714827496206, 15.58253174999999224 ) ) ;
#13483=CARTESIAN_POINT ( 'NONE',  ( 48.32499999726881157, 145.8408176439707802, 12.60653300113718345 ) ) ;
#13485=CARTESIAN_POINT ( 'NONE',  ( 60.98867513459482836, 163.8167787843871110, -12.13525491562423397 ) ) ;
#13487=CARTESIAN_POINT ( 'NONE',  ( 53.87499999726881583, 171.3844434931184253, -7.942151717890132712E-15 ) ) ;
#13489=CARTESIAN_POINT ( 'NONE',  ( 127.5000000000000000, 155.0000000000010800, 106.0000000000000142 ) ) ;
#13490=EDGE_CURVE ( 'NONE', #27429, #15361, #30257, .T. ) ;
#13491=CARTESIAN_POINT ( 'NONE',  ( 76.80000000000001137, 167.3344367211045096, -8.961492836873482304 ) ) ;
#13492=CARTESIAN_POINT ( 'NONE',  ( 40.18867513459483121, 140.7341522555726669, 4.635254915624211769 ) ) ;
#13497=CARTESIAN_POINT ( 'NONE',  ( 39.77499999726881441, 169.8198683612136222, -4.815267126137197984 ) ) ;
#13500=CARTESIAN_POINT ( 'NONE',  ( 80.12499999726881583, 155.0000000000000000, 15.58253174999999402 ) ) ;
#13503=CARTESIAN_POINT ( 'NONE',  ( 48.61132485994281893, 159.8737954434936057, 15.00000000000001421 ) ) ;
#13504=CARTESIAN_POINT ( 'NONE',  ( 40.29999999453762882, 167.3344367211045096, -8.961492836873482304 ) ) ;
#13526=CARTESIAN_POINT ( 'NONE',  ( 35.57499999726881157, 164.1591823560292198, -12.60653300113719766 ) ) ;
#13531=CARTESIAN_POINT ( 'NONE',  ( 53.60000000000000853, 150.2886644046228639, 14.49999999999999645 ) ) ;
#13534=CARTESIAN_POINT ( 'NONE',  ( 59.52499999726881441, 169.8198683612136222, -4.815267126137197984 ) ) ;
#13538=CARTESIAN_POINT ( 'NONE',  ( 62.02499999726880020, 160.0630714827496206, 15.58253174999999224 ) ) ;
#13539=CARTESIAN_POINT ( 'NONE',  ( 78.27499999726880731, 160.0630714827496206, 15.58253174999999402 ) ) ;
#13541=CARTESIAN_POINT ( 'NONE',  ( 49.21132485994281325, 139.2280666364260071, -4.041636747397287284E-15 ) ) ;
#13558=ORIENTED_EDGE ( 'NONE', *, *, #2237, .T. ) ;
#13563=VERTEX_POINT ( 'NONE', #1134 ) ;
#13564=CARTESIAN_POINT ( 'NONE',  ( 75.42499999726879878, 168.2552932293087906, -9.630534252274387086 ) ) ;
#13565=DIRECTION ( 'NONE',  ( 0.000000000000000000, 0.000000000000000000, -1.000000000000000000 ) ) ;
#13568=CARTESIAN_POINT ( 'NONE',  ( 70.42499999726881299, 141.7447067706911810, 9.630534252274376428 ) ) ;
#13572=CARTESIAN_POINT ( 'NONE',  ( 35.29999999999999716, 163.5228861582408797, 11.73074641843673049 ) ) ;
#13575=DIRECTION ( 'NONE',  ( -1.000000000000000000, -0.000000000000000000, 0.000000000000000000 ) ) ;
#13581=CARTESIAN_POINT ( 'NONE',  ( 44.72499999726881015, 140.1801316387863778, -4.815267126137194431 ) ) ;
#13588=CARTESIAN_POINT ( 'NONE',  ( 76.59999999453762598, 168.7903194862797420, 4.480746418436729606 ) ) ;
#13593=EDGE_LOOP ( 'NONE', ( #29234, #29785, #4600, #7743 ) ) ;
#13597=CARTESIAN_POINT ( 'NONE',  ( 79.27499999726880731, 149.9369285172503510, -15.58253175000000823 ) ) ;
#13598=CARTESIAN_POINT ( 'NONE',  ( 52.91132485994280898, 146.1832212156128890, 12.13525491562421976 ) ) ;
#13602=CARTESIAN_POINT ( 'NONE',  ( 69.87499999726880162, 171.3844434931184253, -7.942151717890134290E-15 ) ) ;
#13605=CARTESIAN_POINT ( 'NONE',  ( 43.48867513459482836, 167.7597621252805880, 9.270509831248428867 ) ) ;
#13611=CARTESIAN_POINT ( 'NONE',  ( 83.17499999726882720, 145.8408176439707802, -12.60653300113719588 ) ) ;
#13614=CARTESIAN_POINT ( 'NONE',  ( 40.42499999726881299, 141.7447067706911810, 9.630534252274376428 ) ) ;
#13618=CARTESIAN_POINT ( 'NONE',  ( 55.67499999726879878, 168.2552932293087906, -9.630534252274385310 ) ) ;
#13622=CARTESIAN_POINT ( 'NONE',  ( 78.71132485994280614, 155.0000000000000000, 15.00000000000001243 ) ) ;
#13625=CARTESIAN_POINT ( 'NONE',  ( 60.89999999453761603, 159.7113355953771077, 14.49999999999999289 ) ) ;
#13626=EDGE_LOOP ( 'NONE', ( #10393, #33552, #51, #3448, #33138, #3840 ) ) ;
#13628=CARTESIAN_POINT ( 'NONE',  ( 37.28867513459483263, 170.7719333635740497, -7.904646289410545231E-15 ) ) ;
#13640=CARTESIAN_POINT ( 'NONE',  ( 89.50000000000001421, 155.0000000000000000, -6.938893903907228378E-15 ) ) ;
#13642=CARTESIAN_POINT ( 'NONE',  ( 42.17499999726881299, 164.1591823560292198, 12.60653300113718167 ) ) ;
#13643=ORIENTED_EDGE ( 'NONE', *, *, #2660, .F. ) ;
#13644=CARTESIAN_POINT ( 'NONE',  ( 51.02499999726880731, 149.9369285172503510, -15.58253175000000823 ) ) ;
#13645=CARTESIAN_POINT ( 'NONE',  ( 127.5000000000000000, 154.9999999999996305, -106.0000000000000142 ) ) ;
#13650=CARTESIAN_POINT ( 'NONE',  ( 55.47499999726881015, 160.0630714827496206, -15.58253175000000823 ) ) ;
#13654=CARTESIAN_POINT ( 'NONE',  ( 70.90000000000000568, 168.7903194862797420, -4.480746418436745593 ) ) ;
#13655=CARTESIAN_POINT ( 'NONE',  ( 62.61132485994281893, 159.8737954434936057, 15.00000000000001421 ) ) ;
#13659=CARTESIAN_POINT ( 'NONE',  ( 35.67499999726880588, 168.2552932293087906, -9.630534252274385310 ) ) ;
#13661=CARTESIAN_POINT ( 'NONE',  ( 74.42499999726881299, 141.7447067706911810, 9.630534252274376428 ) ) ;
#13663=CARTESIAN_POINT ( 'NONE',  ( 40.39999999453763024, 168.7903194862797420, -4.480746418436745593 ) ) ;
#13674=ADVANCED_FACE ( 'NONE', ( #14582 ), #8968, .T. ) ;
#13675=CARTESIAN_POINT ( 'NONE',  ( 50.58867513459482268, 146.1832212156128890, -12.13525491562423042 ) ) ;
#13683=CARTESIAN_POINT ( 'NONE',  ( 87.52499999726882152, 169.8198683612136222, -4.815267126137197984 ) ) ;
#13686=CARTESIAN_POINT ( 'NONE',  ( 57.60000000000000142, 150.2886644046228639, 14.49999999999999645 ) ) ;
#13689=EDGE_CURVE ( 'NONE', #24269, #608, #32972, .T. ) ;
#13690=CARTESIAN_POINT ( 'NONE',  ( 57.62499999726880873, 171.3844434931184253, -7.942151717890132712E-15 ) ) ;
#13694=CARTESIAN_POINT ( 'NONE',  ( 62.82499999726881867, 141.7447067706911810, -9.630534252274387086 ) ) ;
#13695=CARTESIAN_POINT ( 'NONE',  ( 76.97499999726881015, 140.1801316387863778, -4.815267126137194431 ) ) ;
#13697=FACE_OUTER_BOUND ( 'NONE', #9022, .T. ) ;
#13710=ORIENTED_EDGE ( 'NONE', *, *, #17229, .F. ) ;
#13713=ORIENTED_EDGE ( 'NONE', *, *, #28526, .F. ) ;
#13717=CARTESIAN_POINT ( 'NONE',  ( 76.72499999726881015, 140.1801316387863778, -4.815267126137194431 ) ) ;
#13722=CARTESIAN_POINT ( 'NONE',  ( 69.82499999726880446, 168.2552932293087906, 9.630534252274372875 ) ) ;
#13724=EDGE_CURVE ( 'NONE', #16104, #13382, #19693, .T. ) ;
#13726=EDGE_CURVE ( 'NONE', #3615, #9027, #1469, .T. ) ;
#13728=CARTESIAN_POINT ( 'NONE',  ( 32.70000000000000284, 163.5228861582408797, -11.73074641843674470 ) ) ;
#13732=PRODUCT_DEFINITION ( 'UNKNOWN', '', #5049, #24414 ) ;
#13733=EDGE_CURVE ( 'NONE', #33037, #12292, #32638, .T. ) ;
#13740=CARTESIAN_POINT ( 'NONE',  ( 43.82499999726881157, 168.2552932293087906, 9.630534252274372875 ) ) ;
#13749=CARTESIAN_POINT ( 'NONE',  ( 81.09999999453764019, 150.2886644046228639, 14.49999999999999645 ) ) ;
#13755=AXIS2_PLACEMENT_3D ( 'NONE', #2514, #20735, #18187 ) ;
#13759=ORIENTED_EDGE ( 'NONE', *, *, #6759, .T. ) ;
#13763=CARTESIAN_POINT ( 'NONE',  ( 76.37499999726881583, 155.0000000000000000, 15.58253174999999402 ) ) ;
#13770=CARTESIAN_POINT ( 'NONE',  ( 67.97499999726881015, 169.8198683612136222, 4.815267126137181997 ) ) ;
#13772=CARTESIAN_POINT ( 'NONE',  ( 68.08867513459483689, 142.2402378747194405, 9.270509831248432420 ) ) ;
#13780=CARTESIAN_POINT ( 'NONE',  ( 87.17499999726881299, 145.8408176439707802, -12.60653300113719588 ) ) ;
#13784=CARTESIAN_POINT ( 'NONE',  ( 36.42499999726879878, 141.7447067706911810, 9.630534252274376428 ) ) ;
#13789=CARTESIAN_POINT ( 'NONE',  ( 63.67499999726880588, 168.2552932293087906, -9.630534252274385310 ) ) ;
#13797=CARTESIAN_POINT ( 'NONE',  ( 61.49999999453762456, 139.7537977485451393, -4.138211985947621020E-15 ) ) ;
#13800=CYLINDRICAL_SURFACE ( 'NONE', #24070, 15.00000000000001776 ) ;
#13808=CARTESIAN_POINT ( 'NONE',  ( 50.31132485994280046, 169.2658477444273331, 4.635254915624208216 ) ) ;
#13814=CARTESIAN_POINT ( 'NONE',  ( 51.37499999726881583, 155.0000000000000000, -15.58253175000000823 ) ) ;
#13816=CARTESIAN_POINT ( 'NONE',  ( 58.12499999726881583, 155.0000000000000000, 15.58253174999999402 ) ) ;
#13822=CARTESIAN_POINT ( 'NONE',  ( 62.17499999726882010, 164.1591823560292198, 12.60653300113718167 ) ) ;
#13824=CARTESIAN_POINT ( 'NONE',  ( 46.78867513459482552, 155.0000000000000000, -15.00000000000002487 ) ) ;
#13828=CARTESIAN_POINT ( 'NONE',  ( 72.00000000000001421, 139.7537977485451393, -4.138211985947621020E-15 ) ) ;
#13830=FACE_OUTER_BOUND ( 'NONE', #8288, .T. ) ;
#13833=CARTESIAN_POINT ( 'NONE',  ( 38.37499999726880873, 155.0000000000000000, 15.58253174999999402 ) ) ;
#13836=CARTESIAN_POINT ( 'NONE',  ( 74.22499999726881015, 149.9369285172503510, 15.58253174999999580 ) ) ;
#13839=CARTESIAN_POINT ( 'NONE',  ( 43.19999999453762740, 146.4771138417591203, 11.73074641843673227 ) ) ;
#13859=CARTESIAN_POINT ( 'NONE',  ( 35.12499999726881583, 155.0000000000000000, -15.58253175000000823 ) ) ;
#13861=CARTESIAN_POINT ( 'NONE',  ( 36.07499999726880446, 168.2552932293087906, 9.630534252274372875 ) ) ;
#13864=CARTESIAN_POINT ( 'NONE',  ( 52.00000000000000000, 139.7537977485451393, -4.138211985947621020E-15 ) ) ;
#13868=CARTESIAN_POINT ( 'NONE',  ( 55.02499999726881441, 149.9369285172503510, -15.58253175000000823 ) ) ;
#13871=CARTESIAN_POINT ( 'NONE',  ( 64.62499999726881583, 138.6155565068815747, -3.929120461958505118E-15 ) ) ;
#13872=CARTESIAN_POINT ( 'NONE',  ( 77.87499999726881583, 171.3844434931184253, -7.942151717890132712E-15 ) ) ;
#13878=ORIENTED_EDGE ( 'NONE', *, *, #4596, .F. ) ;
#13887=CARTESIAN_POINT ( 'NONE',  ( 71.78867513459482552, 155.0000000000000000, 15.00000000000001243 ) ) ;
#13893=EDGE_CURVE ( 'NONE', #5650, #19014, #28212, .T. ) ;
#13894=CARTESIAN_POINT ( 'NONE',  ( 78.42499999726881299, 141.7447067706911810, 9.630534252274376428 ) ) ;
#13899=CARTESIAN_POINT ( 'NONE',  ( 67.72499999726881015, 169.8198683612136222, 4.815267126137181997 ) ) ;
#13903=CARTESIAN_POINT ( 'NONE',  ( 34.00000000000000711, 139.7537977485451393, -4.138211985947621020E-15 ) ) ;
#13907=EDGE_CURVE ( 'NONE', #5638, #5752, #12191, .T. ) ;
#13911=CARTESIAN_POINT ( 'NONE',  ( 60.38867513459481984, 140.7341522555726669, -4.635254915624220651 ) ) ;
#13912=CARTESIAN_POINT ( 'NONE',  ( 43.22499999726881015, 160.0630714827496206, -15.58253175000000823 ) ) ;
#13919=CARTESIAN_POINT ( 'NONE',  ( 86.79999999453762882, 163.5228861582408797, 11.73074641843673049 ) ) ;
#13931=CARTESIAN_POINT ( 'NONE',  ( 80.07499999726880446, 168.2552932293087906, 9.630534252274372875 ) ) ;
#13933=CARTESIAN_POINT ( 'NONE',  ( 59.18867513459482410, 169.2658477444273331, -4.635254915624224203 ) ) ;
#13938=CARTESIAN_POINT ( 'NONE',  ( 69.07499999726881867, 141.7447067706911810, -9.630534252274387086 ) ) ;
#13941=CARTESIAN_POINT ( 'NONE',  ( 36.71132485994280614, 155.0000000000000000, 15.00000000000001243 ) ) ;
#13942=CARTESIAN_POINT ( 'NONE',  ( 51.88867513459483405, 150.1262045565062806, 14.99999999999992006 ) ) ;
#13943=CARTESIAN_POINT ( 'NONE',  ( 125.5000000000000000, 152.8499999999996533, -106.0000000000000000 ) ) ;
#13947=CARTESIAN_POINT ( 'NONE',  ( 83.27499999726880731, 149.9369285172503510, -15.58253175000000823 ) ) ;
#13950=CARTESIAN_POINT ( 'NONE',  ( 39.82499999726880446, 168.2552932293087906, 9.630534252274372875 ) ) ;
#13955=CARTESIAN_POINT ( 'NONE',  ( 63.57499999726881867, 164.1591823560292198, -12.60653300113719766 ) ) ;
#13961=CARTESIAN_POINT ( 'NONE',  ( 65.29999999453762882, 142.6655632788954620, 8.961492836873471646 ) ) ;
#13974=CARTESIAN_POINT ( 'NONE',  ( 49.91132485994280188, 163.8167787843871110, -12.13525491562423397 ) ) ;
#13981=CARTESIAN_POINT ( 'NONE',  ( 47.07499999726881157, 141.7447067706911810, -9.630534252274387086 ) ) ;
#13983=CARTESIAN_POINT ( 'NONE',  ( 56.52499999726881441, 140.1801316387863778, 4.815267126137185549 ) ) ;
#13989=CARTESIAN_POINT ( 'NONE',  ( 58.27499999726880731, 160.0630714827496206, 15.58253174999999402 ) ) ;
#13991=CARTESIAN_POINT ( 'NONE',  ( 47.48867513459482836, 167.7597621252805880, 9.270509831248428867 ) ) ;
#13994=CARTESIAN_POINT ( 'NONE',  ( 73.89999999999999147, 141.2096805137202580, 4.480746418436733158 ) ) ;
#13998=CARTESIAN_POINT ( 'NONE',  ( 32.78867513459481842, 155.0000000000000000, -15.00000000000002487 ) ) ;
#13999=CARTESIAN_POINT ( 'NONE',  ( 46.97499999726881015, 140.1801316387863778, -4.815267126137194431 ) ) ;
#14001=CARTESIAN_POINT ( 'NONE',  ( 76.62499999726880162, 138.6155565068815463, -3.929120461958505118E-15 ) ) ;
#14004=CARTESIAN_POINT ( 'NONE',  ( 45.19999999453762740, 146.4771138417591203, 11.73074641843673227 ) ) ;
#14014=ORIENTED_EDGE ( 'NONE', *, *, #7853, .T. ) ;
#14016=VECTOR ( 'NONE', #18454, 1000.000000000000000 ) ;
#14017=CARTESIAN_POINT ( 'NONE',  ( 51.11132485994281183, 140.7341522555726669, 4.635254915624211769 ) ) ;
#14021=FACE_OUTER_BOUND ( 'NONE', #6396, .T. ) ;
#14023=CARTESIAN_POINT ( 'NONE',  ( 40.42499999726881299, 141.7447067706911810, 9.630534252274376428 ) ) ;
#14026=CARTESIAN_POINT ( 'NONE',  ( 42.07499999726881157, 168.2552932293087906, 9.630534252274372875 ) ) ;
#14031=AXIS2_PLACEMENT_3D ( 'NONE', #15581, #31272, #33483 ) ;
#14032=CARTESIAN_POINT ( 'NONE',  ( 56.90000000000000568, 168.7903194862797420, -4.480746418436745593 ) ) ;
#14037=CARTESIAN_POINT ( 'NONE',  ( 56.52499999726881441, 140.1801316387863778, 4.815267126137185549 ) ) ;
#14040=CYLINDRICAL_SURFACE ( 'NONE', #29868, 15.00000000000001776 ) ;
#14041=CARTESIAN_POINT ( 'NONE',  ( 67.02499999726880731, 149.9369285172503510, -15.58253175000000823 ) ) ;
#14042=CARTESIAN_POINT ( 'NONE',  ( 78.87499999726878741, 138.6155565068815463, -3.929120461958505118E-15 ) ) ;
#14062=CARTESIAN_POINT ( 'NONE',  ( 86.12499999726881583, 155.0000000000000000, 15.58253174999999402 ) ) ;
#14065=CARTESIAN_POINT ( 'NONE',  ( 78.62499999726881583, 138.6155565068815463, -3.929120461958505118E-15 ) ) ;
#14068=CARTESIAN_POINT ( 'NONE',  ( 35.10000000000000142, 168.7903194862797420, 4.480746418436729606 ) ) ;
#14079=CARTESIAN_POINT ( 'NONE',  ( 51.52499999726881441, 169.8198683612136222, -4.815267126137197984 ) ) ;
#14087=CARTESIAN_POINT ( 'NONE',  ( 83.19999999453763451, 146.4771138417591203, 11.73074641843673227 ) ) ;
#14090=EDGE_CURVE ( 'NONE', #13563, #28748, #32188, .T. ) ;
#14092=DIRECTION ( 'NONE',  ( 1.000000000000000000, 0.000000000000000000, 0.000000000000000000 ) ) ;
#14095=VERTEX_POINT ( 'NONE', #24926 ) ;
#14096=CARTESIAN_POINT ( 'NONE',  ( 73.57499999726880446, 164.1591823560292198, -12.60653300113719766 ) ) ;
#14100=CARTESIAN_POINT ( 'NONE',  ( 83.67499999726884141, 168.2552932293087906, -9.630534252274387086 ) ) ;
#14106=CARTESIAN_POINT ( 'NONE',  ( 68.67499999726881299, 141.7447067706911810, 9.630534252274376428 ) ) ;
#14112=( BOUNDED_CURVE ( )  B_SPLINE_CURVE ( 2, ( #2584, #7697, #18249, #7361, #15851, #26242, #18080, #2912, #15519, #25911, #12970 ),
 .UNSPECIFIED., .F., .T. ) 
 B_SPLINE_CURVE_WITH_KNOTS ( ( 3, 2, 2, 2, 2, 3 ),
 ( 0.01785714285714299493, 0.02142857142857154673, 0.02500000000000009853, 0.02857142857142864686, 0.03214285714285719520, 0.03571428571428574700 ),
 .UNSPECIFIED. ) 
 CURVE ( )  GEOMETRIC_REPRESENTATION_ITEM ( )  RATIONAL_B_SPLINE_CURVE ( ( 0.9999999999999981126, 0.9510565162951553075, 1.000000000000000000, 0.9510565162951534202, 1.000000000000000000, 0.9510565162951534202, 1.000000000000000000, 0.9510565162951534202, 1.000000000000000000, 0.9510565162951529761, 1.000000000000000444 ) ) 
 REPRESENTATION_ITEM ( '' )  );
#14119=CARTESIAN_POINT ( 'NONE',  ( 43.02499999726880020, 149.9369285172503510, -15.58253175000000823 ) ) ;
#14120=CARTESIAN_POINT ( 'NONE',  ( 35.88867513459481984, 150.1262045565062806, 14.99999999999992006 ) ) ;
#14121=CARTESIAN_POINT ( 'NONE',  ( 125.5000000000000000, 80.04668119422552763, -74.95331880577366235 ) ) ;
#14124=CARTESIAN_POINT ( 'NONE',  ( 82.78867513459482552, 155.0000000000000000, -15.00000000000002487 ) ) ;
#14128=DIRECTION ( 'NONE',  ( 1.000000000000000000, 0.000000000000000000, 0.000000000000000000 ) ) ;
#14132=CARTESIAN_POINT ( 'NONE',  ( 67.79999999453762882, 146.4771138417591203, -11.73074641843674470 ) ) ;
#14137=CARTESIAN_POINT ( 'NONE',  ( 83.31132485994280046, 140.7341522555726669, -4.635254915624220651 ) ) ;
#14143=DIRECTION ( 'NONE',  ( 0.000000000000000000, -1.000000000000000000, 0.000000000000000000 ) ) ;
#14144=LINE ( 'NONE', #16527, #18726 ) ;
#14149=CARTESIAN_POINT ( 'NONE',  ( 49.47499999726881725, 160.0630714827496206, -15.58253175000000823 ) ) ;
#14151=CARTESIAN_POINT ( 'NONE',  ( 58.72499999726881015, 140.1801316387863778, -4.815267126137194431 ) ) ;
#14157=CARTESIAN_POINT ( 'NONE',  ( 61.77499999726881441, 169.8198683612136222, -4.815267126137197984 ) ) ;
#14163=AXIS2_PLACEMENT_3D ( 'NONE', #4785, #15178, #25571 ) ;
#14164=CARTESIAN_POINT ( 'NONE',  ( 79.40000000000000568, 159.7113355953771077, 14.49999999999999289 ) ) ;
#14165=CARTESIAN_POINT ( 'NONE',  ( 65.28867513459482552, 170.7719333635740497, -7.904646289410545231E-15 ) ) ;
#14166=FACE_OUTER_BOUND ( 'NONE', #11806, .T. ) ;
#14169=CARTESIAN_POINT ( 'NONE',  ( 43.17499999726881299, 145.8408176439707802, -12.60653300113719588 ) ) ;
#14170=EDGE_CURVE ( 'NONE', #2840, #10102, #25600, .T. ) ;
#14172=CARTESIAN_POINT ( 'NONE',  ( 77.92499999726881299, 164.1591823560292198, 12.60653300113718167 ) ) ;
#14176=CARTESIAN_POINT ( 'NONE',  ( 44.49999999453763166, 170.2462022514548323, -7.872454543227099337E-15 ) ) ;
#14187=CARTESIAN_POINT ( 'NONE',  ( 50.71132485994280614, 155.0000000000000000, 15.00000000000001243 ) ) ;
#14195=CARTESIAN_POINT ( 'NONE',  ( 41.02499999726880731, 149.9369285172503510, -15.58253175000000823 ) ) ;
#14197=CARTESIAN_POINT ( 'NONE',  ( 43.67499999726881299, 168.2552932293087906, -9.630534252274385310 ) ) ;
#14201=CARTESIAN_POINT ( 'NONE',  ( 56.20000000000000284, 142.6655632788954620, -8.961492836873480528 ) ) ;
#14202=CARTESIAN_POINT ( 'NONE',  ( 63.68867513459485252, 159.8737954434935489, 15.00000000000006040 ) ) ;
#14206=CARTESIAN_POINT ( 'NONE',  ( 57.92499999726881299, 164.1591823560292198, 12.60653300113718167 ) ) ;
#14208=VERTEX_POINT ( 'NONE', #18271 ) ;
#14211=CARTESIAN_POINT ( 'NONE',  ( 82.97499999726881015, 140.1801316387863778, -4.815267126137194431 ) ) ;
#14214=CARTESIAN_POINT ( 'NONE',  ( 32.78867513459481842, 155.0000000000000000, -15.00000000000002487 ) ) ;
#14215=ORIENTED_EDGE ( 'NONE', *, *, #32690, .F. ) ;
#14223=ORIENTED_EDGE ( 'NONE', *, *, #11401, .F. ) ;
#14225=ORIENTED_EDGE ( 'NONE', *, *, #10184, .T. ) ;
#14227=( BOUNDED_CURVE ( )  B_SPLINE_CURVE ( 2, ( #32878, #12439, #30162, #4428, #27590, #6993, #29993, #19929, #25049, #6650, #30326 ),
 .UNSPECIFIED., .F., .T. ) 
 B_SPLINE_CURVE_WITH_KNOTS ( ( 3, 2, 2, 2, 2, 3 ),
 ( 0.9107142857142858094, 0.9142857142857143682, 0.9178571428571429269, 0.9214285714285713746, 0.9250000000000000444, 0.9285714285714286031 ),
 .UNSPECIFIED. ) 
 CURVE ( )  GEOMETRIC_REPRESENTATION_ITEM ( )  RATIONAL_B_SPLINE_CURVE ( ( 0.9999999999999984457, 0.9510565162951549745, 1.000000000000000000, 0.9510565162951534202, 1.000000000000000000, 0.9510565162951534202, 1.000000000000000000, 0.9510565162951534202, 1.000000000000000000, 0.9510565162951534202, 1.000000000000000000 ) ) 
 REPRESENTATION_ITEM ( '' )  );
#14229=VERTEX_POINT ( 'NONE', #2440 ) ;
#14230=CARTESIAN_POINT ( 'NONE',  ( 81.12499999726881583, 155.0000000000000000, -15.58253175000000823 ) ) ;
#14232=CARTESIAN_POINT ( 'NONE',  ( 68.71132485994280614, 155.0000000000000000, 15.00000000000001243 ) ) ;
#14233=TOROIDAL_SURFACE ( 'NONE', #25670, 70.00000000000001421, 27.99999999999999645 ) ;
#14234=CARTESIAN_POINT ( 'NONE',  ( 79.12499999726881583, 155.0000000000000000, -15.58253175000000823 ) ) ;
#14236=CARTESIAN_POINT ( 'NONE',  ( 87.49999999999998579, 169.2633224522697333, 5.220106800459117125 ) ) ;
#14238=CARTESIAN_POINT ( 'NONE',  ( 34.60000000000000142, 159.7113355953771077, -14.50000000000000888 ) ) ;
#14245=CARTESIAN_POINT ( 'NONE',  ( 48.82499999726881157, 141.7447067706911810, -9.630534252274387086 ) ) ;
#14247=CARTESIAN_POINT ( 'NONE',  ( 41.41132485994280898, 142.2402378747194405, -9.270509831248439525 ) ) ;
#14262=CARTESIAN_POINT ( 'NONE',  ( 74.67499999726879878, 141.7447067706911810, 9.630534252274376428 ) ) ;
#14266=CARTESIAN_POINT ( 'NONE',  ( 81.27499999726877888, 149.9369285172503510, -15.58253175000000823 ) ) ;
#14272=CARTESIAN_POINT ( 'NONE',  ( 70.67499999726881299, 141.7447067706911810, 9.630534252274376428 ) ) ;
#14281=CARTESIAN_POINT ( 'NONE',  ( 87.97499999726882436, 169.8198683612136222, 4.815267126137181997 ) ) ;
#14284=CARTESIAN_POINT ( 'NONE',  ( 48.12499999726880873, 155.0000000000000000, 15.58253174999999402 ) ) ;
#14285=FACE_OUTER_BOUND ( 'NONE', #26171, .T. ) ;
#14286=CARTESIAN_POINT ( 'NONE',  ( 34.12499999726881583, 155.0000000000000000, 15.58253174999999402 ) ) ;
#14288=DIRECTION ( 'NONE',  ( 1.000000000000000000, 0.000000000000000000, 0.000000000000000000 ) ) ;
#14293=CARTESIAN_POINT ( 'NONE',  ( 32.50000000000000000, 155.0000000000000000, -6.938893903907228378E-15 ) ) ;
#14294=DIRECTION ( 'NONE',  ( 1.000000000000000000, 0.000000000000000000, 0.000000000000000000 ) ) ;
#14297=CARTESIAN_POINT ( 'NONE',  ( 68.69999999453763451, 167.3344367211045096, 8.961492836873468093 ) ) ;
#14298=VERTEX_POINT ( 'NONE', #10111 ) ;
#14320=CARTESIAN_POINT ( 'NONE',  ( 52.97499999726881015, 140.1801316387863778, -4.815267126137194431 ) ) ;
#14321=ORIENTED_EDGE ( 'NONE', *, *, #16565, .F. ) ;
#14327=ADVANCED_FACE ( 'NONE', ( #4990 ), #10449, .F. ) ;
#14328=CARTESIAN_POINT ( 'NONE',  ( 61.17499999726882010, 145.8408176439707802, -12.60653300113719588 ) ) ;
#14334=CARTESIAN_POINT ( 'NONE',  ( 78.40000000000000568, 150.2886644046228639, -14.50000000000000888 ) ) ;
#14340=CARTESIAN_POINT ( 'NONE',  ( 46.27499999726881441, 160.0630714827496206, 15.58253174999999402 ) ) ;
#14342=CARTESIAN_POINT ( 'NONE',  ( 80.32499999726880446, 145.8408176439707802, 12.60653300113718345 ) ) ;
#14343=VERTEX_POINT ( 'NONE', #12995 ) ;
#14345=CARTESIAN_POINT ( 'NONE',  ( 49.11132485994281183, 140.7341522555726669, 4.635254915624211769 ) ) ;
#14346=AXIS2_PLACEMENT_3D ( 'NONE', #9383, #20115, #30507 ) ;
#14347=CARTESIAN_POINT ( 'NONE',  ( 44.69999999453762030, 167.3344367211045096, 8.961492836873468093 ) ) ;
#14350=FACE_OUTER_BOUND ( 'NONE', #13024, .T. ) ;
#14351=CIRCLE ( 'NONE', #4010, 98.00000000000002842 ) ;
#14359=AXIS2_PLACEMENT_3D ( 'NONE', #29535, #584, #914 ) ;
#14368=CARTESIAN_POINT ( 'NONE',  ( 37.42499999726881299, 168.2552932293087906, -9.630534252274385310 ) ) ;
#14370=AXIS2_PLACEMENT_3D ( 'NONE', #26903, #21784, #21957 ) ;
#14374=CARTESIAN_POINT ( 'NONE',  ( 39.67499999726881299, 168.2552932293087906, -9.630534252274385310 ) ) ;
#14377=CARTESIAN_POINT ( 'NONE',  ( 63.50000000000000000, 155.0000000000000000, 14.49999999999999467 ) ) ;
#14382=( BOUNDED_CURVE ( )  B_SPLINE_CURVE ( 2, ( #14560, #19169, #11508, #32445, #19674, #940, #11174, #24623, #26832, #1449, #11842 ),
 .UNSPECIFIED., .F., .T. ) 
 B_SPLINE_CURVE_WITH_KNOTS ( ( 3, 2, 2, 2, 2, 3 ),
 ( 0.5178571428571429047, 0.5214285714285714635, 0.5250000000000000222, 0.5285714285714284699, 0.5321428571428570287, 0.5357142857142855874 ),
 .UNSPECIFIED. ) 
 CURVE ( )  GEOMETRIC_REPRESENTATION_ITEM ( )  RATIONAL_B_SPLINE_CURVE ( ( 1.000000000000000000, 0.9510565162951534202, 1.000000000000000000, 0.9510565162951534202, 1.000000000000000000, 0.9510565162951534202, 1.000000000000000000, 0.9510565162951534202, 1.000000000000000000, 0.9510565162951549745, 0.9999999999999984457 ) ) 
 REPRESENTATION_ITEM ( '' )  );
#14383=CARTESIAN_POINT ( 'NONE',  ( 62.42499999726881299, 141.7447067706911810, 9.630534252274376428 ) ) ;
#14387=CARTESIAN_POINT ( 'NONE',  ( 85.47499999726879594, 160.0630714827496206, -15.58253175000000823 ) ) ;
#14389=CARTESIAN_POINT ( 'NONE',  ( 71.88867513459481984, 150.1262045565060816, 14.99999999999978328 ) ) ;
#14390=CARTESIAN_POINT ( 'NONE',  ( 53.38867513459481984, 169.2658477444273331, 4.635254915624208216 ) ) ;
#14399=EDGE_CURVE ( 'NONE', #2009, #8990, #19099, .T. ) ;
#14401=ORIENTED_EDGE ( 'NONE', *, *, #12476, .T. ) ;
#14402=DIRECTION ( 'NONE',  ( -1.000000000000000000, -0.000000000000000000, -0.000000000000000000 ) ) ;
#14406=CARTESIAN_POINT ( 'NONE',  ( 82.32499999726880446, 145.8408176439707802, 12.60653300113718345 ) ) ;
#14407=ORIENTED_EDGE ( 'NONE', *, *, #10231, .F. ) ;
#14408=CARTESIAN_POINT ( 'NONE',  ( 79.22499999726879594, 160.0630714827496206, -15.58253175000000823 ) ) ;
#14409=FACE_OUTER_BOUND ( 'NONE', #9837, .T. ) ;
#14411=CARTESIAN_POINT ( 'NONE',  ( 87.50000000000004263, 170.3440178963778351, 0.6416442768189705159 ) ) ;
#14412=CARTESIAN_POINT ( 'NONE',  ( 40.30000000000000426, 146.4771138417591203, -11.73074641843674470 ) ) ;
#14417=CARTESIAN_POINT ( 'NONE',  ( 48.02499999726879309, 160.0630714827496206, 15.58253174999999224 ) ) ;
#14424=CARTESIAN_POINT ( 'NONE',  ( 84.99999999453764588, 155.0000000000000000, 14.49999999999999467 ) ) ;
#14429=CYLINDRICAL_SURFACE ( 'NONE', #16140, 15.00000000000001776 ) ;
#14433=CARTESIAN_POINT ( 'NONE',  ( 72.87499999726881583, 138.6155565068815463, -3.929120461958505118E-15 ) ) ;
#14437=CARTESIAN_POINT ( 'NONE',  ( 82.07499999726880446, 168.2552932293087906, 9.630534252274372875 ) ) ;
#14439=CARTESIAN_POINT ( 'NONE',  ( 125.5000000000000000, 155.0000000000010800, 106.0000000000000142 ) ) ;
#14445=CARTESIAN_POINT ( 'NONE',  ( 48.78867513459482552, 155.0000000000000000, -15.00000000000002487 ) ) ;
#14450=CARTESIAN_POINT ( 'NONE',  ( 71.21132485994279193, 139.2280666364260071, -4.041636747397287284E-15 ) ) ;
#14453=CARTESIAN_POINT ( 'NONE',  ( 42.72499999726881015, 140.1801316387863778, -4.815267126137194431 ) ) ;
#14459=DIRECTION ( 'NONE',  ( 1.000000000000000000, 0.000000000000000000, 0.000000000000000000 ) ) ;
#14463=CARTESIAN_POINT ( 'NONE',  ( 69.39999999453763735, 141.2096805137202580, 4.480746418436733158 ) ) ;
#14473=DIRECTION ( 'NONE',  ( 0.000000000000000000, 0.000000000000000000, -1.000000000000000000 ) ) ;
#14475=EDGE_LOOP ( 'NONE', ( #11050, #28246, #11436, #23536 ) ) ;
#14480=CARTESIAN_POINT ( 'NONE',  ( 48.47499999726881015, 149.9369285172503510, 15.58253174999999580 ) ) ;
#14481=ORIENTED_EDGE ( 'NONE', *, *, #31027, .F. ) ;
#14484=CARTESIAN_POINT ( 'NONE',  ( 125.5000000000000000, 155.0000000000000000, -6.938893903907228378E-15 ) ) ;
#14486=CARTESIAN_POINT ( 'NONE',  ( 59.07499999726880446, 141.7447067706911810, -9.630534252274385310 ) ) ;
#14488=CARTESIAN_POINT ( 'NONE',  ( 69.98867513459484258, 146.1832212156128890, 12.13525491562421976 ) ) ;
#14492=EDGE_CURVE ( 'NONE', #31949, #20089, #10495, .T. ) ;
#14494=CARTESIAN_POINT ( 'NONE',  ( 77.70000000000000284, 146.4771138417591203, 11.73074641843673227 ) ) ;
#14498=CARTESIAN_POINT ( 'NONE',  ( 42.67499999726880588, 141.7447067706911810, 9.630534252274376428 ) ) ;
#14501=CARTESIAN_POINT ( 'NONE',  ( 85.92499999726881299, 164.1591823560292198, 12.60653300113718167 ) ) ;
#14503=DIRECTION ( 'NONE',  ( 0.000000000000000000, 0.000000000000000000, -1.000000000000000000 ) ) ;
#14504=CARTESIAN_POINT ( 'NONE',  ( 50.09999999453762598, 159.7113355953771077, -14.50000000000000888 ) ) ;
#14515=VECTOR ( 'NONE', #543, 1000.000000000000000 ) ;
#14516=CARTESIAN_POINT ( 'NONE',  ( 49.88867513459483405, 150.1262045565061385, 14.99999999999982947 ) ) ;
#14523=AXIS2_PLACEMENT_3D ( 'NONE', #267, #15919, #10984 ) ;
#14525=CARTESIAN_POINT ( 'NONE',  ( 34.92499999726881299, 145.8408176439707802, -12.60653300113719588 ) ) ;
#14526=DIRECTION ( 'NONE',  ( 1.000000000000000000, 0.000000000000000000, 0.000000000000000000 ) ) ;
#14529=CARTESIAN_POINT ( 'NONE',  ( 39.17499999726881299, 145.8408176439707802, -12.60653300113719588 ) ) ;
#14534=CARTESIAN_POINT ( 'NONE',  ( 58.10000000000000142, 141.2096805137202580, -4.480746418436742040 ) ) ;
#14541=CARTESIAN_POINT ( 'NONE',  ( 67.02499999726882152, 149.9369285172503510, -15.58253175000000823 ) ) ;
#14545=CIRCLE ( 'NONE', #6860, 2.149999999999985256 ) ;
#14547=CARTESIAN_POINT ( 'NONE',  ( 83.37499999726881583, 155.0000000000000000, -15.58253175000000823 ) ) ;
#14549=EDGE_CURVE ( 'NONE', #20617, #24401, #16203, .T. ) ;
#14560=CARTESIAN_POINT ( 'NONE',  ( 62.71132485994281325, 155.0000000000000000, 15.00000000000001243 ) ) ;
#14566=AXIS2_PLACEMENT_3D ( 'NONE', #538, #5794, #16192 ) ;
#14567=CARTESIAN_POINT ( 'NONE',  ( 86.02499999726880731, 160.0630714827496206, 15.58253174999999224 ) ) ;
#14569=CARTESIAN_POINT ( 'NONE',  ( 69.48867513459482836, 167.7597621252805880, 9.270509831248428867 ) ) ;
#14570=CARTESIAN_POINT ( 'NONE',  ( 74.72499999726881015, 140.1801316387863778, -4.815267126137194431 ) ) ;
#14572=( BOUNDED_CURVE ( )  B_SPLINE_CURVE ( 2, ( #20046, #14756, #28048, #4374, #32360, #4709, #2165, #12548, #32985, #33335, #3749 ),
 .UNSPECIFIED., .F., .T. ) 
 B_SPLINE_CURVE_WITH_KNOTS ( ( 3, 2, 2, 2, 2, 3 ),
 ( 0.2321428571428568455, 0.2357142857142854042, 0.2392857142857139352, 0.2428571428571424939, 0.2464285714285710249, 0.2499999999999996947 ),
 .UNSPECIFIED. ) 
 CURVE ( )  GEOMETRIC_REPRESENTATION_ITEM ( )  RATIONAL_B_SPLINE_CURVE ( ( 1.000000000000003331, 0.9510565162951499785, 1.000000000000000000, 0.9510565162951534202, 1.000000000000000000, 0.9510565162951534202, 1.000000000000000000, 0.9510565162951534202, 1.000000000000000000, 0.9510565162951576390, 0.9999999999999957812 ) ) 
 REPRESENTATION_ITEM ( '' )  );
#14574=CARTESIAN_POINT ( 'NONE',  ( 75.38867513459481984, 169.2658477444273331, 4.635254915624208216 ) ) ;
#14576=CARTESIAN_POINT ( 'NONE',  ( 40.60000000000000142, 159.7113355953771077, -14.50000000000000888 ) ) ;
#14581=CARTESIAN_POINT ( 'NONE',  ( 78.38867513459481984, 140.7341522555726669, -4.635254915624220651 ) ) ;
#14582=FACE_OUTER_BOUND ( 'NONE', #32428, .T. ) ;
#14583=CARTESIAN_POINT ( 'NONE',  ( 52.82499999726880446, 141.7447067706911810, -9.630534252274387086 ) ) ;
#14584=CARTESIAN_POINT ( 'NONE',  ( 66.57499999726881867, 145.8408176439707802, 12.60653300113718345 ) ) ;
#14605=CARTESIAN_POINT ( 'NONE',  ( 69.67499999726878457, 168.2552932293087906, -9.630534252274385310 ) ) ;
#14608=CARTESIAN_POINT ( 'NONE',  ( 80.47499999726881015, 149.9369285172503510, 15.58253174999999580 ) ) ;
#14609=CARTESIAN_POINT ( 'NONE',  ( 32.50000000000000000, 155.0000000000000000, -6.938893903907228378E-15 ) ) ;
#14623=CARTESIAN_POINT ( 'NONE',  ( 38.01132485994281041, 167.7597621252805880, -9.270509831248443078 ) ) ;
#14627=CARTESIAN_POINT ( 'NONE',  ( 43.12499999726881583, 155.0000000000000000, -15.58253175000000823 ) ) ;
#14629=CARTESIAN_POINT ( 'NONE',  ( 34.52499999726880731, 140.1801316387863778, 4.815267126137185549 ) ) ;
#14634=FACE_OUTER_BOUND ( 'NONE', #2563, .T. ) ;
#14638=CARTESIAN_POINT ( 'NONE',  ( 64.39999999453763735, 168.7903194862797420, -4.480746418436745593 ) ) ;
#14644=CARTESIAN_POINT ( 'NONE',  ( 76.61132485994281183, 159.8737954434937478, 14.99999999999991651 ) ) ;
#14648=ORIENTED_EDGE ( 'NONE', *, *, #2945, .T. ) ;
#14655=CARTESIAN_POINT ( 'NONE',  ( 58.87499999726880873, 138.6155565068815747, -3.929120461958505118E-15 ) ) ;
#14658=FACE_OUTER_BOUND ( 'NONE', #15498, .T. ) ;
#14662=CARTESIAN_POINT ( 'NONE',  ( 65.57499999726881867, 164.1591823560292198, -12.60653300113719766 ) ) ;
#14667=CARTESIAN_POINT ( 'NONE',  ( 81.00000000000001421, 170.2462022514548323, -7.872454543227099337E-15 ) ) ;
#14672=CARTESIAN_POINT ( 'NONE',  ( 42.77499999726880731, 140.1801316387863778, 4.815267126137185549 ) ) ;
#14674=CARTESIAN_POINT ( 'NONE',  ( 80.62499999726880162, 138.6155565068815463, -3.929120461958505118E-15 ) ) ;
#14677=CARTESIAN_POINT ( 'NONE',  ( 44.99999999453763166, 155.0000000000000000, 14.49999999999999467 ) ) ;
#14683=CARTESIAN_POINT ( 'NONE',  ( 66.61132485994281183, 159.8737954434938615, 14.99999999999982592 ) ) ;
#14688=DIRECTION ( 'NONE',  ( 0.000000000000000000, 0.000000000000000000, 1.000000000000000000 ) ) ;
#14689=ORIENTED_EDGE ( 'NONE', *, *, #12085, .T. ) ;
#14693=CARTESIAN_POINT ( 'NONE',  ( 34.27499999726880731, 160.0630714827496206, 15.58253174999999224 ) ) ;
#14694=ORIENTED_EDGE ( 'NONE', *, *, #13689, .T. ) ;
#14695=CARTESIAN_POINT ( 'NONE',  ( 42.42499999726881299, 141.7447067706911810, 9.630534252274376428 ) ) ;
#14697=CARTESIAN_POINT ( 'NONE',  ( 54.71132485994280614, 155.0000000000000000, 15.00000000000001243 ) ) ;
#14699=CARTESIAN_POINT ( 'NONE',  ( 40.87499999726880873, 138.6155565068815463, -3.929120461958505118E-15 ) ) ;
#14703=CARTESIAN_POINT ( 'NONE',  ( 62.10000000000000142, 141.2096805137202580, -4.480746418436742040 ) ) ;
#14704=CARTESIAN_POINT ( 'NONE',  ( 63.71132485994279904, 155.0000000000000000, -15.00000000000002487 ) ) ;
#14709=CARTESIAN_POINT ( 'NONE',  ( 63.72499999726881015, 169.8198683612136222, 4.815267126137181997 ) ) ;
#14713=CARTESIAN_POINT ( 'NONE',  ( 83.07499999726880446, 141.7447067706911810, -9.630534252274385310 ) ) ;
#14727=DIRECTION ( 'NONE',  ( 1.000000000000000000, 0.000000000000000000, 0.000000000000000000 ) ) ;
#14732=CARTESIAN_POINT ( 'NONE',  ( 84.52499999726880731, 140.1801316387863778, 4.815267126137185549 ) ) ;
#14734=DIRECTION ( 'NONE',  ( 1.000000000000000000, 0.000000000000000000, 0.000000000000000000 ) ) ;
#14735=CARTESIAN_POINT ( 'NONE',  ( 75.82499999726881867, 168.2552932293087906, 9.630534252274372875 ) ) ;
#14739=CARTESIAN_POINT ( 'NONE',  ( 87.50000000000004263, 170.2753832955869484, 1.322035671867324513 ) ) ;
#14740=CARTESIAN_POINT ( 'NONE',  ( 42.00000000000000000, 139.7537977485451393, -4.138211985947621020E-15 ) ) ;
#14743=DIRECTION ( 'NONE',  ( -1.000000000000000000, 0.000000000000000000, -0.000000000000000000 ) ) ;
#14744=CARTESIAN_POINT ( 'NONE',  ( 78.08867513459483689, 142.2402378747194405, 9.270509831248432420 ) ) ;
#14746=CARTESIAN_POINT ( 'NONE',  ( 52.52499999726881441, 140.1801316387863778, 4.815267126137185549 ) ) ;
#14747=CARTESIAN_POINT ( 'NONE',  ( 62.57499999726881867, 145.8408176439707802, 12.60653300113718345 ) ) ;
#14756=CARTESIAN_POINT ( 'NONE',  ( 74.68867513459483121, 150.1262045565067069, -15.00000000000023981 ) ) ;
#14760=ORIENTED_EDGE ( 'NONE', *, *, #13490, .F. ) ;
#14764=CARTESIAN_POINT ( 'NONE',  ( 78.67499999726879878, 141.7447067706911810, 9.630534252274376428 ) ) ;
#14767=( BOUNDED_CURVE ( )  B_SPLINE_CURVE ( 2, ( #26364, #11193, #6066, #475, #13911, #18535, #31964, #28917, #3518, #10872, #13248 ),
 .UNSPECIFIED., .F., .T. ) 
 B_SPLINE_CURVE_WITH_KNOTS ( ( 3, 2, 2, 2, 2, 3 ),
 ( 0.4821428571428570398, 0.4857142857142855985, 0.4892857142857141572, 0.4928571428571427715, 0.4964285714285713302, 0.4999999999999998890 ),
 .UNSPECIFIED. ) 
 CURVE ( )  GEOMETRIC_REPRESENTATION_ITEM ( )  RATIONAL_B_SPLINE_CURVE ( ( 1.000000000000000666, 0.9510565162951526430, 1.000000000000000000, 0.9510565162951534202, 1.000000000000000000, 0.9510565162951534202, 1.000000000000000000, 0.9510565162951534202, 1.000000000000000000, 0.9510565162951541973, 0.9999999999999992228 ) ) 
 REPRESENTATION_ITEM ( '' )  );
#14770=CARTESIAN_POINT ( 'NONE',  ( 83.47499999726881015, 160.0630714827496206, -15.58253175000000823 ) ) ;
#14771=CARTESIAN_POINT ( 'NONE',  ( 56.71132485994280614, 155.0000000000000000, 15.00000000000001243 ) ) ;
#14772=DIRECTION ( 'NONE',  ( 1.000000000000000000, 0.000000000000000000, 0.000000000000000000 ) ) ;
#14773=CARTESIAN_POINT ( 'NONE',  ( 59.62499999726882294, 171.3844434931184253, -7.942151717890132712E-15 ) ) ;
#14775=DIRECTION ( 'NONE',  ( 1.000000000000000000, 0.000000000000000000, 0.000000000000000000 ) ) ;
#14780=CARTESIAN_POINT ( 'NONE',  ( 85.91132485994280898, 163.8167787843871110, -12.13525491562423397 ) ) ;
#14788=CARTESIAN_POINT ( 'NONE',  ( 47.42499999726879878, 168.2552932293087906, -9.630534252274385310 ) ) ;
#14790=CARTESIAN_POINT ( 'NONE',  ( 33.62499999726880873, 171.3844434931184253, -7.942151717890134290E-15 ) ) ;
#14795=UNCERTAINTY_MEASURE_WITH_UNIT (LENGTH_MEASURE( 1.000000000000000082E-05 ), #17725, 'distance_accuracy_value', 'NONE');
#14797=CARTESIAN_POINT ( 'NONE',  ( 54.08867513459482979, 142.2402378747194405, 9.270509831248432420 ) ) ;
#14800=CARTESIAN_POINT ( 'NONE',  ( 71.09999999453761177, 150.2886644046228639, 14.49999999999999645 ) ) ;
#14807=ORIENTED_EDGE ( 'NONE', *, *, #8459, .F. ) ;
#14808=VERTEX_POINT ( 'NONE', #5900 ) ;
#14809=EDGE_LOOP ( 'NONE', ( #26267, #17366, #29347, #31334 ) ) ;
#14811=CARTESIAN_POINT ( 'NONE',  ( 57.78867513459481842, 155.0000000000000000, 15.00000000000001243 ) ) ;
#14818=CARTESIAN_POINT ( 'NONE',  ( 54.97499999726881015, 140.1801316387863778, -4.815267126137194431 ) ) ;
#14821=LINE ( 'NONE', #19934, #11819 ) ;
#14826=CARTESIAN_POINT ( 'NONE',  ( 65.27499999726880731, 149.9369285172503510, -15.58253175000000823 ) ) ;
#14828=CARTESIAN_POINT ( 'NONE',  ( 70.58867513459482268, 146.1832212156128890, -12.13525491562423042 ) ) ;
#14831=CARTESIAN_POINT ( 'NONE',  ( 81.50000000000000000, 155.0000000000000000, 14.49999999999999467 ) ) ;
#14836=CARTESIAN_POINT ( 'NONE',  ( 49.87499999726880162, 171.3844434931184253, -7.942151717890132712E-15 ) ) ;
#14838=CARTESIAN_POINT ( 'NONE',  ( 80.92499999726882720, 145.8408176439707802, -12.60653300113719588 ) ) ;
#14842=CARTESIAN_POINT ( 'NONE',  ( 53.09999999453761887, 150.2886644046228639, 14.49999999999999645 ) ) ;
#14845=CARTESIAN_POINT ( 'NONE',  ( 61.51132485994280330, 146.1832212156128890, -12.13525491562423042 ) ) ;
#14856=CARTESIAN_POINT ( 'NONE',  ( 125.5000000000000000, 78.52640161467446944, -73.43303922622258995 ) ) ;
#14859=LINE ( 'NONE', #25255, #3985 ) ;
#14861=CARTESIAN_POINT ( 'NONE',  ( 37.37499999726881583, 155.0000000000000000, -15.58253175000000823 ) ) ;
#14863=CARTESIAN_POINT ( 'NONE',  ( 44.42499999726881299, 141.7447067706911810, 9.630534252274376428 ) ) ;
#14865=CARTESIAN_POINT ( 'NONE',  ( 54.61132485994280472, 159.8737954434937478, 14.99999999999991651 ) ) ;
#14867=CARTESIAN_POINT ( 'NONE',  ( 46.17499999726881299, 164.1591823560292198, 12.60653300113718167 ) ) ;
#14874=CARTESIAN_POINT ( 'NONE',  ( 62.79999999999999716, 167.3344367211045096, -8.961492836873482304 ) ) ;
#14882=AXIS2_PLACEMENT_3D ( 'NONE', #5300, #30524, #12467 ) ;
#14883=CARTESIAN_POINT ( 'NONE',  ( 63.92499999726880588, 164.1591823560292198, 12.60653300113718167 ) ) ;
#14886=CARTESIAN_POINT ( 'NONE',  ( 43.01132485994281751, 142.2402378747194405, 9.270509831248432420 ) ) ;
#14887=CARTESIAN_POINT ( 'NONE',  ( 81.97499999726881015, 169.8198683612136222, 4.815267126137181997 ) ) ;
#14901=ORIENTED_EDGE ( 'NONE', *, *, #2242, .F. ) ;
#14907=ORIENTED_EDGE ( 'NONE', *, *, #6797, .F. ) ;
#14910=CARTESIAN_POINT ( 'NONE',  ( 73.07499999726880446, 141.7447067706911810, -9.630534252274387086 ) ) ;
#14911=CARTESIAN_POINT ( 'NONE',  ( 79.72499999726881015, 169.8198683612136222, 4.815267126137181997 ) ) ;
#14917=CARTESIAN_POINT ( 'NONE',  ( 42.79999999999999716, 167.3344367211045096, -8.961492836873482304 ) ) ;
#14925=CARTESIAN_POINT ( 'NONE',  ( 54.92499999726881299, 145.8408176439707802, -12.60653300113719588 ) ) ;
#14926=CARTESIAN_POINT ( 'NONE',  ( 62.67499999726879878, 141.7447067706911810, 9.630534252274376428 ) ) ;
#14943=CARTESIAN_POINT ( 'NONE',  ( 75.67499999726881299, 168.2552932293087906, -9.630534252274385310 ) ) ;
#14947=CARTESIAN_POINT ( 'NONE',  ( 70.12499999726881583, 155.0000000000000000, 15.58253174999999402 ) ) ;
#14950=CARTESIAN_POINT ( 'NONE',  ( 57.12499999726880873, 155.0000000000000000, -15.58253175000000823 ) ) ;
#14954=ORIENTED_EDGE ( 'NONE', *, *, #23067, .F. ) ;
#14964=CARTESIAN_POINT ( 'NONE',  ( 32.50000000000000000, 155.0000000000000000, -6.938893903907228378E-15 ) ) ;
#14976=CARTESIAN_POINT ( 'NONE',  ( 74.79999999453762882, 163.5228861582408797, 11.73074641843673049 ) ) ;
#14982=CARTESIAN_POINT ( 'NONE',  ( 75.61132485994281183, 150.1262045565064227, -15.00000000000002665 ) ) ;
#14993=CARTESIAN_POINT ( 'NONE',  ( 53.97499999726881015, 169.8198683612136222, 4.815267126137181997 ) ) ;
#14999=CARTESIAN_POINT ( 'NONE',  ( 65.07499999726881867, 141.7447067706911810, -9.630534252274385310 ) ) ;
#15004=CARTESIAN_POINT ( 'NONE',  ( 84.00000000000000000, 139.7537977485451393, -4.138211985947621020E-15 ) ) ;
#15009=CARTESIAN_POINT ( 'NONE',  ( 49.27499999726880020, 149.9369285172503510, -15.58253175000000823 ) ) ;
#15012=ADVANCED_FACE ( 'NONE', ( #6917 ), #22584, .T. ) ;
#15013=CARTESIAN_POINT ( 'NONE',  ( 84.52499999726880731, 140.1801316387863778, 4.815267126137185549 ) ) ;
#15015=CARTESIAN_POINT ( 'NONE',  ( 54.49999999453761745, 170.2462022514548323, -7.872454543227099337E-15 ) ) ;
#15016=ORIENTED_EDGE ( 'NONE', *, *, #6413, .T. ) ;
#15017=( BOUNDED_CURVE ( )  B_SPLINE_CURVE ( 2, ( #24051, #21829, #3435, #32060, #8722, #558, #10951, #6156, #16550, #3604, #13998 ),
 .UNSPECIFIED., .F., .F. ) 
 B_SPLINE_CURVE_WITH_KNOTS ( ( 3, 2, 2, 2, 2, 3 ),
 ( 0.9642857142857140795, 0.9678571428571427493, 0.9714285714285713080, 0.9749999999999999778, 0.9785714285714285365, 0.9821428571428570953 ),
 .UNSPECIFIED. ) 
 CURVE ( )  GEOMETRIC_REPRESENTATION_ITEM ( )  RATIONAL_B_SPLINE_CURVE ( ( 1.000000000000001554, 0.9510565162951518658, 1.000000000000000000, 0.9510565162951534202, 1.000000000000000000, 0.9510565162951534202, 1.000000000000000000, 0.9510565162951534202, 1.000000000000000000, 0.9510565162951534202, 1.000000000000000000 ) ) 
 REPRESENTATION_ITEM ( '' )  );
#15020=FACE_OUTER_BOUND ( 'NONE', #20013, .T. ) ;
#15032=CARTESIAN_POINT ( 'NONE',  ( 39.67499999726881299, 168.2552932293087906, -9.630534252274387086 ) ) ;
#15033=EDGE_LOOP ( 'NONE', ( #6372, #1524 ) ) ;
#15034=CARTESIAN_POINT ( 'NONE',  ( 45.72499999726881015, 169.8198683612136222, 4.815267126137181997 ) ) ;
#15038=CARTESIAN_POINT ( 'NONE',  ( 48.47499999726880304, 149.9369285172503510, 15.58253174999999580 ) ) ;
#15043=CARTESIAN_POINT ( 'NONE',  ( 59.10000000000000142, 168.7903194862797420, 4.480746418436729606 ) ) ;
#15050=CARTESIAN_POINT ( 'NONE',  ( 63.02499999726882152, 149.9369285172503510, -15.58253175000000823 ) ) ;
#15052=ORIENTED_EDGE ( 'NONE', *, *, #13490, .T. ) ;
#15054=CARTESIAN_POINT ( 'NONE',  ( 34.29999999453762882, 167.3344367211045096, -8.961492836873482304 ) ) ;
#15068=CARTESIAN_POINT ( 'NONE',  ( 70.31132485994280046, 169.2658477444273331, 4.635254915624208216 ) ) ;
#15071=CARTESIAN_POINT ( 'NONE',  ( 69.71132485994280614, 155.0000000000000000, -15.00000000000002487 ) ) ;
#15075=CARTESIAN_POINT ( 'NONE',  ( 83.72499999726882436, 169.8198683612136222, 4.815267126137181997 ) ) ;
#15082=CARTESIAN_POINT ( 'NONE',  ( 39.59999999999999432, 150.2886644046228639, 14.49999999999999645 ) ) ;
#15088=CARTESIAN_POINT ( 'NONE',  ( 56.62499999726880162, 138.6155565068815747, -3.929120461958505118E-15 ) ) ;
#15089=CARTESIAN_POINT ( 'NONE',  ( 70.87499999726878741, 138.6155565068815463, -3.929120461958505118E-15 ) ) ;
#15091=CARTESIAN_POINT ( 'NONE',  ( 45.81132485994281467, 159.8737954434936910, -14.99999999999998046 ) ) ;
#15098=DIRECTION ( 'NONE',  ( 1.000000000000000000, 0.000000000000000000, 0.000000000000000000 ) ) ;
#15108=CARTESIAN_POINT ( 'NONE',  ( 78.17499999726881299, 164.1591823560292198, 12.60653300113718167 ) ) ;
#15112=CARTESIAN_POINT ( 'NONE',  ( 69.42499999726881299, 168.2552932293087906, -9.630534252274387086 ) ) ;
#15113=LINE ( 'NONE', #30626, #20041 ) ;
#15115=CARTESIAN_POINT ( 'NONE',  ( 65.52499999726880731, 169.8198683612136222, -4.815267126137197984 ) ) ;
#15122=CARTESIAN_POINT ( 'NONE',  ( 86.31132485994280046, 169.2658477444273331, 4.635254915624208216 ) ) ;
#15128=AXIS2_PLACEMENT_3D ( 'NONE', #25982, #20703, #12532 ) ;
#15132=CARTESIAN_POINT ( 'NONE',  ( 40.72499999726881725, 140.1801316387863778, -4.815267126137194431 ) ) ;
#15140=CARTESIAN_POINT ( 'NONE',  ( 78.78867513459481131, 155.0000000000000000, -15.00000000000002487 ) ) ;
#15143=CARTESIAN_POINT ( 'NONE',  ( 73.29999999453762882, 142.6655632788954620, 8.961492836873471646 ) ) ;
#15157=EDGE_CURVE ( 'NONE', #25537, #8808, #29926, .T. ) ;
#15159=EDGE_LOOP ( 'NONE', ( #20732, #24199, #6881, #28538 ) ) ;
#15163=CARTESIAN_POINT ( 'NONE',  ( 55.67499999726880588, 168.2552932293087906, -9.630534252274387086 ) ) ;
#15170=CARTESIAN_POINT ( 'NONE',  ( 66.77499999726880731, 140.1801316387863778, 4.815267126137185549 ) ) ;
#15172=CARTESIAN_POINT ( 'NONE',  ( 69.78867513459482552, 155.0000000000000000, 15.00000000000001243 ) ) ;
#15175=CARTESIAN_POINT ( 'NONE',  ( 32.50000000000000000, 155.0000000000000000, -6.938893903907228378E-15 ) ) ;
#15176=CARTESIAN_POINT ( 'NONE',  ( 84.19999999999998863, 142.6655632788954620, -8.961492836873480528 ) ) ;
#15178=DIRECTION ( 'NONE',  ( 1.000000000000000000, 0.000000000000000000, 0.000000000000000000 ) ) ;
#15181=CARTESIAN_POINT ( 'NONE',  ( 48.07499999726881867, 168.2552932293087906, 9.630534252274372875 ) ) ;
#15182=EDGE_CURVE ( 'NONE', #14808, #5021, #27698, .T. ) ;
#15184=DIRECTION ( 'NONE',  ( 1.000000000000000000, 0.000000000000000000, 0.000000000000000000 ) ) ;
#15189=CARTESIAN_POINT ( 'NONE',  ( 56.89999999453762314, 159.7113355953771077, 14.49999999999999289 ) ) ;
#15192=CARTESIAN_POINT ( 'NONE',  ( 47.51132485994280330, 146.1832212156128890, -12.13525491562423042 ) ) ;
#15206=CARTESIAN_POINT ( 'NONE',  ( 40.07499999726880446, 168.2552932293087906, 9.630534252274372875 ) ) ;
#15208=CARTESIAN_POINT ( 'NONE',  ( 46.22499999726880304, 149.9369285172503510, 15.58253174999999580 ) ) ;
#15212=CARTESIAN_POINT ( 'NONE',  ( 45.07499999726880446, 141.7447067706911810, -9.630534252274385310 ) ) ;
#15213=DIRECTION ( 'NONE',  ( -1.000000000000000000, -0.000000000000000000, -0.000000000000000000 ) ) ;
#15216=EDGE_CURVE ( 'NONE', #14343, #4684, #7771, .T. ) ;
#15217=CARTESIAN_POINT ( 'NONE',  ( 69.90000000000000568, 141.2096805137202580, 4.480746418436733158 ) ) ;
#15222=CARTESIAN_POINT ( 'NONE',  ( 33.97499999726881725, 169.8198683612136222, 4.815267126137181997 ) ) ;
#15225=CARTESIAN_POINT ( 'NONE',  ( 70.32499999726881867, 145.8408176439707802, 12.60653300113718345 ) ) ;
#15228=CARTESIAN_POINT ( 'NONE',  ( 43.61132485994281183, 150.1262045565064511, -15.00000000000005151 ) ) ;
#15229=CARTESIAN_POINT ( 'NONE',  ( 35.89999999453763024, 150.2886644046228639, -14.50000000000000888 ) ) ;
#15238=CARTESIAN_POINT ( 'NONE',  ( 66.68867513459485963, 150.1262045565066785, -15.00000000000021316 ) ) ;
#15245=CARTESIAN_POINT ( 'NONE',  ( 39.78867513459481842, 155.0000000000000000, 15.00000000000001243 ) ) ;
#15249=CARTESIAN_POINT ( 'NONE',  ( 81.82499999726879025, 168.2552932293087906, 9.630534252274372875 ) ) ;
#15254=CARTESIAN_POINT ( 'NONE',  ( 46.10000000000000142, 141.2096805137202580, -4.480746418436742040 ) ) ;
#15258=CARTESIAN_POINT ( 'NONE',  ( 50.71132485994280614, 155.0000000000000000, 15.00000000000001243 ) ) ;
#15261=CARTESIAN_POINT ( 'NONE',  ( 57.92499999726881299, 164.1591823560292198, 12.60653300113718167 ) ) ;
#15262=CARTESIAN_POINT ( 'NONE',  ( 67.47499999726879594, 160.0630714827496206, -15.58253175000000823 ) ) ;
#15279=CARTESIAN_POINT ( 'NONE',  ( 75.77499999726880731, 169.8198683612136222, -4.815267126137197984 ) ) ;
#15281=EDGE_LOOP ( 'NONE', ( #20397, #26221, #9029, #8524 ) ) ;
#15282=CARTESIAN_POINT ( 'NONE',  ( 69.52499999726880731, 169.8198683612136222, -4.815267126137197984 ) ) ;
#15285=CARTESIAN_POINT ( 'NONE',  ( 64.32499999726881867, 145.8408176439707802, 12.60653300113718345 ) ) ;
#15293=FACE_OUTER_BOUND ( 'NONE', #22138, .T. ) ;
#15302=CARTESIAN_POINT ( 'NONE',  ( 35.62499999726881583, 171.3844434931184253, -7.942151717890134290E-15 ) ) ;
#15304=DIRECTION ( 'NONE',  ( 0.000000000000000000, 0.000000000000000000, -1.000000000000000000 ) ) ;
#15307=DIRECTION ( 'NONE',  ( 1.000000000000000000, 0.000000000000000000, 0.000000000000000000 ) ) ;
#15310=VECTOR ( 'NONE', #6836, 1000.000000000000000 ) ;
#15311=CARTESIAN_POINT ( 'NONE',  ( 74.99999999453763166, 155.0000000000000000, 14.49999999999999467 ) ) ;
#15321=DIRECTION ( 'NONE',  ( 1.000000000000000000, 0.000000000000000000, 0.000000000000000000 ) ) ;
#15324=( BOUNDED_CURVE ( )  B_SPLINE_CURVE ( 2, ( #11769, #31717, #3428, #13991, #31878, #19106, #8389, #24387, #9045, #29841, #13824 ),
 .UNSPECIFIED., .F., .T. ) 
 B_SPLINE_CURVE_WITH_KNOTS ( ( 3, 2, 2, 2, 2, 3 ),
 ( 0.7142857142857140795, 0.7178571428571426383, 0.7214285714285711970, 0.7249999999999998668, 0.7285714285714284255, 0.7321428571428569843 ),
 .UNSPECIFIED. ) 
 CURVE ( )  GEOMETRIC_REPRESENTATION_ITEM ( )  RATIONAL_B_SPLINE_CURVE ( ( 1.000000000000001554, 0.9510565162951518658, 1.000000000000000000, 0.9510565162951534202, 1.000000000000000000, 0.9510565162951534202, 1.000000000000000000, 0.9510565162951534202, 1.000000000000000000, 0.9510565162951549745, 0.9999999999999984457 ) ) 
 REPRESENTATION_ITEM ( '' )  );
#15328=CARTESIAN_POINT ( 'NONE',  ( 57.97499999726881015, 169.8198683612136222, 4.815267126137181997 ) ) ;
#15344=CARTESIAN_POINT ( 'NONE',  ( 86.90000000000000568, 168.7903194862797420, -4.480746418436745593 ) ) ;
#15349=CARTESIAN_POINT ( 'NONE',  ( 48.28867513459482552, 139.2280666364260071, -4.041636747397287284E-15 ) ) ;
#15350=CARTESIAN_POINT ( 'NONE',  ( 48.57499999726881157, 145.8408176439707802, 12.60653300113718345 ) ) ;
#15352=CARTESIAN_POINT ( 'NONE',  ( 125.5000000000000000, 155.0000000000010800, 106.0000000000000142 ) ) ;
#15356=CARTESIAN_POINT ( 'NONE',  ( 51.19999999453762740, 146.4771138417591203, 11.73074641843673227 ) ) ;
#15359=CARTESIAN_POINT ( 'NONE',  ( 46.71132485994281325, 155.0000000000000000, 15.00000000000001243 ) ) ;
#15361=VERTEX_POINT ( 'NONE', #19496 ) ;
#15366=VERTEX_POINT ( 'NONE', #19665 ) ;
#15371=ADVANCED_FACE ( 'NONE', ( #30568 ), #30056, .F. ) ;
#15374=CARTESIAN_POINT ( 'NONE',  ( 38.87499999726880873, 138.6155565068815747, -3.929120461958505118E-15 ) ) ;
#15376=CARTESIAN_POINT ( 'NONE',  ( 45.42499999726879878, 168.2552932293087906, -9.630534252274385310 ) ) ;
#15380=CARTESIAN_POINT ( 'NONE',  ( 48.27499999726880731, 160.0630714827496206, 15.58253174999999402 ) ) ;
#15383=CARTESIAN_POINT ( 'NONE',  ( 44.68867513459483121, 150.1262045565065364, -15.00000000000012434 ) ) ;
#15385=CARTESIAN_POINT ( 'NONE',  ( 68.20000000000001705, 142.6655632788954620, -8.961492836873480528 ) ) ;
#15389=CARTESIAN_POINT ( 'NONE',  ( 57.78867513459481842, 155.0000000000000000, 15.00000000000001243 ) ) ;
#15390=CARTESIAN_POINT ( 'NONE',  ( 34.27499999726880731, 160.0630714827496206, 15.58253174999999402 ) ) ;
#15392=CARTESIAN_POINT ( 'NONE',  ( 73.62499999726883004, 171.3844434931184253, -7.942151717890132712E-15 ) ) ;
#15393=ORIENTED_EDGE ( 'NONE', *, *, #2722, .F. ) ;
#15396=CARTESIAN_POINT ( 'NONE',  ( 36.59999999453762598, 168.7903194862797420, 4.480746418436729606 ) ) ;
#15407=EDGE_CURVE ( 'NONE', #7020, #30153, #28986, .T. ) ;
#15413=EDGE_CURVE ( 'NONE', #19088, #3486, #1606, .T. ) ;
#15415=CARTESIAN_POINT ( 'NONE',  ( 34.11132485994280472, 169.2658477444273331, -4.635254915624224203 ) ) ;
#15420=CARTESIAN_POINT ( 'NONE',  ( 85.52499999726880731, 169.8198683612136222, -4.815267126137197984 ) ) ;
#15425=CARTESIAN_POINT ( 'NONE',  ( 49.60000000000000853, 150.2886644046228639, 14.49999999999999645 ) ) ;
#15428=CARTESIAN_POINT ( 'NONE',  ( 53.62499999726881583, 171.3844434931184253, -7.942151717890132712E-15 ) ) ;
#15429=AXIS2_PLACEMENT_3D ( 'NONE', #22579, #9810, #11689 ) ;
#15432=CARTESIAN_POINT ( 'NONE',  ( 59.32499999726881157, 164.1591823560292198, -12.60653300113719766 ) ) ;
#15433=CARTESIAN_POINT ( 'NONE',  ( 72.27499999726879309, 160.0630714827496206, 15.58253174999999402 ) ) ;
#15435=CARTESIAN_POINT ( 'NONE',  ( 46.51132485994280330, 163.8167787843871110, 12.13525491562421621 ) ) ;
#15447=EDGE_CURVE ( 'NONE', #24401, #18472, #11103, .T. ) ;
#15453=ORIENTED_EDGE ( 'NONE', *, *, #19475, .T. ) ;
#15454=CARTESIAN_POINT ( 'NONE',  ( 78.47499999726881015, 149.9369285172503510, 15.58253174999999580 ) ) ;
#15456=ORIENTED_EDGE ( 'NONE', *, *, #29333, .F. ) ;
#15457=CARTESIAN_POINT ( 'NONE',  ( 74.32499999726881867, 145.8408176439707802, 12.60653300113718345 ) ) ;
#15461=CARTESIAN_POINT ( 'NONE',  ( 63.12499999726880873, 155.0000000000000000, -15.58253175000000823 ) ) ;
#15476=CARTESIAN_POINT ( 'NONE',  ( 86.67499999726879878, 141.7447067706911810, 9.630534252274376428 ) ) ;
#15478=CARTESIAN_POINT ( 'NONE',  ( 37.72499999726881015, 169.8198683612136222, 4.815267126137181997 ) ) ;
#15487=CARTESIAN_POINT ( 'NONE',  ( 75.99999999453763166, 155.0000000000000000, -14.50000000000000711 ) ) ;
#15491=LINE ( 'NONE', #25882, #8019 ) ;
#15498=EDGE_LOOP ( 'NONE', ( #19419, #21337, #12486, #26624 ) ) ;
#15503=CARTESIAN_POINT ( 'NONE',  ( 62.27499999726880020, 160.0630714827496206, 15.58253174999999224 ) ) ;
#15512=CARTESIAN_POINT ( 'NONE',  ( 85.29999999999999716, 163.5228861582408797, 11.73074641843673049 ) ) ;
#15517=CARTESIAN_POINT ( 'NONE',  ( 53.47499999726881015, 160.0630714827496206, -15.58253175000000823 ) ) ;
#15519=CARTESIAN_POINT ( 'NONE',  ( 35.51132485994281041, 146.1832212156128890, -12.13525491562423042 ) ) ;
#15522=CARTESIAN_POINT ( 'NONE',  ( 54.59999999453762598, 168.7903194862797420, 4.480746418436729606 ) ) ;
#15525=CARTESIAN_POINT ( 'NONE',  ( 47.61132485994280472, 150.1262045565063659, -14.99999999999998046 ) ) ;
#15527=DIRECTION ( 'NONE',  ( 0.000000000000000000, -1.000000000000000000, 1.290957005378097920E-14 ) ) ;
#15529=( BOUNDED_CURVE ( )  B_SPLINE_CURVE ( 2, ( #27901, #2527, #12911, #20745, #31141, #25347, #30640, #9856, #7807, #18199, #137 ),
 .UNSPECIFIED., .F., .F. ) 
 B_SPLINE_CURVE_WITH_KNOTS ( ( 3, 2, 2, 2, 2, 3 ),
 ( 0.7499999999999997780, 0.7535714285714283367, 0.7571428571428568954, 0.7607142857142855652, 0.7642857142857141239, 0.7678571428571426827 ),
 .UNSPECIFIED. ) 
 CURVE ( )  GEOMETRIC_REPRESENTATION_ITEM ( )  RATIONAL_B_SPLINE_CURVE ( ( 1.000000000000003109, 0.9510565162951504226, 1.000000000000000000, 0.9510565162951534202, 1.000000000000000000, 0.9510565162951534202, 1.000000000000000000, 0.9510565162951534202, 1.000000000000000000, 0.9510565162951549745, 0.9999999999999984457 ) ) 
 REPRESENTATION_ITEM ( '' )  );
#15539=CARTESIAN_POINT ( 'NONE',  ( 43.87499999726880873, 171.3844434931184253, -7.942151717890134290E-15 ) ) ;
#15541=CARTESIAN_POINT ( 'NONE',  ( 51.82499999726881157, 168.2552932293087906, 9.630534252274372875 ) ) ;
#15545=CARTESIAN_POINT ( 'NONE',  ( 45.77499999726881441, 169.8198683612136222, -4.815267126137197984 ) ) ;
#15546=CARTESIAN_POINT ( 'NONE',  ( 79.21132485994282035, 139.2280666364260071, -4.041636747397287284E-15 ) ) ;
#15549=CARTESIAN_POINT ( 'NONE',  ( 70.20000000000001705, 142.6655632788954620, -8.961492836873480528 ) ) ;
#15555=CARTESIAN_POINT ( 'NONE',  ( 73.12499999726881583, 155.0000000000000000, -15.58253175000000823 ) ) ;
#15558=CARTESIAN_POINT ( 'NONE',  ( 37.49999999453762456, 139.7537977485451393, -4.138211985947621020E-15 ) ) ;
#15560=EDGE_CURVE ( 'NONE', #25621, #1492, #27828, .T. ) ;
#15578=CARTESIAN_POINT ( 'NONE',  ( 83.02499999726879309, 149.9369285172503510, -15.58253175000000823 ) ) ;
#15581=CARTESIAN_POINT ( 'NONE',  ( 89.50000000000001421, 155.0000000000000000, -6.938893903907228378E-15 ) ) ;
#15583=CARTESIAN_POINT ( 'NONE',  ( 51.29999999999999716, 163.5228861582408797, 11.73074641843673049 ) ) ;
#15588=CARTESIAN_POINT ( 'NONE',  ( 50.52499999726880731, 140.1801316387863778, 4.815267126137185549 ) ) ;
#15592=CARTESIAN_POINT ( 'NONE',  ( 58.42499999726880588, 141.7447067706911810, 9.630534252274376428 ) ) ;
#15593=CARTESIAN_POINT ( 'NONE',  ( 70.57499999726881867, 145.8408176439707802, 12.60653300113718345 ) ) ;
#15595=CARTESIAN_POINT ( 'NONE',  ( 41.61132485994280472, 150.1262045565064227, -15.00000000000002665 ) ) ;
#15598=AXIS2_PLACEMENT_3D ( 'NONE', #2446, #15213, #9940 ) ;
#15602=CARTESIAN_POINT ( 'NONE',  ( 34.58867513459482268, 146.1832212156128890, -12.13525491562423042 ) ) ;
#15612=ORIENTED_EDGE ( 'NONE', *, *, #31990, .F. ) ;
#15614=CARTESIAN_POINT ( 'NONE',  ( 72.32499999726880446, 145.8408176439707802, 12.60653300113718345 ) ) ;
#15618=CARTESIAN_POINT ( 'NONE',  ( 60.82499999726881867, 141.7447067706911810, -9.630534252274385310 ) ) ;
#15636=CARTESIAN_POINT ( 'NONE',  ( 36.12499999726881583, 155.0000000000000000, 15.58253174999999402 ) ) ;
#15649=CARTESIAN_POINT ( 'NONE',  ( 79.39999999453763735, 141.2096805137202580, 4.480746418436733158 ) ) ;
#15666=CARTESIAN_POINT ( 'NONE',  ( 63.07499999726881867, 141.7447067706911810, -9.630534252274387086 ) ) ;
#15667=ORIENTED_EDGE ( 'NONE', *, *, #17414, .F. ) ;
#15669=VECTOR ( 'NONE', #32631, 1000.000000000000000 ) ;
#15670=DIRECTION ( 'NONE',  ( 1.000000000000000000, 0.000000000000000000, 0.000000000000000000 ) ) ;
#15673=( BOUNDED_CURVE ( )  B_SPLINE_CURVE ( 2, ( #8851, #27871, #4546, #12378, #33168, #25840, #7620, #31613, #31454, #26165, #18004 ),
 .UNSPECIFIED., .F., .T. ) 
 B_SPLINE_CURVE_WITH_KNOTS ( ( 3, 2, 2, 2, 2, 3 ),
 ( 0.6071428571428569843, 0.6107142857142856540, 0.6142857142857142128, 0.6178571428571427715, 0.6214285714285713302, 0.6249999999999998890 ),
 .UNSPECIFIED. ) 
 CURVE ( )  GEOMETRIC_REPRESENTATION_ITEM ( )  RATIONAL_B_SPLINE_CURVE ( ( 1.000000000000001554, 0.9510565162951518658, 1.000000000000000000, 0.9510565162951534202, 1.000000000000000000, 0.9510565162951534202, 1.000000000000000000, 0.9510565162951534202, 1.000000000000000000, 0.9510565162951549745, 0.9999999999999984457 ) ) 
 REPRESENTATION_ITEM ( '' )  );
#15679=CARTESIAN_POINT ( 'NONE',  ( 86.60000000000000853, 159.7113355953771077, -14.50000000000000888 ) ) ;
#15684=CARTESIAN_POINT ( 'NONE',  ( 57.17499999726881299, 145.8408176439707802, -12.60653300113719588 ) ) ;
#15687=CARTESIAN_POINT ( 'NONE',  ( 65.01132485994280330, 142.2402378747194405, 9.270509831248432420 ) ) ;
#15688=CARTESIAN_POINT ( 'NONE',  ( 59.29999999453762882, 142.6655632788954620, 8.961492836873471646 ) ) ;
#15691=CARTESIAN_POINT ( 'NONE',  ( 47.21132485994281325, 139.2280666364260071, -4.041636747397287284E-15 ) ) ;
#15700=TOROIDAL_SURFACE ( 'NONE', #1541, 70.00000000000001421, 27.99999999999999645 ) ;
#15701=CARTESIAN_POINT ( 'NONE',  ( 44.41132485994282320, 167.7597621252805880, 9.270509831248428867 ) ) ;
#15702=VERTEX_POINT ( 'NONE', #12673 ) ;
#15705=CARTESIAN_POINT ( 'NONE',  ( 43.37499999726881583, 155.0000000000000000, -15.58253175000000823 ) ) ;
#15707=CARTESIAN_POINT ( 'NONE',  ( 52.52499999726881441, 140.1801316387863778, 4.815267126137185549 ) ) ;
#15712=CARTESIAN_POINT ( 'NONE',  ( 51.07499999726879736, 141.7447067706911810, -9.630534252274385310 ) ) ;
#15713=CARTESIAN_POINT ( 'NONE',  ( 78.91132485994282320, 146.1832212156128890, 12.13525491562421976 ) ) ;
#15718=CARTESIAN_POINT ( 'NONE',  ( 64.29999999999999716, 146.4771138417591203, -11.73074641843674470 ) ) ;
#15722=CARTESIAN_POINT ( 'NONE',  ( 32.50000000000000000, 155.0000000000000000, 15.00000000000001243 ) ) ;
#15723=CARTESIAN_POINT ( 'NONE',  ( 38.47499999726881015, 149.9369285172503510, 15.58253174999999580 ) ) ;
#15727=CARTESIAN_POINT ( 'NONE',  ( 69.22499999726881015, 160.0630714827496206, -15.58253175000000823 ) ) ;
#15730=CARTESIAN_POINT ( 'NONE',  ( 33.99999999453763166, 155.0000000000000000, -14.50000000000000711 ) ) ;
#15742=CARTESIAN_POINT ( 'NONE',  ( 74.21132485994283456, 170.7719333635740497, -7.904646289410545231E-15 ) ) ;
#15747=CARTESIAN_POINT ( 'NONE',  ( 80.78867513459482552, 155.0000000000000000, -15.00000000000002487 ) ) ;
#15750=CARTESIAN_POINT ( 'NONE',  ( 37.37499999726881583, 155.0000000000000000, -15.58253175000000823 ) ) ;
#15751=DIRECTION ( 'NONE',  ( 0.000000000000000000, 0.000000000000000000, -1.000000000000000000 ) ) ;
#15754=CARTESIAN_POINT ( 'NONE',  ( 47.10000000000000142, 168.7903194862797420, 4.480746418436729606 ) ) ;
#15759=CARTESIAN_POINT ( 'NONE',  ( 49.32499999726881157, 164.1591823560292198, -12.60653300113719766 ) ) ;
#15762=CARTESIAN_POINT ( 'NONE',  ( 61.22499999726880304, 160.0630714827496206, -15.58253175000000823 ) ) ;
#15763=CARTESIAN_POINT ( 'NONE',  ( 69.27499999726880731, 149.9369285172503510, -15.58253175000000823 ) ) ;
#15782=CARTESIAN_POINT ( 'NONE',  ( 75.52499999726880731, 169.8198683612136222, -4.815267126137197984 ) ) ;
#15787=ADVANCED_FACE ( 'NONE', ( #20511, #28355 ), #18463, .F. ) ;
#15788=CARTESIAN_POINT ( 'NONE',  ( 61.22499999726880304, 160.0630714827496206, -15.58253175000000823 ) ) ;
#15803=CARTESIAN_POINT ( 'NONE',  ( 37.32499999726881157, 164.1591823560292198, -12.60653300113719766 ) ) ;
#15810=CARTESIAN_POINT ( 'NONE',  ( 80.09999999453761177, 159.7113355953771077, -14.50000000000000888 ) ) ;
#15824=CARTESIAN_POINT ( 'NONE',  ( 87.50000000000001421, 166.8192717339189812, 9.236060614774261879 ) ) ;
#15825=CARTESIAN_POINT ( 'NONE',  ( 56.18867513459483121, 140.7341522555726669, 4.635254915624211769 ) ) ;
#15828=CARTESIAN_POINT ( 'NONE',  ( 82.21132485994283456, 170.7719333635740497, -7.904646289410545231E-15 ) ) ;
#15830=CARTESIAN_POINT ( 'NONE',  ( 64.77499999726882152, 140.1801316387863778, 4.815267126137185549 ) ) ;
#15834=CARTESIAN_POINT ( 'NONE',  ( 43.78867513459481842, 155.0000000000000000, 15.00000000000001243 ) ) ;
#15837=CARTESIAN_POINT ( 'NONE',  ( 125.5000000000000000, 81.56696077377658582, -76.47359838532473475 ) ) ;
#15843=CARTESIAN_POINT ( 'NONE',  ( 37.22499999726881015, 160.0630714827496206, -15.58253175000000823 ) ) ;
#15848=CARTESIAN_POINT ( 'NONE',  ( 60.47499999726881725, 149.9369285172503510, 15.58253174999999580 ) ) ;
#15851=CARTESIAN_POINT ( 'NONE',  ( 35.11132485994280472, 140.7341522555726669, 4.635254915624211769 ) ) ;
#15853=CARTESIAN_POINT ( 'NONE',  ( 50.78867513459482552, 155.0000000000000000, -15.00000000000002487 ) ) ;
#15854=CARTESIAN_POINT ( 'NONE',  ( 61.99999999453763166, 155.0000000000000000, -14.50000000000000711 ) ) ;
#15857=CARTESIAN_POINT ( 'NONE',  ( 77.11132485994281183, 140.7341522555726669, 4.635254915624211769 ) ) ;
#15861=CARTESIAN_POINT ( 'NONE',  ( 71.08867513459483689, 167.7597621252805880, -9.270509831248443078 ) ) ;
#15869=( BOUNDED_CURVE ( )  B_SPLINE_CURVE ( 2, ( #29142, #3079, #26576, #859, #3406, #13467, #5961, #26744, #23860, #18427, #28977 ),
 .UNSPECIFIED., .F., .T. ) 
 B_SPLINE_CURVE_WITH_KNOTS ( ( 3, 2, 2, 2, 2, 3 ),
 ( 0.6785714285714284921, 0.6821428571428570509, 0.6857142857142856096, 0.6892857142857142794, 0.6928571428571428381, 0.6964285714285713969 ),
 .UNSPECIFIED. ) 
 CURVE ( )  GEOMETRIC_REPRESENTATION_ITEM ( )  RATIONAL_B_SPLINE_CURVE ( ( 1.000000000000001554, 0.9510565162951518658, 1.000000000000000000, 0.9510565162951534202, 1.000000000000000000, 0.9510565162951534202, 1.000000000000000000, 0.9510565162951534202, 1.000000000000000000, 0.9510565162951534202, 1.000000000000000000 ) ) 
 REPRESENTATION_ITEM ( '' )  );
#15871=CARTESIAN_POINT ( 'NONE',  ( 41.27499999726880731, 149.9369285172503510, -15.58253175000000823 ) ) ;
#15872=ORIENTED_EDGE ( 'NONE', *, *, #11608, .F. ) ;
#15873=CARTESIAN_POINT ( 'NONE',  ( 53.82499999726881157, 168.2552932293087906, 9.630534252274372875 ) ) ;
#15876=AXIS2_PLACEMENT_3D ( 'NONE', #22414, #27196, #1309 ) ;
#15878=CARTESIAN_POINT ( 'NONE',  ( 53.27499999726880731, 149.9369285172503510, -15.58253175000000823 ) ) ;
#15879=CARTESIAN_POINT ( 'NONE',  ( 32.50000000000000000, 155.0000000000000000, 15.00000000000001243 ) ) ;
#15882=CARTESIAN_POINT ( 'NONE',  ( 64.70000000000000284, 163.5228861582408797, -11.73074641843674470 ) ) ;
#15887=CARTESIAN_POINT ( 'NONE',  ( 39.87499999726880162, 171.3844434931184253, -7.942151717890132712E-15 ) ) ;
#15889=CARTESIAN_POINT ( 'NONE',  ( 68.12499999726881583, 155.0000000000000000, 15.58253174999999402 ) ) ;
#15892=CARTESIAN_POINT ( 'NONE',  ( 39.79999999453762882, 146.4771138417591203, -11.73074641843674470 ) ) ;
#15895=VERTEX_POINT ( 'NONE', #10959 ) ;
#15908=CARTESIAN_POINT ( 'NONE',  ( 56.31132485994280756, 169.2658477444273331, 4.635254915624208216 ) ) ;
#15910=CARTESIAN_POINT ( 'NONE',  ( 33.22499999726881725, 160.0630714827496206, -15.58253175000000823 ) ) ;
#15912=CARTESIAN_POINT ( 'NONE',  ( 35.37499999726881583, 155.0000000000000000, -15.58253175000000823 ) ) ;
#15917=CARTESIAN_POINT ( 'NONE',  ( 45.60000000000000142, 150.2886644046228639, 14.49999999999999645 ) ) ;
#15919=DIRECTION ( 'NONE',  ( -1.000000000000000000, 0.000000000000000000, -0.000000000000000000 ) ) ;
#15921=CARTESIAN_POINT ( 'NONE',  ( 48.92499999726881299, 145.8408176439707802, -12.60653300113719588 ) ) ;
#15925=CARTESIAN_POINT ( 'NONE',  ( 61.62499999726880162, 171.3844434931184253, -7.942151717890134290E-15 ) ) ;
#15926=CARTESIAN_POINT ( 'NONE',  ( 76.67499999726881299, 141.7447067706911810, 9.630534252274376428 ) ) ;
#15928=CARTESIAN_POINT ( 'NONE',  ( 49.01132485994281041, 142.2402378747194405, 9.270509831248432420 ) ) ;
#15950=CARTESIAN_POINT ( 'NONE',  ( 74.62499999726881583, 138.6155565068815747, -3.929120461958505118E-15 ) ) ;
#15952=CARTESIAN_POINT ( 'NONE',  ( 32.50000000000000000, 155.0000000000000000, -6.938893903907228378E-15 ) ) ;
#15953=CARTESIAN_POINT ( 'NONE',  ( 73.02499999726882152, 149.9369285172503510, -15.58253175000000823 ) ) ;
#15971=CARTESIAN_POINT ( 'NONE',  ( 43.02499999726880020, 149.9369285172503510, -15.58253175000000823 ) ) ;
#15980=CARTESIAN_POINT ( 'NONE',  ( 82.69999999453762030, 167.3344367211045096, 8.961492836873468093 ) ) ;
#15983=EDGE_CURVE ( 'NONE', #14298, #14095, #23926, .T. ) ;
#15991=CARTESIAN_POINT ( 'NONE',  ( 79.97499999726881015, 169.8198683612136222, 4.815267126137181997 ) ) ;
#15993=CARTESIAN_POINT ( 'NONE',  ( 59.38867513459481984, 169.2658477444273331, 4.635254915624208216 ) ) ;
#15997=CARTESIAN_POINT ( 'NONE',  ( 65.57499999726881867, 164.1591823560292198, -12.60653300113719766 ) ) ;
#15999=CARTESIAN_POINT ( 'NONE',  ( 41.58867513459482979, 163.8167787843871110, 12.13525491562421621 ) ) ;
#16007=CARTESIAN_POINT ( 'NONE',  ( 82.67499999726879878, 141.7447067706911810, 9.630534252274376428 ) ) ;
#16009=CARTESIAN_POINT ( 'NONE',  ( 41.02499999726880731, 149.9369285172503510, -15.58253175000000823 ) ) ;
#16014=CARTESIAN_POINT ( 'NONE',  ( 55.27499999726881441, 149.9369285172503510, -15.58253175000000823 ) ) ;
#16022=CARTESIAN_POINT ( 'NONE',  ( 60.69999999453763451, 167.3344367211045096, 8.961492836873468093 ) ) ;
#16026=CARTESIAN_POINT ( 'NONE',  ( 125.5000000000000000, 229.9533188057739039, -74.95331880577418815 ) ) ;
#16031=ORIENTED_EDGE ( 'NONE', *, *, #6663, .F. ) ;
#16032=CARTESIAN_POINT ( 'NONE',  ( 87.50000000000002842, 169.3860439379083402, -5.988074444788474615 ) ) ;
#16037=CARTESIAN_POINT ( 'NONE',  ( 46.37499999726880873, 155.0000000000000000, 15.58253174999999402 ) ) ;
#16039=CARTESIAN_POINT ( 'NONE',  ( 49.12499999726880873, 155.0000000000000000, -15.58253175000000823 ) ) ;
#16043=CARTESIAN_POINT ( 'NONE',  ( 53.47499999726881015, 160.0630714827496206, -15.58253175000000823 ) ) ;
#16048=CARTESIAN_POINT ( 'NONE',  ( 76.70000000000000284, 163.5228861582408797, -11.73074641843674470 ) ) ;
#16054=CARTESIAN_POINT ( 'NONE',  ( 36.57499999726881157, 145.8408176439707802, 12.60653300113718345 ) ) ;
#16057=CARTESIAN_POINT ( 'NONE',  ( 79.62499999726881583, 171.3844434931184253, -7.942151717890132712E-15 ) ) ;
#16060=CARTESIAN_POINT ( 'NONE',  ( 41.79999999453762882, 146.4771138417591203, -11.73074641843674470 ) ) ;
#16075=CARTESIAN_POINT ( 'NONE',  ( 56.41132485994282320, 167.7597621252805880, 9.270509831248428867 ) ) ;
#16078=CARTESIAN_POINT ( 'NONE',  ( 34.17499999726881299, 164.1591823560292198, 12.60653300113718167 ) ) ;
#16082=CARTESIAN_POINT ( 'NONE',  ( 57.50000000000000000, 155.0000000000000000, 14.49999999999999467 ) ) ;
#16084=CARTESIAN_POINT ( 'NONE',  ( 32.50000000000000000, 155.0000000000000000, -15.00000000000002487 ) ) ;
#16085=CARTESIAN_POINT ( 'NONE',  ( 51.52499999726881441, 169.8198683612136222, -4.815267126137197984 ) ) ;
#16087=CARTESIAN_POINT ( 'NONE',  ( 89.50000000000001421, 155.0000000000000000, 70.00000000000000000 ) ) ;
#16088=CARTESIAN_POINT ( 'NONE',  ( 63.82499999726881867, 168.2552932293087906, 9.630534252274372875 ) ) ;
#16089=CARTESIAN_POINT ( 'NONE',  ( 77.77499999726880731, 169.8198683612136222, -4.815267126137197984 ) ) ;
#16093=CARTESIAN_POINT ( 'NONE',  ( 84.38867513459483405, 140.7341522555726669, -4.635254915624220651 ) ) ;
#16094=ORIENTED_EDGE ( 'NONE', *, *, #3345, .F. ) ;
#16104=VERTEX_POINT ( 'NONE', #30191 ) ;
#16108=CARTESIAN_POINT ( 'NONE',  ( 80.72499999726881015, 140.1801316387863778, -4.815267126137194431 ) ) ;
#16112=CARTESIAN_POINT ( 'NONE',  ( 66.82499999726881867, 141.7447067706911810, -9.630534252274385310 ) ) ;
#16123=CIRCLE ( 'NONE', #5790, 2.149999999999984812 ) ;
#16128=CARTESIAN_POINT ( 'NONE',  ( 44.12499999726881583, 155.0000000000000000, 15.58253174999999402 ) ) ;
#16132=EDGE_CURVE ( 'NONE', #28748, #13563, #27398, .T. ) ;
#16136=CARTESIAN_POINT ( 'NONE',  ( 79.59999999453762598, 141.2096805137202580, -4.480746418436742040 ) ) ;
#16140=AXIS2_PLACEMENT_3D ( 'NONE', #29605, #14092, #11710 ) ;
#16146=ORIENTED_EDGE ( 'NONE', *, *, #13907, .T. ) ;
#16148=CARTESIAN_POINT ( 'NONE',  ( 75.87499999726881583, 171.3844434931184253, -7.942151717890134290E-15 ) ) ;
#16150=DIRECTION ( 'NONE',  ( 1.000000000000000000, 0.000000000000000000, 0.000000000000000000 ) ) ;
#16154=CARTESIAN_POINT ( 'NONE',  ( 62.57499999726881867, 145.8408176439707802, 12.60653300113718345 ) ) ;
#16161=CARTESIAN_POINT ( 'NONE',  ( 82.88867513459484826, 159.8737954434937194, -14.99999999999995559 ) ) ;
#16163=CARTESIAN_POINT ( 'NONE',  ( 85.37499999726881583, 155.0000000000000000, -15.58253175000000823 ) ) ;
#16168=CARTESIAN_POINT ( 'NONE',  ( 37.82499999726881157, 168.2552932293087906, 9.630534252274372875 ) ) ;
#16172=CARTESIAN_POINT ( 'NONE',  ( 54.87499999726880162, 138.6155565068815463, -3.929120461958505118E-15 ) ) ;
#16178=CARTESIAN_POINT ( 'NONE',  ( 54.88867513459484115, 159.8737954434938615, -14.99999999999984190 ) ) ;
#16180=CARTESIAN_POINT ( 'NONE',  ( 58.99999999453763166, 155.0000000000000000, 14.49999999999999467 ) ) ;
#16183=CARTESIAN_POINT ( 'NONE',  ( 77.51132485994280330, 146.1832212156128890, -12.13525491562423042 ) ) ;
#16185=CARTESIAN_POINT ( 'NONE',  ( 59.71132485994280614, 155.0000000000000000, -15.00000000000002487 ) ) ;
#16192=DIRECTION ( 'NONE',  ( 0.000000000000000000, 0.7071067811865475727, 0.7071067811865475727 ) ) ;
#16193=CARTESIAN_POINT ( 'NONE',  ( 87.50000000000002842, 169.3860439379083402, -5.988074444788474615 ) ) ;
#16199=CARTESIAN_POINT ( 'NONE',  ( 46.97499999726881015, 140.1801316387863778, -4.815267126137194431 ) ) ;
#16200=AXIS2_PLACEMENT_3D ( 'NONE', #27451, #17737, #9557 ) ;
#16202=CARTESIAN_POINT ( 'NONE',  ( 50.82499999726880446, 141.7447067706911810, -9.630534252274385310 ) ) ;
#16203=LINE ( 'NONE', #31712, #6105 ) ;
#16208=CARTESIAN_POINT ( 'NONE',  ( 52.97499999726881015, 140.1801316387863778, -4.815267126137194431 ) ) ;
#16210=CARTESIAN_POINT ( 'NONE',  ( 73.08867513459483689, 167.7597621252805880, -9.270509831248443078 ) ) ;
#16212=CARTESIAN_POINT ( 'NONE',  ( 70.70000000000001705, 163.5228861582408797, -11.73074641843674470 ) ) ;
#16213=CARTESIAN_POINT ( 'NONE',  ( 127.5000000000000000, 228.4330392262228600, -76.47359838532526055 ) ) ;
#16217=CARTESIAN_POINT ( 'NONE',  ( 37.47499999726880304, 160.0630714827496206, -15.58253175000000823 ) ) ;
#16220=CARTESIAN_POINT ( 'NONE',  ( 79.42499999726881299, 168.2552932293087906, -9.630534252274385310 ) ) ;
#16223=CARTESIAN_POINT ( 'NONE',  ( 48.51132485994280330, 163.8167787843871110, 12.13525491562421621 ) ) ;
#16224=CARTESIAN_POINT ( 'NONE',  ( 38.59999999453762598, 168.7903194862797420, 4.480746418436729606 ) ) ;
#16227=VECTOR ( 'NONE', #26367, 1000.000000000000000 ) ;
#16234=ORIENTED_EDGE ( 'NONE', *, *, #23067, .T. ) ;
#16236=EDGE_CURVE ( 'NONE', #17237, #7737, #14351, .T. ) ;
#16239=ORIENTED_EDGE ( 'NONE', *, *, #5564, .F. ) ;
#16242=ADVANCED_FACE ( 'NONE', ( #14350 ), #16896, .T. ) ;
#16244=AXIS2_PLACEMENT_3D ( 'NONE', #10856, #23626, #13565 ) ;
#16246=CARTESIAN_POINT ( 'NONE',  ( 55.71132485994280614, 155.0000000000000000, -15.00000000000002487 ) ) ;
#16250=CARTESIAN_POINT ( 'NONE',  ( 35.47499999726880304, 160.0630714827496206, -15.58253175000000823 ) ) ;
#16254=CARTESIAN_POINT ( 'NONE',  ( 52.70000000000000284, 163.5228861582408797, -11.73074641843674470 ) ) ;
#16257=CARTESIAN_POINT ( 'NONE',  ( 58.12499999726881583, 155.0000000000000000, 15.58253174999999402 ) ) ;
#16260=CARTESIAN_POINT ( 'NONE',  ( 64.12499999726881583, 155.0000000000000000, 15.58253174999999402 ) ) ;
#16261=CARTESIAN_POINT ( 'NONE',  ( 75.17499999726881299, 145.8408176439707802, -12.60653300113719588 ) ) ;
#16276=VERTEX_POINT ( 'NONE', #30359 ) ;
#16282=CARTESIAN_POINT ( 'NONE',  ( 76.42499999726879878, 141.7447067706911810, 9.630534252274376428 ) ) ;
#16286=CARTESIAN_POINT ( 'NONE',  ( 69.32499999726881867, 164.1591823560292198, -12.60653300113719766 ) ) ;
#16290=CARTESIAN_POINT ( 'NONE',  ( 36.70000000000000284, 163.5228861582408797, -11.73074641843674470 ) ) ;
#16298=CARTESIAN_POINT ( 'NONE',  ( 46.92499999726881299, 145.8408176439707802, -12.60653300113719588 ) ) ;
#16307=CARTESIAN_POINT ( 'NONE',  ( 79.69999999453764872, 142.6655632788954620, -8.961492836873480528 ) ) ;
#16317=CARTESIAN_POINT ( 'NONE',  ( 75.27499999726880731, 149.9369285172503510, -15.58253175000000823 ) ) ;
#16318=CARTESIAN_POINT ( 'NONE',  ( 53.71132485994279904, 155.0000000000000000, -15.00000000000002487 ) ) ;
#16323=CARTESIAN_POINT ( 'NONE',  ( 70.47499999726881015, 149.9369285172503510, 15.58253174999999580 ) ) ;
#16324=ORIENTED_EDGE ( 'NONE', *, *, #30352, .F. ) ;
#16329=CARTESIAN_POINT ( 'NONE',  ( 80.61132485994284025, 159.8737954434934920, 15.00000000000010836 ) ) ;
#16331=CARTESIAN_POINT ( 'NONE',  ( 83.07499999726880446, 141.7447067706911810, -9.630534252274385310 ) ) ;
#16334=CARTESIAN_POINT ( 'NONE',  ( 37.42499999726881299, 168.2552932293087906, -9.630534252274385310 ) ) ;
#16335=CARTESIAN_POINT ( 'NONE',  ( 36.28867513459483263, 139.2280666364260071, -4.041636747397287284E-15 ) ) ;
#16339=CARTESIAN_POINT ( 'NONE',  ( 59.87499999726882294, 171.3844434931184253, -7.942151717890132712E-15 ) ) ;
#16345=CARTESIAN_POINT ( 'NONE',  ( 57.69999999453762740, 142.6655632788954620, -8.961492836873480528 ) ) ;
#16353=ORIENTED_EDGE ( 'NONE', *, *, #20444, .T. ) ;
#16361=CARTESIAN_POINT ( 'NONE',  ( 50.57499999726881157, 145.8408176439707802, 12.60653300113718345 ) ) ;
#16363=CARTESIAN_POINT ( 'NONE',  ( 57.22499999726879594, 160.0630714827496206, -15.58253175000000823 ) ) ;
#16365=AXIS2_PLACEMENT_3D ( 'NONE', #33528, #22965, #33363 ) ;
#16367=EDGE_CURVE ( 'NONE', #20973, #4513, #5429, .T. ) ;
#16369=CARTESIAN_POINT ( 'NONE',  ( 55.77499999726881441, 169.8198683612136222, -4.815267126137197984 ) ) ;
#16374=CARTESIAN_POINT ( 'NONE',  ( 70.80000000000001137, 167.3344367211045096, -8.961492836873482304 ) ) ;
#16375=CARTESIAN_POINT ( 'NONE',  ( 40.48867513459481415, 142.2402378747194405, -9.270509831248439525 ) ) ;
#16379=CARTESIAN_POINT ( 'NONE',  ( 39.27499999726880020, 149.9369285172503510, -15.58253175000000823 ) ) ;
#16381=CARTESIAN_POINT ( 'NONE',  ( 77.42499999726882720, 168.2552932293087906, -9.630534252274385310 ) ) ;
#16384=CARTESIAN_POINT ( 'NONE',  ( 43.89999999453761603, 150.2886644046228639, -14.50000000000000888 ) ) ;
#16386=EDGE_CURVE ( 'NONE', #7333, #23334, #20650, .T. ) ;
#16398=CARTESIAN_POINT ( 'NONE',  ( 50.28867513459483263, 139.2280666364260071, -4.041636747397287284E-15 ) ) ;
#16404=ORIENTED_EDGE ( 'NONE', *, *, #11642, .T. ) ;
#16405=CARTESIAN_POINT ( 'NONE',  ( 39.02499999726880731, 149.9369285172503510, -15.58253175000000823 ) ) ;
#16406=( BOUNDED_CURVE ( )  B_SPLINE_CURVE ( 2, ( #29083, #14202, #7978, #5731, #1260, #16756, #11485, #18362, #11655, #11817, #13242 ),
 .UNSPECIFIED., .F., .T. ) 
 B_SPLINE_CURVE_WITH_KNOTS ( ( 3, 2, 2, 2, 2, 3 ),
 ( 0.4285714285714284366, 0.4321428571428569954, 0.4357142857142856651, 0.4392857142857141683, 0.4428571428571427271, 0.4464285714285712858 ),
 .UNSPECIFIED. ) 
 CURVE ( )  GEOMETRIC_REPRESENTATION_ITEM ( )  RATIONAL_B_SPLINE_CURVE ( ( 1.000000000000000666, 0.9510565162951526430, 1.000000000000000000, 0.9510565162951534202, 1.000000000000000000, 0.9510565162951534202, 1.000000000000000000, 0.9510565162951534202, 1.000000000000000000, 0.9510565162951549745, 0.9999999999999984457 ) ) 
 REPRESENTATION_ITEM ( '' )  );
#16408=CARTESIAN_POINT ( 'NONE',  ( 88.12499999726880162, 155.0000000000000000, 15.58253174999999402 ) ) ;
#16412=CARTESIAN_POINT ( 'NONE',  ( 54.39999999999999147, 150.2886644046228639, -14.50000000000000888 ) ) ;
#16414=DIRECTION ( 'NONE',  ( 0.000000000000000000, 0.000000000000000000, -1.000000000000000000 ) ) ;
#16416=CARTESIAN_POINT ( 'NONE',  ( 60.92499999726882010, 145.8408176439707802, -12.60653300113719588 ) ) ;
#16418=FACE_OUTER_BOUND ( 'NONE', #5532, .T. ) ;
#16420=CARTESIAN_POINT ( 'NONE',  ( 60.82499999726881157, 141.7447067706911810, -9.630534252274387086 ) ) ;
#16421=CARTESIAN_POINT ( 'NONE',  ( 73.87499999726881583, 171.3844434931184253, -7.942151717890132712E-15 ) ) ;
#16423=EDGE_CURVE ( 'NONE', #29398, #6338, #32291, .T. ) ;
#16425=CARTESIAN_POINT ( 'NONE',  ( 84.58867513459483689, 146.1832212156128890, -12.13525491562423042 ) ) ;
#16435=ORIENTED_EDGE ( 'NONE', *, *, #25101, .T. ) ;
#16442=CARTESIAN_POINT ( 'NONE',  ( 75.62499999726881583, 171.3844434931184253, -7.942151717890134290E-15 ) ) ;
#16447=CARTESIAN_POINT ( 'NONE',  ( 69.92499999726881299, 164.1591823560292198, 12.60653300113718167 ) ) ;
#16451=CARTESIAN_POINT ( 'NONE',  ( 38.19999999999998153, 142.6655632788954620, -8.961492836873480528 ) ) ;
#16461=CARTESIAN_POINT ( 'NONE',  ( 42.92499999726881299, 145.8408176439707802, -12.60653300113719588 ) ) ;
#16469=CARTESIAN_POINT ( 'NONE',  ( 82.89999999453760893, 159.7113355953771077, 14.49999999999999289 ) ) ;
#16470=AXIS2_PLACEMENT_3D ( 'NONE', #7230, #32772, #11832 ) ;
#16475=AXIS2_PLACEMENT_3D ( 'NONE', #15952, #11643, #1580 ) ;
#16481=ORIENTED_EDGE ( 'NONE', *, *, #24941, .F. ) ;
#16482=CARTESIAN_POINT ( 'NONE',  ( 78.67499999726879878, 141.7447067706911810, 9.630534252274376428 ) ) ;
#16484=AXIS2_PLACEMENT_3D ( 'NONE', #17132, #28203, #15751 ) ;
#16489=CARTESIAN_POINT ( 'NONE',  ( 66.37499999726881583, 155.0000000000000000, 15.58253174999999402 ) ) ;
#16490=EDGE_LOOP ( 'NONE', ( #25295, #16703 ) ) ;
#16491=CARTESIAN_POINT ( 'NONE',  ( 61.88867513459483405, 150.1262045565064227, 15.00000000000001599 ) ) ;
#16497=CARTESIAN_POINT ( 'NONE',  ( 80.31132485994280046, 169.2658477444273331, 4.635254915624208216 ) ) ;
#16499=CARTESIAN_POINT ( 'NONE',  ( 83.77499999726880731, 169.8198683612136222, -4.815267126137197984 ) ) ;
#16500=AXIS2_PLACEMENT_3D ( 'NONE', #6847, #19800, #11961 ) ;
#16503=CARTESIAN_POINT ( 'NONE',  ( 35.42499999726880588, 168.2552932293087906, -9.630534252274385310 ) ) ;
#16505=CARTESIAN_POINT ( 'NONE',  ( 37.78867513459481842, 155.0000000000000000, 15.00000000000001243 ) ) ;
#16508=CARTESIAN_POINT ( 'NONE',  ( 62.47499999726881725, 149.9369285172503510, 15.58253174999999580 ) ) ;
#16515=CARTESIAN_POINT ( 'NONE',  ( 64.29999999453762882, 167.3344367211045096, -8.961492836873482304 ) ) ;
#16526=PLANE ( 'NONE',  #6424 ) ;
#16527=CARTESIAN_POINT ( 'NONE',  ( 32.50000000000000000, 155.0000000000000000, -15.00000000000002487 ) ) ;
#16533=CARTESIAN_POINT ( 'NONE',  ( 48.07499999726881867, 168.2552932293087906, 9.630534252274372875 ) ) ;
#16534=EDGE_LOOP ( 'NONE', ( #16831, #216, #3837, #1294 ) ) ;
#16535=CARTESIAN_POINT ( 'NONE',  ( 57.02499999726882152, 149.9369285172503510, -15.58253175000000823 ) ) ;
#16539=DIRECTION ( 'NONE',  ( 1.000000000000000000, 0.000000000000000000, 0.000000000000000000 ) ) ;
#16541=CARTESIAN_POINT ( 'NONE',  ( 62.87499999726881583, 138.6155565068815463, -3.929120461958505118E-15 ) ) ;
#16546=CARTESIAN_POINT ( 'NONE',  ( 71.90000000000000568, 141.2096805137202580, 4.480746418436733158 ) ) ;
#16547=CARTESIAN_POINT ( 'NONE',  ( 61.71132485994280614, 155.0000000000000000, -15.00000000000002487 ) ) ;
#16550=CARTESIAN_POINT ( 'NONE',  ( 32.98867513459481415, 163.8167787843871110, -12.13525491562423397 ) ) ;
#16552=CARTESIAN_POINT ( 'NONE',  ( 44.07499999726881157, 168.2552932293087906, 9.630534252274372875 ) ) ;
#16554=CARTESIAN_POINT ( 'NONE',  ( 73.92499999726881299, 164.1591823560292198, 12.60653300113718167 ) ) ;
#16557=CARTESIAN_POINT ( 'NONE',  ( 42.79999999453762882, 163.5228861582408797, 11.73074641843673049 ) ) ;
#16559=CARTESIAN_POINT ( 'NONE',  ( 40.21132485994280614, 170.7719333635740497, -7.904646289410545231E-15 ) ) ;
#16560=ADVANCED_FACE ( 'NONE', ( #15020 ), #31206, .F. ) ;
#16565=EDGE_CURVE ( 'NONE', #8868, #3834, #27407, .T. ) ;
#16571=CARTESIAN_POINT ( 'NONE',  ( 51.31132485994280046, 140.7341522555726669, -4.635254915624220651 ) ) ;
#16572=ORIENTED_EDGE ( 'NONE', *, *, #20497, .T. ) ;
#16575=CARTESIAN_POINT ( 'NONE',  ( 33.97499999726881725, 169.8198683612136222, 4.815267126137181997 ) ) ;
#16577=CARTESIAN_POINT ( 'NONE',  ( 39.52499999726881441, 169.8198683612136222, -4.815267126137197984 ) ) ;
#16579=CARTESIAN_POINT ( 'NONE',  ( 41.37499999726880873, 155.0000000000000000, -15.58253175000000823 ) ) ;
#16582=APPLICATION_CONTEXT ( 'automotive_design' ) ;
#16583=CARTESIAN_POINT ( 'NONE',  ( 56.80000000000000426, 167.3344367211045096, -8.961492836873482304 ) ) ;
#16586=CARTESIAN_POINT ( 'NONE',  ( 57.12499999726880873, 155.0000000000000000, -15.58253175000000823 ) ) ;
#16589=CARTESIAN_POINT ( 'NONE',  ( 37.41132485994281609, 142.2402378747194405, -9.270509831248439525 ) ) ;
#16590=CARTESIAN_POINT ( 'NONE',  ( 67.42499999726879878, 168.2552932293087906, -9.630534252274387086 ) ) ;
#16591=CARTESIAN_POINT ( 'NONE',  ( 77.47499999726878173, 160.0630714827496206, -15.58253175000000823 ) ) ;
#16594=EDGE_CURVE ( 'NONE', #5188, #22989, #19346, .T. ) ;
#16608=CARTESIAN_POINT ( 'NONE',  ( 72.78867513459482552, 155.0000000000000000, -15.00000000000002487 ) ) ;
#16609=( BOUNDED_CURVE ( )  B_SPLINE_CURVE ( 2, ( #20996, #15383, #5325, #2944, #5658, #23555, #13327, #26116, #23719, #31393, #5160 ),
 .UNSPECIFIED., .F., .T. ) 
 B_SPLINE_CURVE_WITH_KNOTS ( ( 3, 2, 2, 2, 2, 3 ),
 ( 0.7678571428571426827, 0.7714285714285712414, 0.7749999999999998002, 0.7785714285714284699, 0.7821428571428570287, 0.7857142857142856984 ),
 .UNSPECIFIED. ) 
 CURVE ( )  GEOMETRIC_REPRESENTATION_ITEM ( )  RATIONAL_B_SPLINE_CURVE ( ( 1.000000000000001554, 0.9510565162951518658, 1.000000000000000000, 0.9510565162951534202, 1.000000000000000000, 0.9510565162951534202, 1.000000000000000000, 0.9510565162951534202, 1.000000000000000000, 0.9510565162951534202, 1.000000000000000000 ) ) 
 REPRESENTATION_ITEM ( '' )  );
#16612=CARTESIAN_POINT ( 'NONE',  ( 81.62499999726880162, 171.3844434931184253, -7.942151717890134290E-15 ) ) ;
#16615=CARTESIAN_POINT ( 'NONE',  ( 67.02499999726882152, 149.9369285172503510, -15.58253175000000823 ) ) ;
#16621=CARTESIAN_POINT ( 'NONE',  ( 32.89999999999999858, 168.7903194862797420, -4.480746418436745593 ) ) ;
#16623=ADVANCED_FACE ( 'NONE', ( #28974 ), #8204, .T. ) ;
#16630=CARTESIAN_POINT ( 'NONE',  ( 43.92499999726881299, 164.1591823560292198, 12.60653300113718167 ) ) ;
#16637=CARTESIAN_POINT ( 'NONE',  ( 87.09999999453764019, 150.2886644046228639, 14.49999999999999645 ) ) ;
#16644=CARTESIAN_POINT ( 'NONE',  ( 73.27499999726882152, 149.9369285172503510, -15.58253175000000823 ) ) ;
#16650=CARTESIAN_POINT ( 'NONE',  ( 81.37499999726881583, 155.0000000000000000, -15.58253175000000823 ) ) ;
#16655=EDGE_CURVE ( 'NONE', #25537, #2009, #10020, .T. ) ;
#16658=CARTESIAN_POINT ( 'NONE',  ( 66.47499999726881015, 149.9369285172503510, 15.58253174999999580 ) ) ;
#16665=EDGE_CURVE ( 'NONE', #30462, #6526, #10011, .T. ) ;
#16668=CARTESIAN_POINT ( 'NONE',  ( 86.07499999726880446, 168.2552932293087906, 9.630534252274372875 ) ) ;
#16671=CARTESIAN_POINT ( 'NONE',  ( 47.62499999726880162, 171.3844434931184253, -7.942151717890132712E-15 ) ) ;
#16680=CARTESIAN_POINT ( 'NONE',  ( 85.68867513459483121, 159.8737954434936341, 14.99999999999997158 ) ) ;
#16683=CARTESIAN_POINT ( 'NONE',  ( 67.49999999453763166, 139.7537977485451393, -4.138211985947621020E-15 ) ) ;
#16687=CARTESIAN_POINT ( 'NONE',  ( 32.50000000000000000, 155.0000000000000000, 15.00000000000001243 ) ) ;
#16702=CARTESIAN_POINT ( 'NONE',  ( 51.97499999726881725, 169.8198683612136222, 4.815267126137181997 ) ) ;
#16703=ORIENTED_EDGE ( 'NONE', *, *, #28307, .F. ) ;
#16704=CARTESIAN_POINT ( 'NONE',  ( 54.32499999726880446, 145.8408176439707802, 12.60653300113718345 ) ) ;
#16709=CARTESIAN_POINT ( 'NONE',  ( 58.17499999726881299, 164.1591823560292198, 12.60653300113718167 ) ) ;
#16714=CARTESIAN_POINT ( 'NONE',  ( 72.70000000000000284, 163.5228861582408797, -11.73074641843674470 ) ) ;
#16715=CARTESIAN_POINT ( 'NONE',  ( 65.68867513459483121, 159.8737954434934920, 15.00000000000010836 ) ) ;
#16719=CARTESIAN_POINT ( 'NONE',  ( 44.77499999726881441, 140.1801316387863778, 4.815267126137185549 ) ) ;
#16721=CARTESIAN_POINT ( 'NONE',  ( 77.12499999726881583, 155.0000000000000000, -15.58253175000000823 ) ) ;
#16724=CARTESIAN_POINT ( 'NONE',  ( 46.49999999453762456, 170.2462022514548323, -7.872454543227099337E-15 ) ) ;
#16737=VECTOR ( 'NONE', #20121, 1000.000000000000000 ) ;
#16745=CARTESIAN_POINT ( 'NONE',  ( 37.72499999726881015, 169.8198683612136222, 4.815267126137181997 ) ) ;
#16748=CARTESIAN_POINT ( 'NONE',  ( 41.57499999726881157, 164.1591823560292198, -12.60653300113719766 ) ) ;
#16753=AXIS2_PLACEMENT_3D ( 'NONE', #29989, #30157, #14473 ) ;
#16755=CARTESIAN_POINT ( 'NONE',  ( 55.50000000000000000, 155.0000000000000000, 14.49999999999999467 ) ) ;
#16756=CARTESIAN_POINT ( 'NONE',  ( 63.28867513459482552, 170.7719333635740497, -7.904646289410545231E-15 ) ) ;
#16758=CARTESIAN_POINT ( 'NONE',  ( 77.58867513459483689, 163.8167787843871110, 12.13525491562421621 ) ) ;
#16760=( BOUNDED_CURVE ( )  B_SPLINE_CURVE ( 2, ( #20977, #13305, #23697, #1031, #30316, #19755, #8853, #22136, #1362, #4246, #32193 ),
 .UNSPECIFIED., .F., .T. ) 
 B_SPLINE_CURVE_WITH_KNOTS ( ( 3, 2, 2, 2, 2, 3 ),
 ( 0.1964285714285714524, 0.2000000000000000389, 0.2035714285714285976, 0.2071428571428572118, 0.2107142857142857706, 0.2142857142857143293 ),
 .UNSPECIFIED. ) 
 CURVE ( )  GEOMETRIC_REPRESENTATION_ITEM ( )  RATIONAL_B_SPLINE_CURVE ( ( 0.9999999999999996669, 0.9510565162951537532, 1.000000000000000000, 0.9510565162951534202, 1.000000000000000000, 0.9510565162951534202, 1.000000000000000000, 0.9510565162951534202, 1.000000000000000000, 0.9510565162951526430, 1.000000000000000666 ) ) 
 REPRESENTATION_ITEM ( '' )  );
#16761=CARTESIAN_POINT ( 'NONE',  ( 58.82499999726881867, 141.7447067706911810, -9.630534252274385310 ) ) ;
#16765=CARTESIAN_POINT ( 'NONE',  ( 82.07499999726880446, 168.2552932293087906, 9.630534252274372875 ) ) ;
#16778=ORIENTED_EDGE ( 'NONE', *, *, #6413, .F. ) ;
#16781=CARTESIAN_POINT ( 'NONE',  ( 32.50000000000000000, 155.0000000000000000, -15.00000000000002487 ) ) ;
#16784=CARTESIAN_POINT ( 'NONE',  ( 83.12499999726881583, 155.0000000000000000, -15.58253175000000823 ) ) ;
#16786=CARTESIAN_POINT ( 'NONE',  ( 76.42499999726879878, 141.7447067706911810, 9.630534252274376428 ) ) ;
#16788=CARTESIAN_POINT ( 'NONE',  ( 75.78867513459483973, 155.0000000000000000, 15.00000000000001243 ) ) ;
#16790=CARTESIAN_POINT ( 'NONE',  ( 37.10000000000000142, 168.7903194862797420, 4.480746418436729606 ) ) ;
#16800=CARTESIAN_POINT ( 'NONE',  ( 51.22499999726881725, 160.0630714827496206, -15.58253175000000823 ) ) ;
#16808=CARTESIAN_POINT ( 'NONE',  ( 83.49999999453764588, 139.7537977485451393, -4.138211985947621020E-15 ) ) ;
#16809=( BOUNDED_CURVE ( )  B_SPLINE_CURVE ( 2, ( #1765, #19999, #27824, #14886, #27162, #1269, #7399, #23231, #26126, #15228, #5171 ),
 .UNSPECIFIED., .F., .T. ) 
 B_SPLINE_CURVE_WITH_KNOTS ( ( 3, 2, 2, 2, 2, 3 ),
 ( 0.1607142857142856984, 0.1642857142857142572, 0.1678571428571428437, 0.1714285714285714302, 0.1750000000000000167, 0.1785714285714286031 ),
 .UNSPECIFIED. ) 
 CURVE ( )  GEOMETRIC_REPRESENTATION_ITEM ( )  RATIONAL_B_SPLINE_CURVE ( ( 1.000000000000000444, 0.9510565162951530871, 1.000000000000000000, 0.9510565162951534202, 1.000000000000000000, 0.9510565162951534202, 1.000000000000000000, 0.9510565162951534202, 1.000000000000000000, 0.9510565162951530871, 1.000000000000000444 ) ) 
 REPRESENTATION_ITEM ( '' )  );
#16812=ADVANCED_FACE ( 'NONE', ( #5959 ), #13800, .T. ) ;
#16818=CARTESIAN_POINT ( 'NONE',  ( 72.07499999726880446, 168.2552932293087906, 9.630534252274372875 ) ) ;
#16821=EDGE_CURVE ( 'NONE', #11212, #28445, #6123, .T. ) ;
#16823=CARTESIAN_POINT ( 'NONE',  ( 86.57499999726880446, 145.8408176439707802, 12.60653300113718345 ) ) ;
#16830=CARTESIAN_POINT ( 'NONE',  ( 69.37499999726881583, 155.0000000000000000, -15.58253175000000823 ) ) ;
#16831=ORIENTED_EDGE ( 'NONE', *, *, #18646, .T. ) ;
#16841=CARTESIAN_POINT ( 'NONE',  ( 45.12499999726880873, 155.0000000000000000, -15.58253175000000823 ) ) ;
#16850=CARTESIAN_POINT ( 'NONE',  ( 32.50000000000000000, 155.0000000000000000, -15.00000000000002487 ) ) ;
#16854=CARTESIAN_POINT ( 'NONE',  ( 69.79999999453761461, 146.4771138417591203, -11.73074641843674470 ) ) ;
#16865=CARTESIAN_POINT ( 'NONE',  ( 42.68867513459482410, 150.1262045565064227, -15.00000000000002665 ) ) ;
#16866=LINE ( 'NONE', #18764, #29060 ) ;
#16871=CARTESIAN_POINT ( 'NONE',  ( 52.67499999726880588, 141.7447067706911810, 9.630534252274376428 ) ) ;
#16877=CARTESIAN_POINT ( 'NONE',  ( 60.67499999726881299, 141.7447067706911810, 9.630534252274376428 ) ) ;
#16881=CARTESIAN_POINT ( 'NONE',  ( 83.30000000000001137, 163.5228861582408797, 11.73074641843673049 ) ) ;
#16882=CARTESIAN_POINT ( 'NONE',  ( 62.51132485994280330, 163.8167787843871110, 12.13525491562421621 ) ) ;
#16886=CARTESIAN_POINT ( 'NONE',  ( 45.57499999726881157, 164.1591823560292198, -12.60653300113719766 ) ) ;
#16889=CARTESIAN_POINT ( 'NONE',  ( 85.12499999726881583, 155.0000000000000000, -15.58253175000000823 ) ) ;
#16892=CARTESIAN_POINT ( 'NONE',  ( 49.51132485994280330, 146.1832212156128890, -12.13525491562423042 ) ) ;
#16893=CARTESIAN_POINT ( 'NONE',  ( 50.79999999453762882, 163.5228861582408797, 11.73074641843673049 ) ) ;
#16895=EDGE_CURVE ( 'NONE', #28642, #11454, #6930, .T. ) ;
#16896=CYLINDRICAL_SURFACE ( 'NONE', #16500, 15.00000000000001776 ) ;
#16897=CARTESIAN_POINT ( 'NONE',  ( 66.41132485994285162, 167.7597621252805880, 9.270509831248428867 ) ) ;
#16904=CARTESIAN_POINT ( 'NONE',  ( 78.98867513459482836, 163.8167787843871110, -12.13525491562423397 ) ) ;
#16905=VECTOR ( 'NONE', #15670, 1000.000000000000000 ) ;
#16910=CARTESIAN_POINT ( 'NONE',  ( 33.57499999726881157, 164.1591823560292198, -12.60653300113719766 ) ) ;
#16912=CARTESIAN_POINT ( 'NONE',  ( 36.52499999726881441, 140.1801316387863778, 4.815267126137185549 ) ) ;
#16915=CARTESIAN_POINT ( 'NONE',  ( 38.77499999726881441, 140.1801316387863778, 4.815267126137185549 ) ) ;
#16918=CARTESIAN_POINT ( 'NONE',  ( 63.90000000000001279, 141.2096805137202580, 4.480746418436733158 ) ) ;
#16921=CARTESIAN_POINT ( 'NONE',  ( 77.28867513459483973, 170.7719333635740497, -7.904646289410545231E-15 ) ) ;
#16925=CARTESIAN_POINT ( 'NONE',  ( 59.32499999726881157, 164.1591823560292198, -12.60653300113719766 ) ) ;
#16928=CARTESIAN_POINT ( 'NONE',  ( 125.5000000000000000, 80.04668119422552763, -74.95331880577366235 ) ) ;
#16929=AXIS2_PLACEMENT_3D ( 'NONE', #23306, #7129, #25688 ) ;
#16930=CARTESIAN_POINT ( 'NONE',  ( 84.27499999726879309, 160.0630714827496206, 15.58253174999999402 ) ) ;
#16932=CARTESIAN_POINT ( 'NONE',  ( 72.78867513459482552, 155.0000000000000000, -15.00000000000002487 ) ) ;
#16933=CARTESIAN_POINT ( 'NONE',  ( 53.18867513459482410, 169.2658477444273331, -4.635254915624224203 ) ) ;
#16942=ORIENTED_EDGE ( 'NONE', *, *, #12294, .F. ) ;
#16943=CARTESIAN_POINT ( 'NONE',  ( 38.81132485994282177, 150.1262045565064795, 15.00000000000006395 ) ) ;
#16948=CARTESIAN_POINT ( 'NONE',  ( 84.32499999726880446, 145.8408176439707802, 12.60653300113718345 ) ) ;
#16949=ORIENTED_EDGE ( 'NONE', *, *, #11483, .F. ) ;
#16950=CARTESIAN_POINT ( 'NONE',  ( 68.81132485994281467, 150.1262045565065364, 15.00000000000011191 ) ) ;
#16952=CARTESIAN_POINT ( 'NONE',  ( 74.12499999726881583, 155.0000000000000000, 15.58253174999999402 ) ) ;
#16954=( BOUNDED_CURVE ( )  B_SPLINE_CURVE ( 2, ( #5944, #842, #5618, #24342, #5773, #16335, #3731, #26729, #11568, #14120, #8191 ),
 .UNSPECIFIED., .F., .T. ) 
 B_SPLINE_CURVE_WITH_KNOTS ( ( 3, 2, 2, 2, 2, 3 ),
 ( 0.9107142857142853654, 0.9142857142857139241, 0.9178571428571425939, 0.9214285714285711526, 0.9249999999999998224, 0.9285714285714283811 ),
 .UNSPECIFIED. ) 
 CURVE ( )  GEOMETRIC_REPRESENTATION_ITEM ( )  RATIONAL_B_SPLINE_CURVE ( ( 1.000000000000004663, 0.9510565162951488682, 1.000000000000000000, 0.9510565162951534202, 1.000000000000000000, 0.9510565162951534202, 1.000000000000000000, 0.9510565162951534202, 1.000000000000000000, 0.9510565162951549745, 0.9999999999999984457 ) ) 
 REPRESENTATION_ITEM ( '' )  );
#16956=CARTESIAN_POINT ( 'NONE',  ( 87.50000000000001421, 166.8192717339189812, 9.236060614774261879 ) ) ;
#16959=CARTESIAN_POINT ( 'NONE',  ( 43.10000000000000142, 168.7903194862797420, 4.480746418436729606 ) ) ;
#16963=LINE ( 'NONE', #17138, #4279 ) ;
#16965=CARTESIAN_POINT ( 'NONE',  ( 48.52499999726880731, 140.1801316387863778, 4.815267126137185549 ) ) ;
#16972=CARTESIAN_POINT ( 'NONE',  ( 85.49999999453763166, 139.7537977485451393, -4.138211985947621020E-15 ) ) ;
#16981=CARTESIAN_POINT ( 'NONE',  ( 70.27499999726880731, 160.0630714827496206, 15.58253174999999402 ) ) ;
#16983=EDGE_CURVE ( 'NONE', #15895, #18797, #14572, .T. ) ;
#16986=CARTESIAN_POINT ( 'NONE',  ( 84.17499999726882720, 164.1591823560292198, 12.60653300113718167 ) ) ;
#16993=CARTESIAN_POINT ( 'NONE',  ( 70.17499999726881299, 164.1591823560292198, 12.60653300113718167 ) ) ;
#16996=EDGE_CURVE ( 'NONE', #17245, #28697, #9811, .T. ) ;
#17003=CARTESIAN_POINT ( 'NONE',  ( 71.01132485994281751, 142.2402378747194405, 9.270509831248432420 ) ) ;
#17008=CARTESIAN_POINT ( 'NONE',  ( 46.72499999726881015, 140.1801316387863778, -4.815267126137194431 ) ) ;
#17010=CARTESIAN_POINT ( 'NONE',  ( 33.72499999726881725, 169.8198683612136222, 4.815267126137181997 ) ) ;
#17013=EDGE_CURVE ( 'NONE', #1328, #3092, #15673, .T. ) ;
#17021=CARTESIAN_POINT ( 'NONE',  ( 65.39999999453763735, 141.2096805137202580, 4.480746418436733158 ) ) ;
#17028=ORIENTED_EDGE ( 'NONE', *, *, #26031, .T. ) ;
#17032=CARTESIAN_POINT ( 'NONE',  ( 42.58867513459482979, 146.1832212156128890, -12.13525491562423042 ) ) ;
#17034=FACE_OUTER_BOUND ( 'NONE', #11097, .T. ) ;
#17037=AXIS2_PLACEMENT_3D ( 'NONE', #19968, #7031, #25080 ) ;
#17040=CARTESIAN_POINT ( 'NONE',  ( 48.57499999726881157, 145.8408176439707802, 12.60653300113718345 ) ) ;
#17043=CARTESIAN_POINT ( 'NONE',  ( 67.11132485994281183, 140.7341522555726669, 4.635254915624211769 ) ) ;
#17047=CARTESIAN_POINT ( 'NONE',  ( 57.47499999726879594, 160.0630714827496206, -15.58253175000000823 ) ) ;
#17049=DIRECTION ( 'NONE',  ( 1.000000000000000000, 0.000000000000000000, 0.000000000000000000 ) ) ;
#17054=CARTESIAN_POINT ( 'NONE',  ( 79.30000000000001137, 163.5228861582408797, 11.73074641843673049 ) ) ;
#17059=CARTESIAN_POINT ( 'NONE',  ( 46.17499999726881299, 164.1591823560292198, 12.60653300113718167 ) ) ;
#17060=EDGE_CURVE ( 'NONE', #31940, #11543, #6523, .T. ) ;
#17062=CARTESIAN_POINT ( 'NONE',  ( 85.82499999726879025, 168.2552932293087906, 9.630534252274372875 ) ) ;
#17064=CARTESIAN_POINT ( 'NONE',  ( 35.78867513459482552, 155.0000000000000000, 15.00000000000001243 ) ) ;
#17066=CARTESIAN_POINT ( 'NONE',  ( 44.59999999453762598, 168.7903194862797420, 4.480746418436729606 ) ) ;
#17081=CARTESIAN_POINT ( 'NONE',  ( 125.5000000000000000, 261.0000000000000000, 0.000000000000000000 ) ) ;
#17089=ORIENTED_EDGE ( 'NONE', *, *, #23274, .F. ) ;
#17090=CARTESIAN_POINT ( 'NONE',  ( 38.72499999726881015, 140.1801316387863778, -4.815267126137194431 ) ) ;
#17092=CARTESIAN_POINT ( 'NONE',  ( 117.5000000000000142, 155.0000000000000000, -70.00000000000002842 ) ) ;
#17097=CARTESIAN_POINT ( 'NONE',  ( 37.57499999726881157, 164.1591823560292198, -12.60653300113719766 ) ) ;
#17101=CARTESIAN_POINT ( 'NONE',  ( 60.59999999999999432, 159.7113355953771077, -14.50000000000000888 ) ) ;
#17106=CARTESIAN_POINT ( 'NONE',  ( 66.92499999726881299, 145.8408176439707802, -12.60653300113719588 ) ) ;
#17109=VERTEX_POINT ( 'NONE', #18828 ) ;
#17111=CARTESIAN_POINT ( 'NONE',  ( 80.17499999726881299, 164.1591823560292198, 12.60653300113718167 ) ) ;
#17124=ORIENTED_EDGE ( 'NONE', *, *, #15407, .T. ) ;
#17128=CARTESIAN_POINT ( 'NONE',  ( 87.22499999726881015, 160.0630714827496206, -15.58253175000000823 ) ) ;
#17130=CARTESIAN_POINT ( 'NONE',  ( 69.21132485994282035, 139.2280666364260071, -4.041636747397287284E-15 ) ) ;
#17131=CARTESIAN_POINT ( 'NONE',  ( 77.12499999726881583, 155.0000000000000000, -15.58253175000000823 ) ) ;
#17132=CARTESIAN_POINT ( 'NONE',  ( 32.50000000000000000, 155.0000000000000000, -6.938893903907228378E-15 ) ) ;
#17134=CARTESIAN_POINT ( 'NONE',  ( 87.50000000000002842, 170.3690997408855878, -1.377696575527767697 ) ) ;
#17135=CARTESIAN_POINT ( 'NONE',  ( 43.00000000000000711, 170.2462022514548323, -7.872454543227099337E-15 ) ) ;
#17138=CARTESIAN_POINT ( 'NONE',  ( 32.50000000000000000, 155.0000000000000000, 15.00000000000001243 ) ) ;
#17140=CARTESIAN_POINT ( 'NONE',  ( 48.42499999726881299, 141.7447067706911810, 9.630534252274376428 ) ) ;
#17141=CARTESIAN_POINT ( 'NONE',  ( 66.07499999726881867, 168.2552932293087906, 9.630534252274372875 ) ) ;
#17148=CARTESIAN_POINT ( 'NONE',  ( 84.19999999453763451, 163.5228861582408797, -11.73074641843674470 ) ) ;
#17156=CARTESIAN_POINT ( 'NONE',  ( 71.37499999726881583, 155.0000000000000000, -15.58253175000000823 ) ) ;
#17160=CARTESIAN_POINT ( 'NONE',  ( 85.57499999726880446, 164.1591823560292198, -12.60653300113719766 ) ) ;
#17170=CARTESIAN_POINT ( 'NONE',  ( 86.51132485994281751, 163.8167787843871110, 12.13525491562421621 ) ) ;
#17175=CARTESIAN_POINT ( 'NONE',  ( 71.11132485994281183, 140.7341522555726669, 4.635254915624211769 ) ) ;
#17179=CARTESIAN_POINT ( 'NONE',  ( 47.12499999726880873, 155.0000000000000000, -15.58253175000000823 ) ) ;
#17190=CARTESIAN_POINT ( 'NONE',  ( 66.79999999453762882, 163.5228861582408797, 11.73074641843673049 ) ) ;
#17201=CARTESIAN_POINT ( 'NONE',  ( 87.49999999999998579, 165.2808968839347301, -11.75397288630872694 ) ) ;
#17207=CARTESIAN_POINT ( 'NONE',  ( 57.47499999726879594, 160.0630714827496206, -15.58253175000000823 ) ) ;
#17213=CARTESIAN_POINT ( 'NONE',  ( 58.37499999726881583, 155.0000000000000000, 15.58253174999999402 ) ) ;
#17220=CARTESIAN_POINT ( 'NONE',  ( 80.00000000000001421, 139.7537977485451393, -4.138211985947621020E-15 ) ) ;
#17225=CARTESIAN_POINT ( 'NONE',  ( 45.77499999726881441, 169.8198683612136222, -4.815267126137197984 ) ) ;
#17228=CARTESIAN_POINT ( 'NONE',  ( 83.42499999726882720, 168.2552932293087906, -9.630534252274385310 ) ) ;
#17229=EDGE_CURVE ( 'NONE', #28697, #10467, #11001, .T. ) ;
#17232=CARTESIAN_POINT ( 'NONE',  ( 49.89999999453762314, 150.2886644046228639, -14.50000000000000888 ) ) ;
#17237=VERTEX_POINT ( 'NONE', #29724 ) ;
#17245=VERTEX_POINT ( 'NONE', #19162 ) ;
#17250=CARTESIAN_POINT ( 'NONE',  ( 35.27499999726881441, 149.9369285172503510, -15.58253175000000823 ) ) ;
#17253=CARTESIAN_POINT ( 'NONE',  ( 45.82499999726881157, 168.2552932293087906, 9.630534252274372875 ) ) ;
#17257=CARTESIAN_POINT ( 'NONE',  ( 38.87499999726880873, 138.6155565068815463, -3.929120461958505118E-15 ) ) ;
#17261=CARTESIAN_POINT ( 'NONE',  ( 61.40000000000000568, 159.7113355953771077, 14.49999999999999289 ) ) ;
#17268=CARTESIAN_POINT ( 'NONE',  ( 65.32499999726881867, 164.1591823560292198, -12.60653300113719766 ) ) ;
#17273=CARTESIAN_POINT ( 'NONE',  ( 82.17499999726882720, 164.1591823560292198, 12.60653300113718167 ) ) ;
#17278=AXIS2_PLACEMENT_3D ( 'NONE', #29343, #18782, #26770 ) ;
#17285=ORIENTED_EDGE ( 'NONE', *, *, #22941, .T. ) ;
#17297=CARTESIAN_POINT ( 'NONE',  ( 83.92499999726882720, 164.1591823560292198, 12.60653300113718167 ) ) ;
#17301=CARTESIAN_POINT ( 'NONE',  ( 75.02499999726879309, 149.9369285172503510, -15.58253175000000823 ) ) ;
#17306=CARTESIAN_POINT ( 'NONE',  ( 42.70000000000000284, 163.5228861582408797, -11.73074641843674470 ) ) ;
#17311=CARTESIAN_POINT ( 'NONE',  ( 50.32499999726881157, 145.8408176439707802, 12.60653300113718345 ) ) ;
#17312=CARTESIAN_POINT ( 'NONE',  ( 66.77499999726880731, 140.1801316387863778, 4.815267126137185549 ) ) ;
#17315=AXIS2_PLACEMENT_3D ( 'NONE', #30583, #10144, #2140 ) ;
#17331=CARTESIAN_POINT ( 'NONE',  ( 69.47499999726881015, 160.0630714827496206, -15.58253175000000823 ) ) ;
#17334=CARTESIAN_POINT ( 'NONE',  ( 82.27499999726880731, 160.0630714827496206, 15.58253174999999224 ) ) ;
#17335=CARTESIAN_POINT ( 'NONE',  ( 74.71132485994280614, 155.0000000000000000, 15.00000000000001243 ) ) ;
#17336=CARTESIAN_POINT ( 'NONE',  ( 32.50000000000000000, 155.0000000000000000, 15.00000000000001243 ) ) ;
#17338=CARTESIAN_POINT ( 'NONE',  ( 56.32499999726881157, 145.8408176439707802, 12.60653300113718345 ) ) ;
#17350=CARTESIAN_POINT ( 'NONE',  ( 66.98867513459482836, 163.8167787843871110, -12.13525491562423397 ) ) ;
#17355=CARTESIAN_POINT ( 'NONE',  ( 43.62499999726880162, 171.3844434931184253, -7.942151717890132712E-15 ) ) ;
#17356=CARTESIAN_POINT ( 'NONE',  ( 34.82499999726881157, 141.7447067706911810, -9.630534252274387086 ) ) ;
#17361=DIRECTION ( 'NONE',  ( 1.000000000000000000, 0.000000000000000000, 0.000000000000000000 ) ) ;
#17362=CARTESIAN_POINT ( 'NONE',  ( 34.78867513459482552, 155.0000000000000000, -15.00000000000002487 ) ) ;
#17365=CARTESIAN_POINT ( 'NONE',  ( 75.59999999453764019, 141.2096805137202580, -4.480746418436742040 ) ) ;
#17366=ORIENTED_EDGE ( 'NONE', *, *, #31990, .T. ) ;
#17373=ORIENTED_EDGE ( 'NONE', *, *, #17229, .T. ) ;
#17382=CARTESIAN_POINT ( 'NONE',  ( 56.87499999726880162, 138.6155565068815747, -3.929120461958505118E-15 ) ) ;
#17389=CARTESIAN_POINT ( 'NONE',  ( 66.17499999726881299, 164.1591823560292198, 12.60653300113718167 ) ) ;
#17393=CARTESIAN_POINT ( 'NONE',  ( 77.10000000000000853, 168.7903194862797420, 4.480746418436729606 ) ) ;
#17398=CARTESIAN_POINT ( 'NONE',  ( 50.57499999726881157, 145.8408176439707802, 12.60653300113718345 ) ) ;
#17400=CARTESIAN_POINT ( 'NONE',  ( 83.62499999726881583, 171.3844434931184253, -7.942151717890132712E-15 ) ) ;
#17402=DIRECTION ( 'NONE',  ( 0.000000000000000000, 1.000000000000000000, -1.290957005378097920E-14 ) ) ;
#17403=CARTESIAN_POINT ( 'NONE',  ( 48.49999999453761745, 170.2462022514548323, -7.872454543227099337E-15 ) ) ;
#17407=CARTESIAN_POINT ( 'NONE',  ( 61.41132485994281609, 142.2402378747194405, -9.270509831248439525 ) ) ;
#17414=EDGE_CURVE ( 'NONE', #27498, #3666, #33125, .T. ) ;
#17420=CARTESIAN_POINT ( 'NONE',  ( 38.07499999726880446, 168.2552932293087906, 9.630534252274372875 ) ) ;
#17422=CARTESIAN_POINT ( 'NONE',  ( 45.32499999726881157, 164.1591823560292198, -12.60653300113719766 ) ) ;
#17423=DIRECTION ( 'NONE',  ( 0.000000000000000000, 0.000000000000000000, 1.000000000000000000 ) ) ;
#17425=CARTESIAN_POINT ( 'NONE',  ( 54.11132485994280472, 169.2658477444273331, -4.635254915624224203 ) ) ;
#17427=CARTESIAN_POINT ( 'NONE',  ( 48.57499999726881157, 145.8408176439707802, 12.60653300113718345 ) ) ;
#17431=CARTESIAN_POINT ( 'NONE',  ( 58.80000000000000426, 167.3344367211045096, -8.961492836873482304 ) ) ;
#17438=CARTESIAN_POINT ( 'NONE',  ( 65.42499999726881299, 168.2552932293087906, -9.630534252274385310 ) ) ;
#17442=CARTESIAN_POINT ( 'NONE',  ( 84.77499999726880731, 140.1801316387863778, 4.815267126137185549 ) ) ;
#17446=AXIS2_PLACEMENT_3D ( 'NONE', #28303, #31033, #8025 ) ;
#17456=CARTESIAN_POINT ( 'NONE',  ( 32.50000000000000000, 155.0000000000000000, -6.938893903907228378E-15 ) ) ;
#17463=CARTESIAN_POINT ( 'NONE',  ( 81.01132485994281751, 142.2402378747194405, 9.270509831248432420 ) ) ;
#17464=CARTESIAN_POINT ( 'NONE',  ( 85.32499999726880446, 164.1591823560292198, -12.60653300113719766 ) ) ;
#17469=CARTESIAN_POINT ( 'NONE',  ( 38.90000000000000568, 168.7903194862797420, -4.480746418436745593 ) ) ;
#17473=CARTESIAN_POINT ( 'NONE',  ( 72.81132485994282888, 150.1262045565064227, 15.00000000000001599 ) ) ;
#17475=CARTESIAN_POINT ( 'NONE',  ( 51.42499999726879878, 168.2552932293087906, -9.630534252274387086 ) ) ;
#17476=CARTESIAN_POINT ( 'NONE',  ( 62.07499999726881157, 168.2552932293087906, 9.630534252274372875 ) ) ;
#17485=CARTESIAN_POINT ( 'NONE',  ( 83.11132485994279762, 140.7341522555726669, 4.635254915624211769 ) ) ;
#17493=CARTESIAN_POINT ( 'NONE',  ( 80.77499999726880731, 140.1801316387863778, 4.815267126137185549 ) ) ;
#17496=CARTESIAN_POINT ( 'NONE',  ( 74.12499999726881583, 155.0000000000000000, 15.58253174999999402 ) ) ;
#17498=CARTESIAN_POINT ( 'NONE',  ( 71.71132485994280614, 155.0000000000000000, -15.00000000000002487 ) ) ;
#17500=CARTESIAN_POINT ( 'NONE',  ( 59.82499999726879736, 168.2552932293087906, 9.630534252274372875 ) ) ;
#17502=CARTESIAN_POINT ( 'NONE',  ( 125.5000000000000000, 154.9999999999996305, -106.0000000000000142 ) ) ;
#17508=CARTESIAN_POINT ( 'NONE',  ( 68.71132485994280614, 155.0000000000000000, 15.00000000000001243 ) ) ;
#17518=CARTESIAN_POINT ( 'NONE',  ( 53.32499999726881157, 164.1591823560292198, -12.60653300113719766 ) ) ;
#17519=CARTESIAN_POINT ( 'NONE',  ( 87.50000000000002842, 156.3310307509052279, -15.36965516068564597 ) ) ;
#17525=UNCERTAINTY_MEASURE_WITH_UNIT (LENGTH_MEASURE( 1.000000000000000082E-05 ), #12784, 'distance_accuracy_value', 'NONE');
#17527=CARTESIAN_POINT ( 'NONE',  ( 84.98867513459481415, 163.8167787843871110, -12.13525491562423397 ) ) ;
#17530=CARTESIAN_POINT ( 'NONE',  ( 70.99999999453763166, 155.0000000000000000, 14.49999999999999467 ) ) ;
#17536=CARTESIAN_POINT ( 'NONE',  ( 74.81132485994281467, 150.1262045565064227, 15.00000000000001599 ) ) ;
#17546=CARTESIAN_POINT ( 'NONE',  ( 54.77499999726881441, 140.1801316387863778, 4.815267126137185549 ) ) ;
#17549=DIRECTION ( 'NONE',  ( 1.000000000000000000, 0.000000000000000000, 0.000000000000000000 ) ) ;
#17551=FILL_AREA_STYLE ('',( #7514 ) ) ;
#17554=AXIS2_PLACEMENT_3D ( 'NONE', #27670, #4504, #25113 ) ;
#17555=CARTESIAN_POINT ( 'NONE',  ( 64.07499999726881867, 168.2552932293087906, 9.630534252274372875 ) ) ;
#17560=CARTESIAN_POINT ( 'NONE',  ( 85.70000000000000284, 146.4771138417591203, 11.73074641843673227 ) ) ;
#17565=CARTESIAN_POINT ( 'NONE',  ( 52.57499999726881157, 145.8408176439707802, 12.60653300113718345 ) ) ;
#17567=CARTESIAN_POINT ( 'NONE',  ( 83.92499999726882720, 164.1591823560292198, 12.60653300113718167 ) ) ;
#17570=DIRECTION ( 'NONE',  ( 1.000000000000000000, 0.000000000000000000, 0.000000000000000000 ) ) ;
#17571=CARTESIAN_POINT ( 'NONE',  ( 51.09999999453761887, 150.2886644046228639, 14.49999999999999645 ) ) ;
#17578=AXIS2_PLACEMENT_3D ( 'NONE', #26848, #18846, #8787 ) ;
#17590=CARTESIAN_POINT ( 'NONE',  ( 36.77499999726881441, 140.1801316387863778, 4.815267126137185549 ) ) ;
#17591=ORIENTED_EDGE ( 'NONE', *, *, #1239, .T. ) ;
#17592=CARTESIAN_POINT ( 'NONE',  ( 43.62499999726880162, 171.3844434931184253, -7.942151717890132712E-15 ) ) ;
#17595=AXIS2_PLACEMENT_3D ( 'NONE', #26146, #9981, #10491 ) ;
#17597=CARTESIAN_POINT ( 'NONE',  ( 48.87499999726880873, 138.6155565068815463, -3.929120461958505118E-15 ) ) ;
#17602=CARTESIAN_POINT ( 'NONE',  ( 59.89999999999999858, 141.2096805137202580, 4.480746418436733158 ) ) ;
#17608=CIRCLE ( 'NONE', #30100, 100.0000000000000284 ) ;
#17611=ADVANCED_FACE ( 'NONE', ( #11838 ), #22223, .T. ) ;
#17613=CARTESIAN_POINT ( 'NONE',  ( 64.42499999726879878, 141.7447067706911810, 9.630534252274376428 ) ) ;
#17617=CARTESIAN_POINT ( 'NONE',  ( 88.27499999726880731, 160.0630714827496206, 15.58253174999999402 ) ) ;
#17637=EDGE_CURVE ( 'NONE', #29444, #21593, #18652, .T. ) ;
#17638=CARTESIAN_POINT ( 'NONE',  ( 81.62499999726878741, 171.3844434931184253, -7.942151717890132712E-15 ) ) ;
#17643=CARTESIAN_POINT ( 'NONE',  ( 41.50000000000000000, 155.0000000000000000, 14.49999999999999467 ) ) ;
#17647=CARTESIAN_POINT ( 'NONE',  ( 78.48867513459484258, 142.2402378747194405, -9.270509831248439525 ) ) ;
#17649=CARTESIAN_POINT ( 'NONE',  ( 60.52499999726881441, 140.1801316387863778, 4.815267126137185549 ) ) ;
#17650=CARTESIAN_POINT ( 'NONE',  ( 63.27499999726881441, 149.9369285172503510, -15.58253175000000823 ) ) ;
#17668=CARTESIAN_POINT ( 'NONE',  ( 79.07499999726880446, 141.7447067706911810, -9.630534252274385310 ) ) ;
#17670=EDGE_LOOP ( 'NONE', ( #6255, #11128, #819, #11716 ) ) ;
#17672=CARTESIAN_POINT ( 'NONE',  ( 71.02499999726882152, 149.9369285172503510, -15.58253175000000823 ) ) ;
#17676=CARTESIAN_POINT ( 'NONE',  ( 65.22499999726881015, 160.0630714827496206, -15.58253175000000823 ) ) ;
#17692=CARTESIAN_POINT ( 'NONE',  ( 38.22499999726881015, 149.9369285172503510, 15.58253174999999580 ) ) ;
#17697=CARTESIAN_POINT ( 'NONE',  ( 32.81249999863440792, 155.0000000000000000, -15.04126587500000767 ) ) ;
#17701=CARTESIAN_POINT ( 'NONE',  ( 72.29999999453761461, 167.3344367211045096, -8.961492836873482304 ) ) ;
#17709=ORIENTED_EDGE ( 'NONE', *, *, #18490, .T. ) ;
#17713=FACE_OUTER_BOUND ( 'NONE', #18231, .T. ) ;
#17715=EDGE_LOOP ( 'NONE', ( #8777, #13318 ) ) ;
#17716=( BOUNDED_CURVE ( )  B_SPLINE_CURVE ( 2, ( #15834, #29116, #664, #13605, #6271, #3550, #27229, #24170, #21606, #8497, #8666 ),
 .UNSPECIFIED., .F., .T. ) 
 B_SPLINE_CURVE_WITH_KNOTS ( ( 3, 2, 2, 2, 2, 3 ),
 ( 0.7857142857142856984, 0.7892857142857142572, 0.7928571428571428159, 0.7964285714285713746, 0.7999999999999999334, 0.8035714285714284921 ),
 .UNSPECIFIED. ) 
 CURVE ( )  GEOMETRIC_REPRESENTATION_ITEM ( )  RATIONAL_B_SPLINE_CURVE ( ( 1.000000000000000000, 0.9510565162951534202, 1.000000000000000000, 0.9510565162951534202, 1.000000000000000000, 0.9510565162951534202, 1.000000000000000000, 0.9510565162951534202, 1.000000000000000000, 0.9510565162951534202, 1.000000000000000000 ) ) 
 REPRESENTATION_ITEM ( '' )  );
#17721=CARTESIAN_POINT ( 'NONE',  ( 56.97499999726881015, 140.1801316387863778, -4.815267126137194431 ) ) ;
#17724=CARTESIAN_POINT ( 'NONE',  ( 56.78867513459481842, 155.0000000000000000, -15.00000000000002487 ) ) ;
#17725=( LENGTH_UNIT ( ) NAMED_UNIT ( * ) SI_UNIT ( .MILLI., .METRE. ) );
#17728=CARTESIAN_POINT ( 'NONE',  ( 66.07499999726881867, 168.2552932293087906, 9.630534252274372875 ) ) ;
#17734=CARTESIAN_POINT ( 'NONE',  ( 86.50000000000000000, 155.0000000000000000, -14.50000000000000711 ) ) ;
#17735=CARTESIAN_POINT ( 'NONE',  ( 40.78867513459481842, 155.0000000000000000, -15.00000000000002487 ) ) ;
#17737=DIRECTION ( 'NONE',  ( 1.000000000000000000, 0.000000000000000000, 0.000000000000000000 ) ) ;
#17738=CARTESIAN_POINT ( 'NONE',  ( 53.97499999726881015, 169.8198683612136222, 4.815267126137181997 ) ) ;
#17740=CYLINDRICAL_SURFACE ( 'NONE', #7240, 15.00000000000001776 ) ;
#17742=CARTESIAN_POINT ( 'NONE',  ( 64.91132485994280898, 146.1832212156128890, 12.13525491562421976 ) ) ;
#17743=CARTESIAN_POINT ( 'NONE',  ( 55.29999999453762882, 142.6655632788954620, 8.961492836873471646 ) ) ;
#17752=ORIENTED_EDGE ( 'NONE', *, *, #33099, .F. ) ;
#17755=EDGE_LOOP ( 'NONE', ( #16324, #8367 ) ) ;
#17758=CARTESIAN_POINT ( 'NONE',  ( 39.37499999726880873, 155.0000000000000000, -15.58253175000000823 ) ) ;
#17760=CARTESIAN_POINT ( 'NONE',  ( 43.52499999726881441, 169.8198683612136222, -4.815267126137197984 ) ) ;
#17765=CARTESIAN_POINT ( 'NONE',  ( 47.87499999726880162, 171.3844434931184253, -7.942151717890132712E-15 ) ) ;
#17770=CARTESIAN_POINT ( 'NONE',  ( 69.29999999999999716, 163.5228861582408797, 11.73074641843673049 ) ) ;
#17777=CARTESIAN_POINT ( 'NONE',  ( 63.12499999726880873, 155.0000000000000000, -15.58253175000000823 ) ) ;
#17781=CARTESIAN_POINT ( 'NONE',  ( 88.17499999726881299, 164.1591823560292198, 12.60653300113718167 ) ) ;
#17796=DIRECTION ( 'NONE',  ( 1.000000000000000000, 0.000000000000000000, 0.000000000000000000 ) ) ;
#17805=CARTESIAN_POINT ( 'NONE',  ( 83.82499999726880446, 168.2552932293087906, 9.630534252274372875 ) ) ;
#17809=CIRCLE ( 'NONE', #31947, 15.00000000000001776 ) ;
#17810=CARTESIAN_POINT ( 'NONE',  ( 45.10000000000000142, 168.7903194862797420, 4.480746418436729606 ) ) ;
#17815=CARTESIAN_POINT ( 'NONE',  ( 54.42499999726881299, 141.7447067706911810, 9.630534252274376428 ) ) ;
#17816=CARTESIAN_POINT ( 'NONE',  ( 71.47499999726879594, 160.0630714827496206, -15.58253175000000823 ) ) ;
#17824=CARTESIAN_POINT ( 'NONE',  ( 83.61132485994282604, 150.1262045565064227, -15.00000000000002665 ) ) ;
#17834=CARTESIAN_POINT ( 'NONE',  ( 78.07499999726880446, 168.2552932293087906, 9.630534252274372875 ) ) ;
#17837=EDGE_CURVE ( 'NONE', #7110, #13563, #19713, .T. ) ;
#17839=CARTESIAN_POINT ( 'NONE',  ( 72.02499999726882152, 160.0630714827496206, 15.58253174999999224 ) ) ;
#17843=CARTESIAN_POINT ( 'NONE',  ( 66.22499999726879594, 149.9369285172503510, 15.58253174999999580 ) ) ;
#17863=CARTESIAN_POINT ( 'NONE',  ( 38.82499999726881157, 141.7447067706911810, -9.630534252274387086 ) ) ;
#17867=( BOUNDED_CURVE ( )  B_SPLINE_CURVE ( 2, ( #6179, #27138, #19131, #6525, #27301, #5842, #24073, #19637, #16904, #3623, #24238 ),
 .UNSPECIFIED., .F., .T. ) 
 B_SPLINE_CURVE_WITH_KNOTS ( ( 3, 2, 2, 2, 2, 3 ),
 ( 0.1428571428571427104, 0.1464285714285713247, 0.1499999999999999112, 0.1535714285714285254, 0.1571428571428572230, 0.1607142857142858372 ),
 .UNSPECIFIED. ) 
 CURVE ( )  GEOMETRIC_REPRESENTATION_ITEM ( )  RATIONAL_B_SPLINE_CURVE ( ( 1.000000000000001110, 0.9510565162951523099, 1.000000000000000000, 0.9510565162951534202, 1.000000000000000000, 0.9510565162951534202, 1.000000000000000000, 0.9510565162951534202, 1.000000000000000000, 0.9510565162951515328, 1.000000000000001998 ) ) 
 REPRESENTATION_ITEM ( '' )  );
#17871=LINE ( 'NONE', #17697, #30114 ) ;
#17874=CARTESIAN_POINT ( 'NONE',  ( 72.89999999453765156, 159.7113355953771077, 14.49999999999999289 ) ) ;
#17880=CARTESIAN_POINT ( 'NONE',  ( 75.41132485994282320, 142.2402378747194405, -9.270509831248439525 ) ) ;
#17883=ORIENTED_EDGE ( 'NONE', *, *, #24979, .F. ) ;
#17888=CIRCLE ( 'NONE', #3187, 30.00000000000000000 ) ;
#17894=CARTESIAN_POINT ( 'NONE',  ( 54.07499999726880446, 168.2552932293087906, 9.630534252274372875 ) ) ;
#17895=VERTEX_POINT ( 'NONE', #31088 ) ;
#17901=CARTESIAN_POINT ( 'NONE',  ( 63.27499999726881441, 149.9369285172503510, -15.58253175000000823 ) ) ;
#17904=EDGE_CURVE ( 'NONE', #1328, #29866, #13345, .T. ) ;
#17909=CARTESIAN_POINT ( 'NONE',  ( 84.30000000000001137, 146.4771138417591203, -11.73074641843674470 ) ) ;
#17910=CARTESIAN_POINT ( 'NONE',  ( 81.48867513459484258, 167.7597621252805880, 9.270509831248428867 ) ) ;
#17911=CYLINDRICAL_SURFACE ( 'NONE', #17446, 15.00000000000001776 ) ;
#17915=CARTESIAN_POINT ( 'NONE',  ( 50.67499999726880588, 141.7447067706911810, 9.630534252274376428 ) ) ;
#17918=CARTESIAN_POINT ( 'NONE',  ( 87.22499999726881015, 160.0630714827496206, -15.58253175000000823 ) ) ;
#17921=CARTESIAN_POINT ( 'NONE',  ( 40.02499999726881441, 160.0630714827496206, 15.58253174999999224 ) ) ;
#17923=CARTESIAN_POINT ( 'NONE',  ( 56.19999999453763451, 163.5228861582408797, -11.73074641843674470 ) ) ;
#17924=ORIENTED_EDGE ( 'NONE', *, *, #12703, .T. ) ;
#17931=( BOUNDED_CURVE ( )  B_SPLINE_CURVE ( 2, ( #9254, #32926, #20148, #22878, #17425, #30546, #19979, #9766, #30380, #14865, #14697 ),
 .UNSPECIFIED., .F., .T. ) 
 B_SPLINE_CURVE_WITH_KNOTS ( ( 3, 2, 2, 2, 2, 3 ),
 ( 0.3571428571428570398, 0.3607142857142855985, 0.3642857142857141572, 0.3678571428571427715, 0.3714285714285713302, 0.3749999999999998890 ),
 .UNSPECIFIED. ) 
 CURVE ( )  GEOMETRIC_REPRESENTATION_ITEM ( )  RATIONAL_B_SPLINE_CURVE ( ( 1.000000000000001554, 0.9510565162951518658, 1.000000000000000000, 0.9510565162951534202, 1.000000000000000000, 0.9510565162951534202, 1.000000000000000000, 0.9510565162951534202, 1.000000000000000000, 0.9510565162951549745, 0.9999999999999984457 ) ) 
 REPRESENTATION_ITEM ( '' )  );
#17936=CARTESIAN_POINT ( 'NONE',  ( 79.78867513459482552, 155.0000000000000000, 15.00000000000001243 ) ) ;
#17941=CARTESIAN_POINT ( 'NONE',  ( 39.87499999726879452, 171.3844434931184253, -7.942151717890134290E-15 ) ) ;
#17942=ORIENTED_EDGE ( 'NONE', *, *, #1615, .T. ) ;
#17943=CARTESIAN_POINT ( 'NONE',  ( 41.72499999726881015, 169.8198683612136222, 4.815267126137181997 ) ) ;
#17947=CARTESIAN_POINT ( 'NONE',  ( 48.07499999726881867, 168.2552932293087906, 9.630534252274372875 ) ) ;
#17950=CARTESIAN_POINT ( 'NONE',  ( 127.5000000000000000, 155.0000000000000000, 100.0000000000000000 ) ) ;
#17952=CARTESIAN_POINT ( 'NONE',  ( 68.29999999999999716, 146.4771138417591203, -11.73074641843674470 ) ) ;
#17956=CARTESIAN_POINT ( 'NONE',  ( 57.58867513459482979, 163.8167787843871110, 12.13525491562421621 ) ) ;
#17960=CARTESIAN_POINT ( 'NONE',  ( 72.02499999726882152, 160.0630714827496206, 15.58253174999999402 ) ) ;
#17963=CARTESIAN_POINT ( 'NONE',  ( 34.59999999453763309, 168.7903194862797420, 4.480746418436729606 ) ) ;
#17966=ORIENTED_EDGE ( 'NONE', *, *, #18983, .T. ) ;
#17976=VERTEX_POINT ( 'NONE', #32074 ) ;
#17977=CARTESIAN_POINT ( 'NONE',  ( 34.51132485994281041, 163.8167787843871110, 12.13525491562421621 ) ) ;
#17981=CARTESIAN_POINT ( 'NONE',  ( 83.32499999726880446, 164.1591823560292198, -12.60653300113719766 ) ) ;
#17986=CARTESIAN_POINT ( 'NONE',  ( 48.89999999999999858, 168.7903194862797420, -4.480746418436745593 ) ) ;
#17988=CARTESIAN_POINT ( 'NONE',  ( 67.48867513459484258, 167.7597621252805880, 9.270509831248428867 ) ) ;
#17994=CARTESIAN_POINT ( 'NONE',  ( 55.62499999726881583, 171.3844434931184253, -7.942151717890134290E-15 ) ) ;
#17995=CARTESIAN_POINT ( 'NONE',  ( 69.07499999726881867, 141.7447067706911810, -9.630534252274385310 ) ) ;
#18004=CARTESIAN_POINT ( 'NONE',  ( 68.71132485994280614, 155.0000000000000000, 15.00000000000001243 ) ) ;
#18011=CARTESIAN_POINT ( 'NONE',  ( 76.57499999726881867, 145.8408176439707802, 12.60653300113718345 ) ) ;
#18014=CARTESIAN_POINT ( 'NONE',  ( 74.02499999726879309, 160.0630714827496206, 15.58253174999999224 ) ) ;
#18018=CARTESIAN_POINT ( 'NONE',  ( 63.52499999726880731, 169.8198683612136222, -4.815267126137197984 ) ) ;
#18023=CARTESIAN_POINT ( 'NONE',  ( 127.5000000000000000, 229.9533188057749555, 74.95331880577313655 ) ) ;
#18026=CARTESIAN_POINT ( 'NONE',  ( 117.5000000000000142, 155.0000000000000000, -100.0000000000000284 ) ) ;
#18030=CARTESIAN_POINT ( 'NONE',  ( 46.08867513459482979, 142.2402378747194405, 9.270509831248432420 ) ) ;
#18032=CARTESIAN_POINT ( 'NONE',  ( 38.02499999726881441, 160.0630714827496206, 15.58253174999999224 ) ) ;
#18042=CARTESIAN_POINT ( 'NONE',  ( 74.09999999453764019, 159.7113355953771077, -14.50000000000000888 ) ) ;
#18048=ADVANCED_FACE ( 'NONE', ( #18795 ), #21341, .T. ) ;
#18051=ORIENTED_EDGE ( 'NONE', *, *, #21846, .F. ) ;
#18052=FACE_OUTER_BOUND ( 'NONE', #12267, .T. ) ;
#18053=CARTESIAN_POINT ( 'NONE',  ( 32.50000000000000000, 155.0000000000000000, -6.938893903907228378E-15 ) ) ;
#18058=CARTESIAN_POINT ( 'NONE',  ( 61.27499999726881441, 149.9369285172503510, -15.58253175000000823 ) ) ;
#18065=CARTESIAN_POINT ( 'NONE',  ( 86.91132485994280898, 146.1832212156128890, 12.13525491562421976 ) ) ;
#18066=( BOUNDED_CURVE ( )  B_SPLINE_CURVE ( 2, ( #25649, #32341, #1344, #14623, #11731, #9006, #6788, #4060, #7606, #20537, #2316 ),
 .UNSPECIFIED., .F., .F. ) 
 B_SPLINE_CURVE_WITH_KNOTS ( ( 3, 2, 2, 2, 2, 3 ),
 ( 0.07142857142857135522, 0.07499999999999992784, 0.07857142857142850045, 0.08214285714285708695, 0.08571428571428565957, 0.08928571428571423219 ),
 .UNSPECIFIED. ) 
 CURVE ( )  GEOMETRIC_REPRESENTATION_ITEM ( )  RATIONAL_B_SPLINE_CURVE ( ( 1.000000000000000888, 0.9510565162951523099, 1.000000000000000000, 0.9510565162951534202, 1.000000000000000000, 0.9510565162951534202, 1.000000000000000000, 0.9510565162951534202, 1.000000000000000000, 0.9510565162951541973, 0.9999999999999992228 ) ) 
 REPRESENTATION_ITEM ( '' )  );
#18071=VECTOR ( 'NONE', #6416, 1000.000000000000000 ) ;
#18072=CARTESIAN_POINT ( 'NONE',  ( 85.00000000000001421, 170.2462022514548323, -7.872454543227099337E-15 ) ) ;
#18077=CARTESIAN_POINT ( 'NONE',  ( 49.67499999726879878, 168.2552932293087906, -9.630534252274385310 ) ) ;
#18080=CARTESIAN_POINT ( 'NONE',  ( 35.31132485994280046, 140.7341522555726669, -4.635254915624220651 ) ) ;
#18081=CARTESIAN_POINT ( 'NONE',  ( 52.41132485994280898, 167.7597621252805880, 9.270509831248428867 ) ) ;
#18083=CARTESIAN_POINT ( 'NONE',  ( 51.29999999453762172, 142.6655632788954620, 8.961492836873471646 ) ) ;
#18086=CARTESIAN_POINT ( 'NONE',  ( 47.11132485994280472, 140.7341522555726669, 4.635254915624211769 ) ) ;
#18088=CARTESIAN_POINT ( 'NONE',  ( 60.21132485994281325, 170.7719333635740497, -7.904646289410545231E-15 ) ) ;
#18094=VERTEX_POINT ( 'NONE', #29517 ) ;
#18103=CARTESIAN_POINT ( 'NONE',  ( 46.87499999726880873, 138.6155565068815747, -3.929120461958505118E-15 ) ) ;
#18104=VERTEX_POINT ( 'NONE', #6340 ) ;
#18105=CARTESIAN_POINT ( 'NONE',  ( 51.52499999726881441, 169.8198683612136222, -4.815267126137197984 ) ) ;
#18106=CARTESIAN_POINT ( 'NONE',  ( 125.5000000000000000, 261.0000000000000000, 0.000000000000000000 ) ) ;
#18109=CARTESIAN_POINT ( 'NONE',  ( 47.07499999726880446, 141.7447067706911810, -9.630534252274385310 ) ) ;
#18110=CARTESIAN_POINT ( 'NONE',  ( 79.11132485994279762, 140.7341522555726669, 4.635254915624211769 ) ) ;
#18112=DIRECTION ( 'NONE',  ( -1.000000000000000000, 0.000000000000000000, 0.000000000000000000 ) ) ;
#18114=CARTESIAN_POINT ( 'NONE',  ( 66.59999999999999432, 159.7113355953771077, -14.50000000000000888 ) ) ;
#18121=CARTESIAN_POINT ( 'NONE',  ( 72.22499999726881015, 149.9369285172503510, 15.58253174999999580 ) ) ;
#18122=ORIENTED_EDGE ( 'NONE', *, *, #3976, .T. ) ;
#18125=CARTESIAN_POINT ( 'NONE',  ( 87.27499999726880731, 149.9369285172503510, -15.58253175000000823 ) ) ;
#18127=AXIS2_PLACEMENT_3D ( 'NONE', #17456, #14727, #2298 ) ;
#18129=ORIENTED_EDGE ( 'NONE', *, *, #14549, .T. ) ;
#18134=EDGE_LOOP ( 'NONE', ( #26139, #33632, #12855, #12096 ) ) ;
#18146=CARTESIAN_POINT ( 'NONE',  ( 87.41151231482329820, 167.7028228021052314, -10.03192751310307784 ) ) ;
#18152=CARTESIAN_POINT ( 'NONE',  ( 84.92499999726882720, 145.8408176439707802, -12.60653300113719588 ) ) ;
#18157=CARTESIAN_POINT ( 'NONE',  ( 48.59999999999999432, 159.7113355953771077, -14.50000000000000888 ) ) ;
#18160=CARTESIAN_POINT ( 'NONE',  ( 50.02499999726880020, 160.0630714827496206, 15.58253174999999402 ) ) ;
#18164=CARTESIAN_POINT ( 'NONE',  ( 54.32499999726880446, 145.8408176439707802, 12.60653300113718345 ) ) ;
#18165=CARTESIAN_POINT ( 'NONE',  ( 73.07499999726880446, 141.7447067706911810, -9.630534252274385310 ) ) ;
#18181=ORIENTED_EDGE ( 'NONE', *, *, #31340, .F. ) ;
#18182=CARTESIAN_POINT ( 'NONE',  ( 79.67499999726881299, 168.2552932293087906, -9.630534252274385310 ) ) ;
#18185=CARTESIAN_POINT ( 'NONE',  ( 70.42499999726881299, 141.7447067706911810, 9.630534252274376428 ) ) ;
#18187=DIRECTION ( 'NONE',  ( 0.000000000000000000, -1.000000000000000000, 1.290957005378097920E-14 ) ) ;
#18188=CARTESIAN_POINT ( 'NONE',  ( 60.62499999726879452, 138.6155565068815463, -3.929120461958505118E-15 ) ) ;
#18199=CARTESIAN_POINT ( 'NONE',  ( 44.88867513459483405, 159.8737954434937478, -14.99999999999993072 ) ) ;
#18203=CARTESIAN_POINT ( 'NONE',  ( 46.48867513459483547, 142.2402378747194405, -9.270509831248439525 ) ) ;
#18205=CARTESIAN_POINT ( 'NONE',  ( 39.52499999726881441, 169.8198683612136222, -4.815267126137197984 ) ) ;
#18210=CARTESIAN_POINT ( 'NONE',  ( 37.71132485994279904, 155.0000000000000000, -15.00000000000002487 ) ) ;
#18213=CARTESIAN_POINT ( 'NONE',  ( 78.29999999453762882, 167.3344367211045096, -8.961492836873482304 ) ) ;
#18223=CARTESIAN_POINT ( 'NONE',  ( 78.71132485994280614, 155.0000000000000000, 15.00000000000001243 ) ) ;
#18225=EDGE_LOOP ( 'NONE', ( #4052, #29768, #3367, #19666, #19213 ) ) ;
#18230=CARTESIAN_POINT ( 'NONE',  ( 61.37499999726880873, 155.0000000000000000, -15.58253175000000823 ) ) ;
#18231=EDGE_LOOP ( 'NONE', ( #21602, #17709, #9763, #32072 ) ) ;
#18234=DIRECTION ( 'NONE',  ( 0.000000000000000000, 0.000000000000000000, -1.000000000000000000 ) ) ;
#18242=CARTESIAN_POINT ( 'NONE',  ( 35.32499999726881157, 164.1591823560292198, -12.60653300113719766 ) ) ;
#18247=CARTESIAN_POINT ( 'NONE',  ( 56.47499999726881015, 149.9369285172503510, 15.58253174999999580 ) ) ;
#18249=CARTESIAN_POINT ( 'NONE',  ( 34.91132485994280188, 146.1832212156128890, 12.13525491562421976 ) ) ;
#18252=CARTESIAN_POINT ( 'NONE',  ( 53.89999999453762314, 150.2886644046228639, -14.50000000000000888 ) ) ;
#18257=FACE_OUTER_BOUND ( 'NONE', #19008, .T. ) ;
#18262=CARTESIAN_POINT ( 'NONE',  ( 80.58867513459483689, 146.1832212156128890, -12.13525491562423042 ) ) ;
#18265=( BOUNDED_CURVE ( )  B_SPLINE_CURVE ( 2, ( #18302, #28694, #13349, #23743, #5352, #15742, #26138, #2805, #21185, #13187, #23585 ),
 .UNSPECIFIED., .F., .T. ) 
 B_SPLINE_CURVE_WITH_KNOTS ( ( 3, 2, 2, 2, 2, 3 ),
 ( 0.7142857142857141906, 0.7178571428571427493, 0.7214285714285713080, 0.7249999999999999778, 0.7285714285714285365, 0.7321428571428570953 ),
 .UNSPECIFIED. ) 
 CURVE ( )  GEOMETRIC_REPRESENTATION_ITEM ( )  RATIONAL_B_SPLINE_CURVE ( ( 1.000000000000001554, 0.9510565162951518658, 1.000000000000000000, 0.9510565162951534202, 1.000000000000000000, 0.9510565162951534202, 1.000000000000000000, 0.9510565162951534202, 1.000000000000000000, 0.9510565162951534202, 1.000000000000000000 ) ) 
 REPRESENTATION_ITEM ( '' )  );
#18268=CARTESIAN_POINT ( 'NONE',  ( 41.17499999726881299, 145.8408176439707802, -12.60653300113719588 ) ) ;
#18270=CARTESIAN_POINT ( 'NONE',  ( 52.42499999726880588, 141.7447067706911810, 9.630534252274376428 ) ) ;
#18271=CARTESIAN_POINT ( 'NONE',  ( 79.71132485994280614, 155.0000000000000000, -15.00000000000002487 ) ) ;
#18274=CARTESIAN_POINT ( 'NONE',  ( 50.37499999726881583, 155.0000000000000000, 15.58253174999999402 ) ) ;
#18275=CARTESIAN_POINT ( 'NONE',  ( 79.71132485994280614, 155.0000000000000000, -15.00000000000002487 ) ) ;
#18279=CARTESIAN_POINT ( 'NONE',  ( 65.40000000000000568, 159.7113355953771077, 14.49999999999999289 ) ) ;
#18284=CARTESIAN_POINT ( 'NONE',  ( 38.27499999726881441, 160.0630714827496206, 15.58253174999999402 ) ) ;
#18286=CARTESIAN_POINT ( 'NONE',  ( 73.72499999726881015, 169.8198683612136222, 4.815267126137181997 ) ) ;
#18289=CARTESIAN_POINT ( 'NONE',  ( 35.39999999453763024, 141.2096805137202580, 4.480746418436733158 ) ) ;
#18302=CARTESIAN_POINT ( 'NONE',  ( 73.71132485994280614, 155.0000000000000000, -15.00000000000002487 ) ) ;
#18310=CARTESIAN_POINT ( 'NONE',  ( 33.62499999726881583, 171.3844434931184253, -7.942151717890132712E-15 ) ) ;
#18311=CARTESIAN_POINT ( 'NONE',  ( 34.27499999726880731, 160.0630714827496206, 15.58253174999999402 ) ) ;
#18315=CARTESIAN_POINT ( 'NONE',  ( 45.39999999999999858, 159.7113355953771077, 14.49999999999999289 ) ) ;
#18317=LINE ( 'NONE', #16084, #33583 ) ;
#18320=CARTESIAN_POINT ( 'NONE',  ( 50.72499999726881725, 140.1801316387863778, -4.815267126137194431 ) ) ;
#18323=CARTESIAN_POINT ( 'NONE',  ( 66.12499999726881583, 155.0000000000000000, 15.58253174999999402 ) ) ;
#18324=CARTESIAN_POINT ( 'NONE',  ( 67.37499999726881583, 155.0000000000000000, -15.58253175000000823 ) ) ;
#18326=CARTESIAN_POINT ( 'NONE',  ( 45.71132485994280614, 155.0000000000000000, -15.00000000000002487 ) ) ;
#18331=VECTOR ( 'NONE', #14734, 1000.000000000000000 ) ;
#18335=CARTESIAN_POINT ( 'NONE',  ( 33.88867513459481984, 150.1262045565062806, 14.99999999999992006 ) ) ;
#18342=ORIENTED_EDGE ( 'NONE', *, *, #29441, .T. ) ;
#18346=ORIENTED_EDGE ( 'NONE', *, *, #9576, .T. ) ;
#18348=CARTESIAN_POINT ( 'NONE',  ( 79.82499999726881867, 168.2552932293087906, 9.630534252274372875 ) ) ;
#18351=CARTESIAN_POINT ( 'NONE',  ( 62.12499999726880873, 155.0000000000000000, 15.58253174999999402 ) ) ;
#18352=CARTESIAN_POINT ( 'NONE',  ( 32.50000000000000000, 155.0000000000000000, -6.938893903907228378E-15 ) ) ;
#18362=CARTESIAN_POINT ( 'NONE',  ( 63.08867513459481557, 167.7597621252805880, -9.270509831248443078 ) ) ;
#18369=CARTESIAN_POINT ( 'NONE',  ( 35.92499999726880588, 164.1591823560292198, 12.60653300113718167 ) ) ;
#18378=CARTESIAN_POINT ( 'NONE',  ( 81.69999999453762030, 142.6655632788954620, -8.961492836873480528 ) ) ;
#18395=CARTESIAN_POINT ( 'NONE',  ( 64.57499999726881867, 145.8408176439707802, 12.60653300113718345 ) ) ;
#18397=CARTESIAN_POINT ( 'NONE',  ( 68.78867513459482552, 155.0000000000000000, -15.00000000000002487 ) ) ;
#18402=CARTESIAN_POINT ( 'NONE',  ( 87.11132485994279762, 140.7341522555726669, 4.635254915624211769 ) ) ;
#18408=CARTESIAN_POINT ( 'NONE',  ( 41.22499999726881015, 160.0630714827496206, -15.58253175000000823 ) ) ;
#18412=CARTESIAN_POINT ( 'NONE',  ( 63.98867513459482836, 146.1832212156128890, 12.13525491562421976 ) ) ;
#18413=CARTESIAN_POINT ( 'NONE',  ( 60.07499999726879736, 168.2552932293087906, 9.630534252274372875 ) ) ;
#18416=CARTESIAN_POINT ( 'NONE',  ( 87.62499999726880162, 171.3844434931184253, -7.942151717890132712E-15 ) ) ;
#18419=CARTESIAN_POINT ( 'NONE',  ( 61.79999999453762882, 146.4771138417591203, -11.73074641843674470 ) ) ;
#18427=CARTESIAN_POINT ( 'NONE',  ( 72.61132485994281183, 159.8737954434936057, 15.00000000000001421 ) ) ;
#18432=CARTESIAN_POINT ( 'NONE',  ( 70.71132485994280614, 155.0000000000000000, 15.00000000000001243 ) ) ;
#18433=CARTESIAN_POINT ( 'NONE',  ( 32.50000000000000000, 155.0000000000000000, 13.00000000000001066 ) ) ;
#18437=CARTESIAN_POINT ( 'NONE',  ( 44.87499999726880873, 138.6155565068815747, -3.929120461958505118E-15 ) ) ;
#18439=CARTESIAN_POINT ( 'NONE',  ( 53.62499999726881583, 171.3844434931184253, -7.942151717890132712E-15 ) ) ;
#18444=CARTESIAN_POINT ( 'NONE',  ( 54.57499999726881157, 145.8408176439707802, 12.60653300113718345 ) ) ;
#18445=CARTESIAN_POINT ( 'NONE',  ( 52.38867513459481984, 140.7341522555726669, -4.635254915624220651 ) ) ;
#18450=CARTESIAN_POINT ( 'NONE',  ( 68.09999999999999432, 141.2096805137202580, -4.480746418436742040 ) ) ;
#18452=CARTESIAN_POINT ( 'NONE',  ( 38.58867513459482268, 146.1832212156128890, -12.13525491562423042 ) ) ;
#18454=DIRECTION ( 'NONE',  ( 1.000000000000000000, 0.000000000000000000, 0.000000000000000000 ) ) ;
#18455=CARTESIAN_POINT ( 'NONE',  ( 38.17499999726881299, 164.1591823560292198, 12.60653300113718167 ) ) ;
#18458=CARTESIAN_POINT ( 'NONE',  ( 67.72499999726881015, 169.8198683612136222, 4.815267126137181997 ) ) ;
#18461=CARTESIAN_POINT ( 'NONE',  ( 41.09999999453763309, 150.2886644046228639, 14.49999999999999645 ) ) ;
#18463=PLANE ( 'NONE',  #26806 ) ;
#18464=EDGE_CURVE ( 'NONE', #7333, #33037, #14382, .T. ) ;
#18468=CARTESIAN_POINT ( 'NONE',  ( 117.5000000000000142, 155.0000000000000000, 70.00000000000000000 ) ) ;
#18472=VERTEX_POINT ( 'NONE', #13887 ) ;
#18482=CARTESIAN_POINT ( 'NONE',  ( 33.77499999726880731, 169.8198683612136222, -4.815267126137197984 ) ) ;
#18486=CARTESIAN_POINT ( 'NONE',  ( 47.30000000000000426, 163.5228861582408797, 11.73074641843673049 ) ) ;
#18489=CARTESIAN_POINT ( 'NONE',  ( 83.71132485994282035, 155.0000000000000000, -15.00000000000002487 ) ) ;
#18490=EDGE_CURVE ( 'NONE', #7971, #14298, #27208, .T. ) ;
#18491=CARTESIAN_POINT ( 'NONE',  ( 51.22499999726881015, 160.0630714827496206, -15.58253175000000823 ) ) ;
#18494=CARTESIAN_POINT ( 'NONE',  ( 65.92499999726881299, 164.1591823560292198, 12.60653300113718167 ) ) ;
#18495=CARTESIAN_POINT ( 'NONE',  ( 74.77499999726880731, 140.1801316387863778, 4.815267126137185549 ) ) ;
#18497=DIRECTION ( 'NONE',  ( 0.000000000000000000, 0.000000000000000000, -1.000000000000000000 ) ) ;
#18500=CARTESIAN_POINT ( 'NONE',  ( 35.28867513459481842, 170.7719333635740497, -7.904646289410545231E-15 ) ) ;
#18517=CARTESIAN_POINT ( 'NONE',  ( 78.82499999726881867, 141.7447067706911810, -9.630534252274387086 ) ) ;
#18521=CARTESIAN_POINT ( 'NONE',  ( 72.02499999726882152, 160.0630714827496206, 15.58253174999999402 ) ) ;
#18534=CARTESIAN_POINT ( 'NONE',  ( 86.97499999726882436, 140.1801316387863778, -4.815267126137194431 ) ) ;
#18535=CARTESIAN_POINT ( 'NONE',  ( 60.28867513459481842, 139.2280666364260071, -4.041636747397287284E-15 ) ) ;
#18536=CARTESIAN_POINT ( 'NONE',  ( 41.92499999726881299, 164.1591823560292198, 12.60653300113718167 ) ) ;
#18543=CARTESIAN_POINT ( 'NONE',  ( 82.49999999453764588, 170.2462022514548323, -7.872454543227099337E-15 ) ) ;
#18548=ORIENTED_EDGE ( 'NONE', *, *, #1464, .F. ) ;
#18553=ADVANCED_FACE ( 'NONE', ( #2135 ), #32782, .T. ) ;
#18554=CARTESIAN_POINT ( 'NONE',  ( 78.57499999726881867, 145.8408176439707802, 12.60653300113718345 ) ) ;
#18556=CARTESIAN_POINT ( 'NONE',  ( 55.88867513459482694, 150.1262045565064227, 15.00000000000001599 ) ) ;
#18562=CARTESIAN_POINT ( 'NONE',  ( 62.87499999726880873, 138.6155565068815747, -3.929120461958505118E-15 ) ) ;
#18564=CARTESIAN_POINT ( 'NONE',  ( 62.38867513459482694, 140.7341522555726669, -4.635254915624220651 ) ) ;
#18571=CARTESIAN_POINT ( 'NONE',  ( 86.57499999726880446, 145.8408176439707802, 12.60653300113718345 ) ) ;
#18575=CARTESIAN_POINT ( 'NONE',  ( 38.32499999726881157, 145.8408176439707802, 12.60653300113718345 ) ) ;
#18580=CARTESIAN_POINT ( 'NONE',  ( 58.77499999726881441, 140.1801316387863778, 4.815267126137185549 ) ) ;
#18586=CARTESIAN_POINT ( 'NONE',  ( 60.09999999453762598, 159.7113355953771077, -14.50000000000000888 ) ) ;
#18589=CARTESIAN_POINT ( 'NONE',  ( 77.41132485994280898, 142.2402378747194405, -9.270509831248439525 ) ) ;
#18595=ORIENTED_EDGE ( 'NONE', *, *, #27010, .T. ) ;
#18603=CARTESIAN_POINT ( 'NONE',  ( 46.27499999726881441, 160.0630714827496206, 15.58253174999999224 ) ) ;
#18605=CARTESIAN_POINT ( 'NONE',  ( 47.72499999726881015, 169.8198683612136222, 4.815267126137181997 ) ) ;
#18608=VECTOR ( 'NONE', #30086, 1000.000000000000000 ) ;
#18610=CARTESIAN_POINT ( 'NONE',  ( 55.57499999726881157, 164.1591823560292198, -12.60653300113719766 ) ) ;
#18612=FACE_OUTER_BOUND ( 'NONE', #20100, .T. ) ;
#18613=CARTESIAN_POINT ( 'NONE',  ( 71.09999999999999432, 168.7903194862797420, 4.480746418436729606 ) ) ;
#18615=CARTESIAN_POINT ( 'NONE',  ( 37.98867513459482126, 146.1832212156128890, 12.13525491562421976 ) ) ;
#18618=CARTESIAN_POINT ( 'NONE',  ( 40.97499999726881725, 140.1801316387863778, -4.815267126137194431 ) ) ;
#18620=CARTESIAN_POINT ( 'NONE',  ( 76.42499999726879878, 141.7447067706911810, 9.630534252274376428 ) ) ;
#18623=CARTESIAN_POINT ( 'NONE',  ( 39.09999999453763309, 150.2886644046228639, 14.49999999999999645 ) ) ;
#18628=AXIS2_PLACEMENT_3D ( 'NONE', #18106, #25934, #2609 ) ;
#18632=ORIENTED_EDGE ( 'NONE', *, *, #23130, .T. ) ;
#18635=CYLINDRICAL_SURFACE ( 'NONE', #6713, 2.149999999999974598 ) ;
#18643=CARTESIAN_POINT ( 'NONE',  ( 34.77499999726880731, 140.1801316387863778, 4.815267126137185549 ) ) ;
#18646=EDGE_CURVE ( 'NONE', #18911, #12386, #12135, .T. ) ;
#18649=CARTESIAN_POINT ( 'NONE',  ( 56.99999999999999289, 170.2462022514548323, -7.872454543227099337E-15 ) ) ;
#18651=CARTESIAN_POINT ( 'NONE',  ( 89.50000000000001421, 155.0000000000000000, -70.00000000000000000 ) ) ;
#18652=CIRCLE ( 'NONE', #17554, 2.149999999999985256 ) ;
#18653=CARTESIAN_POINT ( 'NONE',  ( 52.32499999726881157, 145.8408176439707802, 12.60653300113718345 ) ) ;
#18655=CARTESIAN_POINT ( 'NONE',  ( 62.71132485994281325, 155.0000000000000000, 15.00000000000001243 ) ) ;
#18656=CARTESIAN_POINT ( 'NONE',  ( 62.12499999726880873, 155.0000000000000000, 15.58253174999999402 ) ) ;
#18657=CARTESIAN_POINT ( 'NONE',  ( 74.07499999726880446, 168.2552932293087906, 9.630534252274372875 ) ) ;
#18659=CARTESIAN_POINT ( 'NONE',  ( 48.91132485994280188, 146.1832212156128890, 12.13525491562421976 ) ) ;
#18672=CIRCLE ( 'NONE', #1813, 2.149999999999984812 ) ;
#18679=AXIS2_PLACEMENT_3D ( 'NONE', #25083, #27803, #19810 ) ;
#18680=CARTESIAN_POINT ( 'NONE',  ( 80.62499999726880162, 138.6155565068815747, -3.929120461958505118E-15 ) ) ;
#18681=CARTESIAN_POINT ( 'NONE',  ( 32.50000000000000000, 155.0000000000000000, -6.938893903907228378E-15 ) ) ;
#18683=CARTESIAN_POINT ( 'NONE',  ( 70.12499999726881583, 155.0000000000000000, 15.58253174999999402 ) ) ;
#18700=CARTESIAN_POINT ( 'NONE',  ( 42.02499999726880731, 160.0630714827496206, 15.58253174999999224 ) ) ;
#18701=( BOUNDED_CURVE ( )  B_SPLINE_CURVE ( 2, ( #22127, #32517, #19580, #29973, #27411, #27570, #4237, #32857, #4071, #1683, #23320 ),
 .UNSPECIFIED., .F., .T. ) 
 B_SPLINE_CURVE_WITH_KNOTS ( ( 3, 2, 2, 2, 2, 3 ),
 ( 0.1964285714285710915, 0.1999999999999996780, 0.2035714285714282368, 0.2071428571428568233, 0.2107142857142853820, 0.2142857142857139685 ),
 .UNSPECIFIED. ) 
 CURVE ( )  GEOMETRIC_REPRESENTATION_ITEM ( )  RATIONAL_B_SPLINE_CURVE ( ( 1.000000000000004219, 0.9510565162951492013, 1.000000000000000000, 0.9510565162951534202, 1.000000000000000000, 0.9510565162951534202, 1.000000000000000000, 0.9510565162951534202, 1.000000000000000000, 0.9510565162951564178, 0.9999999999999970024 ) ) 
 REPRESENTATION_ITEM ( '' )  );
#18710=CARTESIAN_POINT ( 'NONE',  ( 78.79999999453762882, 163.5228861582408797, 11.73074641843673049 ) ) ;
#18716=CARTESIAN_POINT ( 'NONE',  ( 32.50000000000000000, 155.0000000000000000, -6.938893903907228378E-15 ) ) ;
#18722=CARTESIAN_POINT ( 'NONE',  ( 76.97499999726881015, 140.1801316387863778, -4.815267126137194431 ) ) ;
#18724=CARTESIAN_POINT ( 'NONE',  ( 59.08867513459482979, 167.7597621252805880, -9.270509831248443078 ) ) ;
#18726=VECTOR ( 'NONE', #29147, 1000.000000000000000 ) ;
#18728=CARTESIAN_POINT ( 'NONE',  ( 64.87499999726881583, 138.6155565068815747, -3.929120461958505118E-15 ) ) ;
#18730=CARTESIAN_POINT ( 'NONE',  ( 36.21132485994281325, 170.7719333635740497, -7.904646289410545231E-15 ) ) ;
#18736=CARTESIAN_POINT ( 'NONE',  ( 81.97499999726881015, 169.8198683612136222, 4.815267126137181997 ) ) ;
#18739=CARTESIAN_POINT ( 'NONE',  ( 39.12499999726880873, 155.0000000000000000, -15.58253175000000823 ) ) ;
#18742=CARTESIAN_POINT ( 'NONE',  ( 82.28867513459483973, 139.2280666364260071, -4.041636747397287284E-15 ) ) ;
#18743=CARTESIAN_POINT ( 'NONE',  ( 54.47499999726880304, 149.9369285172503510, 15.58253174999999580 ) ) ;
#18752=CARTESIAN_POINT ( 'NONE',  ( 63.19999999453762740, 146.4771138417591203, 11.73074641843673227 ) ) ;
#18753=ORIENTED_EDGE ( 'NONE', *, *, #19495, .F. ) ;
#18756=DIRECTION ( 'NONE',  ( 0.000000000000000000, 0.7071067811865475727, 0.7071067811865475727 ) ) ;
#18758=CARTESIAN_POINT ( 'NONE',  ( 58.91132485994280898, 146.1832212156128890, 12.13525491562421976 ) ) ;
#18763=FACE_OUTER_BOUND ( 'NONE', #16534, .T. ) ;
#18764=CARTESIAN_POINT ( 'NONE',  ( 32.50000000000000000, 155.0000000000000000, 15.00000000000001243 ) ) ;
#18769=CARTESIAN_POINT ( 'NONE',  ( 44.17499999726881299, 164.1591823560292198, 12.60653300113718167 ) ) ;
#18771=CARTESIAN_POINT ( 'NONE',  ( 50.12499999726881583, 155.0000000000000000, 15.58253174999999402 ) ) ;
#18772=DIRECTION ( 'NONE',  ( 1.000000000000000000, 0.000000000000000000, 0.000000000000000000 ) ) ;
#18775=CARTESIAN_POINT ( 'NONE',  ( 53.17499999726881299, 145.8408176439707802, -12.60653300113719588 ) ) ;
#18777=CARTESIAN_POINT ( 'NONE',  ( 33.78867513459482552, 155.0000000000000000, 15.00000000000001243 ) ) ;
#18778=CARTESIAN_POINT ( 'NONE',  ( 75.89999999999999147, 141.2096805137202580, 4.480746418436733158 ) ) ;
#18782=DIRECTION ( 'NONE',  ( 1.000000000000000000, 0.000000000000000000, 0.000000000000000000 ) ) ;
#18783=CARTESIAN_POINT ( 'NONE',  ( 37.17499999726881299, 145.8408176439707802, -12.60653300113719588 ) ) ;
#18786=CARTESIAN_POINT ( 'NONE',  ( 77.82499999726880446, 168.2552932293087906, 9.630534252274372875 ) ) ;
#18787=VERTEX_POINT ( 'NONE', #31258 ) ;
#18788=CARTESIAN_POINT ( 'NONE',  ( 127.5000000000000000, 155.0000000000000000, 98.00000000000002842 ) ) ;
#18789=CARTESIAN_POINT ( 'NONE',  ( 43.39999999453763024, 141.2096805137202580, 4.480746418436733158 ) ) ;
#18795=FACE_OUTER_BOUND ( 'NONE', #6699, .T. ) ;
#18797=VERTEX_POINT ( 'NONE', #575 ) ;
#18800=EDGE_LOOP ( 'NONE', ( #8418, #20004, #2973, #15456 ) ) ;
#18803=CARTESIAN_POINT ( 'NONE',  ( 127.5000000000000000, 155.0000000000000000, -6.938893903907228378E-15 ) ) ;
#18806=CARTESIAN_POINT ( 'NONE',  ( 37.17499999726881299, 145.8408176439707802, -12.60653300113719588 ) ) ;
#18810=CARTESIAN_POINT ( 'NONE',  ( 56.70000000000000284, 163.5228861582408797, -11.73074641843674470 ) ) ;
#18813=CARTESIAN_POINT ( 'NONE',  ( 56.32499999726881157, 145.8408176439707802, 12.60653300113718345 ) ) ;
#18817=CARTESIAN_POINT ( 'NONE',  ( 61.72499999726881015, 169.8198683612136222, 4.815267126137181997 ) ) ;
#18818=CARTESIAN_POINT ( 'NONE',  ( 74.27499999726880731, 160.0630714827496206, 15.58253174999999402 ) ) ;
#18828=CARTESIAN_POINT ( 'NONE',  ( 127.5000000000000000, 81.56696077377658582, -76.47359838532473475 ) ) ;
#18838=CARTESIAN_POINT ( 'NONE',  ( 77.12499999726881583, 155.0000000000000000, -15.58253175000000823 ) ) ;
#18839=ORIENTED_EDGE ( 'NONE', *, *, #1445, .T. ) ;
#18843=CARTESIAN_POINT ( 'NONE',  ( 71.02499999726882152, 149.9369285172503510, -15.58253175000000823 ) ) ;
#18846=DIRECTION ( 'NONE',  ( 1.000000000000000000, 0.000000000000000000, 0.000000000000000000 ) ) ;
#18856=CARTESIAN_POINT ( 'NONE',  ( 46.42499999726881299, 141.7447067706911810, 9.630534252274376428 ) ) ;
#18863=CARTESIAN_POINT ( 'NONE',  ( 82.09999999453762598, 159.7113355953771077, -14.50000000000000888 ) ) ;
#18875=ADVANCED_FACE ( 'NONE', ( #28858 ), #18635, .F. ) ;
#18876=VERTEX_POINT ( 'NONE', #10319 ) ;
#18878=CARTESIAN_POINT ( 'NONE',  ( 77.57499999726881867, 164.1591823560292198, -12.60653300113719766 ) ) ;
#18879=CARTESIAN_POINT ( 'NONE',  ( 53.41132485994281609, 142.2402378747194405, -9.270509831248439525 ) ) ;
#18885=CARTESIAN_POINT ( 'NONE',  ( 69.17499999726881299, 145.8408176439707802, -12.60653300113719588 ) ) ;
#18887=DIRECTION ( 'NONE',  ( 1.000000000000000000, 0.000000000000000000, 0.000000000000000000 ) ) ;
#18893=CARTESIAN_POINT ( 'NONE',  ( 84.97499999726882436, 140.1801316387863778, -4.815267126137194431 ) ) ;
#18897=CARTESIAN_POINT ( 'NONE',  ( 36.92499999726880588, 145.8408176439707802, -12.60653300113719588 ) ) ;
#18898=CARTESIAN_POINT ( 'NONE',  ( 81.28867513459482552, 170.7719333635740497, -7.904646289410545231E-15 ) ) ;
#18899=DIRECTION ( 'NONE',  ( 1.000000000000000000, 0.000000000000000000, 0.000000000000000000 ) ) ;
#18902=CARTESIAN_POINT ( 'NONE',  ( 59.77499999726881441, 169.8198683612136222, -4.815267126137197984 ) ) ;
#18910=CARTESIAN_POINT ( 'NONE',  ( 58.49999999453762456, 170.2462022514548323, -7.872454543227099337E-15 ) ) ;
#18911=VERTEX_POINT ( 'NONE', #31092 ) ;
#18913=CARTESIAN_POINT ( 'NONE',  ( 77.21132485994282035, 139.2280666364260071, -4.041636747397287284E-15 ) ) ;
#18915=CARTESIAN_POINT ( 'NONE',  ( 59.21132485994281325, 139.2280666364260071, -4.041636747397287284E-15 ) ) ;
#18919=ORIENTED_EDGE ( 'NONE', *, *, #13689, .F. ) ;
#18929=CARTESIAN_POINT ( 'NONE',  ( 47.17499999726881299, 145.8408176439707802, -12.60653300113719588 ) ) ;
#18932=CARTESIAN_POINT ( 'NONE',  ( 60.22499999726881725, 149.9369285172503510, 15.58253174999999580 ) ) ;
#18937=CARTESIAN_POINT ( 'NONE',  ( 54.77499999726881441, 140.1801316387863778, 4.815267126137185549 ) ) ;
#18942=CARTESIAN_POINT ( 'NONE',  ( 72.50000000000001421, 155.0000000000000000, -14.50000000000000711 ) ) ;
#18948=CARTESIAN_POINT ( 'NONE',  ( 37.27499999726880020, 149.9369285172503510, -15.58253175000000823 ) ) ;
#18949=EDGE_CURVE ( 'NONE', #22604, #25621, #18265, .T. ) ;
#18952=CARTESIAN_POINT ( 'NONE',  ( 74.32499999726881867, 145.8408176439707802, 12.60653300113718345 ) ) ;
#18955=CARTESIAN_POINT ( 'NONE',  ( 44.09999999453762598, 159.7113355953771077, -14.50000000000000888 ) ) ;
#18958=VECTOR ( 'NONE', #20928, 1000.000000000000000 ) ;
#18967=CARTESIAN_POINT ( 'NONE',  ( 51.61132485994281893, 150.1262045565065364, -15.00000000000012434 ) ) ;
#18968=ORIENTED_EDGE ( 'NONE', *, *, #15157, .F. ) ;
#18972=AXIS2_PLACEMENT_3D ( 'NONE', #23788, #24277, #29404 ) ;
#18981=CARTESIAN_POINT ( 'NONE',  ( 87.82499999726881867, 168.2552932293087906, 9.630534252274372875 ) ) ;
#18983=EDGE_CURVE ( 'NONE', #7152, #8990, #17867, .T. ) ;
#18986=CARTESIAN_POINT ( 'NONE',  ( 53.50000000000000711, 155.0000000000000000, 14.49999999999999467 ) ) ;
#18988=CARTESIAN_POINT ( 'NONE',  ( 77.08867513459483689, 167.7597621252805880, -9.270509831248443078 ) ) ;
#18989=CARTESIAN_POINT ( 'NONE',  ( 56.22499999726881015, 149.9369285172503510, 15.58253174999999580 ) ) ;
#18992=CARTESIAN_POINT ( 'NONE',  ( 63.32499999726881867, 164.1591823560292198, -12.60653300113719766 ) ) ;
#18993=CARTESIAN_POINT ( 'NONE',  ( 73.67499999726878457, 168.2552932293087906, -9.630534252274385310 ) ) ;
#19008=EDGE_LOOP ( 'NONE', ( #17089, #11381, #29433, #21022 ) ) ;
#19010=( BOUNDED_CURVE ( )  B_SPLINE_CURVE ( 2, ( #8766, #23938, #29552, #6550, #14390, #27329, #16933, #19497, #3993, #24782, #1437 ),
 .UNSPECIFIED., .F., .T. ) 
 B_SPLINE_CURVE_WITH_KNOTS ( ( 3, 2, 2, 2, 2, 3 ),
 ( 0.6071428571428568732, 0.6107142857142854320, 0.6142857142857139907, 0.6178571428571425495, 0.6214285714285711082, 0.6249999999999996669 ),
 .UNSPECIFIED. ) 
 CURVE ( )  GEOMETRIC_REPRESENTATION_ITEM ( )  RATIONAL_B_SPLINE_CURVE ( ( 1.000000000000003109, 0.9510565162951504226, 1.000000000000000000, 0.9510565162951534202, 1.000000000000000000, 0.9510565162951534202, 1.000000000000000000, 0.9510565162951534202, 1.000000000000000000, 0.9510565162951579721, 0.9999999999999954481 ) ) 
 REPRESENTATION_ITEM ( '' )  );
#19013=CARTESIAN_POINT ( 'NONE',  ( 79.32499999726881867, 164.1591823560292198, -12.60653300113719766 ) ) ;
#19014=VERTEX_POINT ( 'NONE', #6009 ) ;
#19017=CARTESIAN_POINT ( 'NONE',  ( 69.62499999726883004, 171.3844434931184253, -7.942151717890132712E-15 ) ) ;
#19021=CARTESIAN_POINT ( 'NONE',  ( 36.50000000000000711, 155.0000000000000000, -14.50000000000000711 ) ) ;
#19029=CARTESIAN_POINT ( 'NONE',  ( 47.62499999726880162, 171.3844434931184253, -7.942151717890134290E-15 ) ) ;
#19036=CARTESIAN_POINT ( 'NONE',  ( 88.39999999453762314, 168.7903194862797420, -4.480746418436745593 ) ) ;
#19040=CARTESIAN_POINT ( 'NONE',  ( 49.28867513459483263, 170.7719333635740497, -7.904646289410545231E-15 ) ) ;
#19047=CARTESIAN_POINT ( 'NONE',  ( 76.27499999726879309, 160.0630714827496206, 15.58253174999999224 ) ) ;
#19051=DIRECTION ( 'NONE',  ( -1.000000000000000000, 0.000000000000000000, 0.000000000000000000 ) ) ;
#19053=CARTESIAN_POINT ( 'NONE',  ( 67.77499999726880731, 169.8198683612136222, -4.815267126137197984 ) ) ;
#19055=CARTESIAN_POINT ( 'NONE',  ( 36.01132485994281041, 167.7597621252805880, -9.270509831248443078 ) ) ;
#19060=CARTESIAN_POINT ( 'NONE',  ( 83.28867513459483973, 170.7719333635740497, -7.904646289410545231E-15 ) ) ;
#19062=ADVANCED_FACE ( 'NONE', ( #11639 ), #9245, .T. ) ;
#19064=CARTESIAN_POINT ( 'NONE',  ( 84.87499999726881583, 138.6155565068815463, -3.929120461958505118E-15 ) ) ;
#19066=CARTESIAN_POINT ( 'NONE',  ( 37.12499999726881583, 155.0000000000000000, -15.58253175000000823 ) ) ;
#19071=CARTESIAN_POINT ( 'NONE',  ( 64.77499999726882152, 140.1801316387863778, 4.815267126137185549 ) ) ;
#19079=CARTESIAN_POINT ( 'NONE',  ( 64.89999999453763735, 159.7113355953771077, 14.49999999999999289 ) ) ;
#19083=DIRECTION ( 'NONE',  ( 1.000000000000000000, 0.000000000000000000, 0.000000000000000000 ) ) ;
#19085=CARTESIAN_POINT ( 'NONE',  ( 71.68867513459484542, 159.8737954434933215, 15.00000000000024336 ) ) ;
#19088=VERTEX_POINT ( 'NONE', #24580 ) ;
#19089=CYLINDRICAL_SURFACE ( 'NONE', #14566, 2.149999999999974598 ) ;
#19093=EDGE_CURVE ( 'NONE', #6936, #33266, #21733, .T. ) ;
#19096=CARTESIAN_POINT ( 'NONE',  ( 48.37499999726880873, 155.0000000000000000, 15.58253174999999402 ) ) ;
#19098=CARTESIAN_POINT ( 'NONE',  ( 59.12499999726881583, 155.0000000000000000, -15.58253175000000823 ) ) ;
#19099=LINE ( 'NONE', #8537, #4468 ) ;
#19104=CARTESIAN_POINT ( 'NONE',  ( 62.27499999726880020, 160.0630714827496206, 15.58253174999999402 ) ) ;
#19106=CARTESIAN_POINT ( 'NONE',  ( 47.28867513459482552, 170.7719333635740497, -7.904646289410545231E-15 ) ) ;
#19109=CARTESIAN_POINT ( 'NONE',  ( 71.20000000000000284, 167.3344367211045096, 8.961492836873468093 ) ) ;
#19113=CARTESIAN_POINT ( 'NONE',  ( 45.47499999726881015, 160.0630714827496206, -15.58253175000000823 ) ) ;
#19115=CARTESIAN_POINT ( 'NONE',  ( 75.52499999726880731, 169.8198683612136222, -4.815267126137197984 ) ) ;
#19118=CARTESIAN_POINT ( 'NONE',  ( 47.71132485994280614, 155.0000000000000000, -15.00000000000002487 ) ) ;
#19119=CARTESIAN_POINT ( 'NONE',  ( 38.69999999453762030, 167.3344367211045096, 8.961492836873468093 ) ) ;
#19121=CARTESIAN_POINT ( 'NONE',  ( 40.11132485994280472, 169.2658477444273331, -4.635254915624224203 ) ) ;
#19122=LINE ( 'NONE', #2500, #28655 ) ;
#19131=CARTESIAN_POINT ( 'NONE',  ( 79.58867513459483689, 163.8167787843871110, 12.13525491562421621 ) ) ;
#19132=EDGE_LOOP ( 'NONE', ( #14689, #15052, #6450, #12595 ) ) ;
#19136=ORIENTED_EDGE ( 'NONE', *, *, #19519, .T. ) ;
#19137=CARTESIAN_POINT ( 'NONE',  ( 40.02499999726881441, 160.0630714827496206, 15.58253174999999402 ) ) ;
#19139=CARTESIAN_POINT ( 'NONE',  ( 39.07499999726881157, 141.7447067706911810, -9.630534252274385310 ) ) ;
#19140=CYLINDRICAL_SURFACE ( 'NONE', #14359, 2.149999999999985256 ) ;
#19142=CARTESIAN_POINT ( 'NONE',  ( 55.70000000000000284, 146.4771138417591203, 11.73074641843673227 ) ) ;
#19144=CARTESIAN_POINT ( 'NONE',  ( 77.48867513459484258, 167.7597621252805880, 9.270509831248428867 ) ) ;
#19145=( BOUNDED_CURVE ( )  B_SPLINE_CURVE ( 2, ( #6486, #16865, #17032, #1534, #30321, #27257, #32700, #9366, #3912, #11755, #19760 ),
 .UNSPECIFIED., .F., .F. ) 
 B_SPLINE_CURVE_WITH_KNOTS ( ( 3, 2, 2, 2, 2, 3 ),
 ( 0.8035714285714284921, 0.8071428571428571619, 0.8107142857142857206, 0.8142857142857142794, 0.8178571428571428381, 0.8214285714285713969 ),
 .UNSPECIFIED. ) 
 CURVE ( )  GEOMETRIC_REPRESENTATION_ITEM ( )  RATIONAL_B_SPLINE_CURVE ( ( 1.000000000000000000, 0.9510565162951534202, 1.000000000000000000, 0.9510565162951534202, 1.000000000000000000, 0.9510565162951534202, 1.000000000000000000, 0.9510565162951534202, 1.000000000000000000, 0.9510565162951534202, 1.000000000000000000 ) ) 
 REPRESENTATION_ITEM ( '' )  );
#19146=CARTESIAN_POINT ( 'NONE',  ( 55.32499999726881157, 164.1591823560292198, -12.60653300113719766 ) ) ;
#19150=CARTESIAN_POINT ( 'NONE',  ( 67.12499999726881583, 155.0000000000000000, -15.58253175000000823 ) ) ;
#19151=CARTESIAN_POINT ( 'NONE',  ( 74.57499999726881867, 145.8408176439707802, 12.60653300113718345 ) ) ;
#19153=EDGE_CURVE ( 'NONE', #30423, #5223, #33291, .T. ) ;
#19156=CARTESIAN_POINT ( 'NONE',  ( 84.08867513459485110, 142.2402378747194405, 9.270509831248432420 ) ) ;
#19162=CARTESIAN_POINT ( 'NONE',  ( 82.71132485994282035, 155.0000000000000000, 15.00000000000001243 ) ) ;
#19165=ADVANCED_FACE ( 'NONE', ( #22352 ), #10104, .F. ) ;
#19169=CARTESIAN_POINT ( 'NONE',  ( 62.81132485994281467, 150.1262045565064227, 15.00000000000001599 ) ) ;
#19175=CARTESIAN_POINT ( 'NONE',  ( 85.22499999726882436, 160.0630714827496206, -15.58253175000000823 ) ) ;
#19180=CARTESIAN_POINT ( 'NONE',  ( 69.72499999726881015, 169.8198683612136222, 4.815267126137181997 ) ) ;
#19185=CARTESIAN_POINT ( 'NONE',  ( 37.40000000000000568, 159.7113355953771077, 14.49999999999999289 ) ) ;
#19194=CARTESIAN_POINT ( 'NONE',  ( 45.32499999726881157, 164.1591823560292198, -12.60653300113719766 ) ) ;
#19201=CARTESIAN_POINT ( 'NONE',  ( 85.19999999453763451, 146.4771138417591203, 11.73074641843673227 ) ) ;
#19210=EDGE_LOOP ( 'NONE', ( #22817, #21266, #25593, #6643 ) ) ;
#19211=CARTESIAN_POINT ( 'NONE',  ( 72.97499999726881015, 140.1801316387863778, -4.815267126137194431 ) ) ;
#19213=ORIENTED_EDGE ( 'NONE', *, *, #24927, .F. ) ;
#19214=CARTESIAN_POINT ( 'NONE',  ( 77.67499999726879878, 168.2552932293087906, -9.630534252274387086 ) ) ;
#19219=SURFACE_SIDE_STYLE ('',( #24324 ) ) ;
#19222=CARTESIAN_POINT ( 'NONE',  ( 68.87499999726881583, 138.6155565068815747, -3.929120461958505118E-15 ) ) ;
#19224=CARTESIAN_POINT ( 'NONE',  ( 62.28867513459482552, 139.2280666364260071, -4.041636747397287284E-15 ) ) ;
#19232=CARTESIAN_POINT ( 'NONE',  ( 81.57499999726880446, 164.1591823560292198, -12.60653300113719766 ) ) ;
#19236=CARTESIAN_POINT ( 'NONE',  ( 42.02499999726880731, 160.0630714827496206, 15.58253174999999402 ) ) ;
#19247=CARTESIAN_POINT ( 'NONE',  ( 64.79999999453762882, 163.5228861582408797, 11.73074641843673049 ) ) ;
#19248=ORIENTED_EDGE ( 'NONE', *, *, #24979, .T. ) ;
#19253=CARTESIAN_POINT ( 'NONE',  ( 32.50000000000000000, 155.0000000000000000, -15.00000000000002487 ) ) ;
#19263=CARTESIAN_POINT ( 'NONE',  ( 32.50000000000000000, 155.0000000000000000, 15.00000000000001243 ) ) ;
#19265=CARTESIAN_POINT ( 'NONE',  ( 51.57499999726881157, 164.1591823560292198, -12.60653300113719766 ) ) ;
#19266=ORIENTED_EDGE ( 'NONE', *, *, #5380, .F. ) ;
#19267=CARTESIAN_POINT ( 'NONE',  ( 58.92499999726881299, 145.8408176439707802, -12.60653300113719588 ) ) ;
#19272=CARTESIAN_POINT ( 'NONE',  ( 57.57499999726881157, 164.1591823560292198, -12.60653300113719766 ) ) ;
#19277=CARTESIAN_POINT ( 'NONE',  ( 75.30000000000001137, 163.5228861582408797, 11.73074641843673049 ) ) ;
#19281=DIRECTION ( 'NONE',  ( 0.000000000000000000, -0.7071067811865411334, 0.7071067811865540120 ) ) ;
#19282=CARTESIAN_POINT ( 'NONE',  ( 42.07499999726881157, 168.2552932293087906, 9.630534252274372875 ) ) ;
#19284=CARTESIAN_POINT ( 'NONE',  ( 75.92499999726881299, 164.1591823560292198, 12.60653300113718167 ) ) ;
#19285=ORIENTED_EDGE ( 'NONE', *, *, #16895, .F. ) ;
#19287=CARTESIAN_POINT ( 'NONE',  ( 45.79999999453762882, 146.4771138417591203, -11.73074641843674470 ) ) ;
#19289=EDGE_CURVE ( 'NONE', #3486, #24793, #17608, .T. ) ;
#19306=EDGE_LOOP ( 'NONE', ( #17752, #6905, #10099, #28886 ) ) ;
#19307=CARTESIAN_POINT ( 'NONE',  ( 36.62499999726881583, 138.6155565068815463, -3.929120461958505118E-15 ) ) ;
#19308=EDGE_CURVE ( 'NONE', #317, #11207, #25252, .T. ) ;
#19310=CARTESIAN_POINT ( 'NONE',  ( 42.17499999726881299, 164.1591823560292198, 12.60653300113718167 ) ) ;
#19313=CARTESIAN_POINT ( 'NONE',  ( 51.79999999999999005, 142.6655632788954620, 8.961492836873471646 ) ) ;
#19319=CARTESIAN_POINT ( 'NONE',  ( 58.72499999726881015, 140.1801316387863778, -4.815267126137194431 ) ) ;
#19321=EDGE_LOOP ( 'NONE', ( #17285, #12727, #26740, #3409 ) ) ;
#19323=CARTESIAN_POINT ( 'NONE',  ( 81.87499999726880162, 171.3844434931184253, -7.942151717890132712E-15 ) ) ;
#19342=CARTESIAN_POINT ( 'NONE',  ( 82.72499999726881015, 140.1801316387863778, -4.815267126137194431 ) ) ;
#19344=VERTEX_POINT ( 'NONE', #22868 ) ;
#19345=CARTESIAN_POINT ( 'NONE',  ( 78.92499999726881299, 145.8408176439707802, -12.60653300113719588 ) ) ;
#19346=( BOUNDED_CURVE ( )  B_SPLINE_CURVE ( 2, ( #2762, #13140, #7189, #23025, #32027, #13628, #28814, #26918, #10599, #21135, #3241 ),
 .UNSPECIFIED., .F., .T. ) 
 B_SPLINE_CURVE_WITH_KNOTS ( ( 3, 2, 2, 2, 2, 3 ),
 ( 0.8928571428571427937, 0.8964285714285712414, 0.8999999999999998002, 0.9035714285714282479, 0.9071428571428569176, 0.9107142857142853654 ),
 .UNSPECIFIED. ) 
 CURVE ( )  GEOMETRIC_REPRESENTATION_ITEM ( )  RATIONAL_B_SPLINE_CURVE ( ( 1.000000000000000000, 0.9510565162951534202, 1.000000000000000000, 0.9510565162951534202, 1.000000000000000000, 0.9510565162951534202, 1.000000000000000000, 0.9510565162951534202, 1.000000000000000000, 0.9510565162951579721, 0.9999999999999954481 ) ) 
 REPRESENTATION_ITEM ( '' )  );
#19351=CARTESIAN_POINT ( 'NONE',  ( 38.10000000000000142, 141.2096805137202580, -4.480746418436742040 ) ) ;
#19354=EDGE_CURVE ( 'NONE', #23763, #29401, #30674, .T. ) ;
#19359=CARTESIAN_POINT ( 'NONE',  ( 52.42499999726880588, 141.7447067706911810, 9.630534252274376428 ) ) ;
#19367=CARTESIAN_POINT ( 'NONE',  ( 87.29999999453764303, 142.6655632788954620, 8.961492836873471646 ) ) ;
#19372=ORIENTED_EDGE ( 'NONE', *, *, #1625, .T. ) ;
#19375=CARTESIAN_POINT ( 'NONE',  ( 74.17499999726881299, 164.1591823560292198, 12.60653300113718167 ) ) ;
#19379=CARTESIAN_POINT ( 'NONE',  ( 85.97499999726882436, 169.8198683612136222, 4.815267126137181997 ) ) ;
#19386=CARTESIAN_POINT ( 'NONE',  ( 71.37499999726881583, 155.0000000000000000, -15.58253175000000823 ) ) ;
#19389=LINE ( 'NONE', #29955, #23281 ) ;
#19395=CARTESIAN_POINT ( 'NONE',  ( 66.88867513459483405, 159.8737954434938615, -14.99999999999984190 ) ) ;
#19398=CARTESIAN_POINT ( 'NONE',  ( 42.42499999726881299, 141.7447067706911810, 9.630534252274376428 ) ) ;
#19400=CARTESIAN_POINT ( 'NONE',  ( 33.92499999726881299, 164.1591823560292198, 12.60653300113718167 ) ) ;
#19402=CARTESIAN_POINT ( 'NONE',  ( 82.58867513459483689, 146.1832212156128890, -12.13525491562423042 ) ) ;
#19410=CARTESIAN_POINT ( 'NONE',  ( 69.29999999453764303, 142.6655632788954620, 8.961492836873471646 ) ) ;
#19419=ORIENTED_EDGE ( 'NONE', *, *, #1655, .F. ) ;
#19420=CARTESIAN_POINT ( 'NONE',  ( 57.88867513459482694, 150.1262045565065364, 15.00000000000011191 ) ) ;
#19425=CARTESIAN_POINT ( 'NONE',  ( 32.50000000000000000, 155.0000000000000000, -6.938893903907228378E-15 ) ) ;
#19428=CARTESIAN_POINT ( 'NONE',  ( 48.97499999726881725, 140.1801316387863778, -4.815267126137194431 ) ) ;
#19430=CARTESIAN_POINT ( 'NONE',  ( 55.22499999726880304, 160.0630714827496206, -15.58253175000000823 ) ) ;
#19435=CARTESIAN_POINT ( 'NONE',  ( 57.17499999726881299, 145.8408176439707802, -12.60653300113719588 ) ) ;
#19440=CARTESIAN_POINT ( 'NONE',  ( 82.90000000000000568, 168.7903194862797420, -4.480746418436745593 ) ) ;
#19441=CARTESIAN_POINT ( 'NONE',  ( 39.78867513459481842, 155.0000000000000000, 15.00000000000001243 ) ) ;
#19442=DIRECTION ( 'NONE',  ( 0.000000000000000000, 0.000000000000000000, -1.000000000000000000 ) ) ;
#19444=DIRECTION ( 'NONE',  ( -1.000000000000000000, 0.000000000000000000, 0.000000000000000000 ) ) ;
#19445=CARTESIAN_POINT ( 'NONE',  ( 44.87499999726880873, 138.6155565068815463, -3.929120461958505118E-15 ) ) ;
#19448=CARTESIAN_POINT ( 'NONE',  ( 84.92499999726882720, 145.8408176439707802, -12.60653300113719588 ) ) ;
#19452=CARTESIAN_POINT ( 'NONE',  ( 49.39999999453763024, 141.2096805137202580, 4.480746418436733158 ) ) ;
#19473=CARTESIAN_POINT ( 'NONE',  ( 36.02499999726881441, 160.0630714827496206, 15.58253174999999402 ) ) ;
#19475=EDGE_CURVE ( 'NONE', #24793, #3486, #206, .T. ) ;
#19478=CARTESIAN_POINT ( 'NONE',  ( 43.77499999726881441, 169.8198683612136222, -4.815267126137197984 ) ) ;
#19483=CARTESIAN_POINT ( 'NONE',  ( 63.20000000000000995, 167.3344367211045096, 8.961492836873468093 ) ) ;
#19484=CARTESIAN_POINT ( 'NONE',  ( 76.78867513459483973, 155.0000000000000000, -15.00000000000002487 ) ) ;
#19489=CARTESIAN_POINT ( 'NONE',  ( 60.02499999726880020, 160.0630714827496206, 15.58253174999999402 ) ) ;
#19491=ORIENTED_EDGE ( 'NONE', *, *, #1465, .T. ) ;
#19493=CARTESIAN_POINT ( 'NONE',  ( 83.27499999726880731, 149.9369285172503510, -15.58253175000000823 ) ) ;
#19495=EDGE_CURVE ( 'NONE', #30928, #31779, #26423, .T. ) ;
#19496=CARTESIAN_POINT ( 'NONE',  ( 55.78867513459481842, 155.0000000000000000, 15.00000000000001243 ) ) ;
#19497=CARTESIAN_POINT ( 'NONE',  ( 53.08867513459482979, 167.7597621252805880, -9.270509831248443078 ) ) ;
#19498=EDGE_CURVE ( 'NONE', #24269, #10286, #23731, .T. ) ;
#19516=CARTESIAN_POINT ( 'NONE',  ( 82.82499999726881867, 141.7447067706911810, -9.630534252274387086 ) ) ;
#19517=ORIENTED_EDGE ( 'NONE', *, *, #5641, .T. ) ;
#19519=EDGE_CURVE ( 'NONE', #5796, #7152, #455, .T. ) ;
#19520=CARTESIAN_POINT ( 'NONE',  ( 78.32499999726881867, 145.8408176439707802, 12.60653300113718345 ) ) ;
#19525=CARTESIAN_POINT ( 'NONE',  ( 35.89999999999999858, 141.2096805137202580, 4.480746418436733158 ) ) ;
#19532=CARTESIAN_POINT ( 'NONE',  ( 73.71132485994280614, 155.0000000000000000, -15.00000000000002487 ) ) ;
#19533=DIRECTION ( 'NONE',  ( 1.000000000000000000, 0.000000000000000000, 0.000000000000000000 ) ) ;
#19534=CARTESIAN_POINT ( 'NONE',  ( 53.52499999726881441, 169.8198683612136222, -4.815267126137197984 ) ) ;
#19542=CARTESIAN_POINT ( 'NONE',  ( 86.89999999453760893, 159.7113355953771077, 14.49999999999999289 ) ) ;
#19549=CARTESIAN_POINT ( 'NONE',  ( 71.67499999726881299, 168.2552932293087906, -9.630534252274385310 ) ) ;
#19554=CARTESIAN_POINT ( 'NONE',  ( 83.37499999726881583, 155.0000000000000000, -15.58253175000000823 ) ) ;
#19555=CYLINDRICAL_SURFACE ( 'NONE', #9708, 13.00000000000001776 ) ;
#19561=CARTESIAN_POINT ( 'NONE',  ( 72.17499999726881299, 164.1591823560292198, 12.60653300113718167 ) ) ;
#19572=CARTESIAN_POINT ( 'NONE',  ( 45.92499999726881299, 164.1591823560292198, 12.60653300113718167 ) ) ;
#19580=CARTESIAN_POINT ( 'NONE',  ( 76.58867513459483689, 146.1832212156128890, -12.13525491562423042 ) ) ;
#19584=CARTESIAN_POINT ( 'NONE',  ( 67.59999999453764019, 141.2096805137202580, -4.480746418436742040 ) ) ;
#19597=DIRECTION ( 'NONE',  ( -1.000000000000000000, 0.000000000000000000, 0.000000000000000000 ) ) ;
#19603=CARTESIAN_POINT ( 'NONE',  ( 51.87499999726880873, 171.3844434931184253, -7.942151717890134290E-15 ) ) ;
#19609=CARTESIAN_POINT ( 'NONE',  ( 60.97499999726881015, 140.1801316387863778, -4.815267126137194431 ) ) ;
#19615=CARTESIAN_POINT ( 'NONE',  ( 78.79999999999999716, 167.3344367211045096, -8.961492836873482304 ) ) ;
#19619=DIRECTION ( 'NONE',  ( 0.000000000000000000, 0.000000000000000000, 1.000000000000000000 ) ) ;
#19620=CARTESIAN_POINT ( 'NONE',  ( 45.17499999726881299, 145.8408176439707802, -12.60653300113719588 ) ) ;
#19622=CARTESIAN_POINT ( 'NONE',  ( 81.42499999726882720, 168.2552932293087906, -9.630534252274385310 ) ) ;
#19625=CARTESIAN_POINT ( 'NONE',  ( 47.99999999453762456, 155.0000000000000000, -14.50000000000000711 ) ) ;
#19628=CARTESIAN_POINT ( 'NONE',  ( 61.01132485994282462, 142.2402378747194405, 9.270509831248432420 ) ) ;
#19637=CARTESIAN_POINT ( 'NONE',  ( 79.08867513459483689, 167.7597621252805880, -9.270509831248443078 ) ) ;
#19642=LINE ( 'NONE', #32580, #25188 ) ;
#19644=CARTESIAN_POINT ( 'NONE',  ( 34.07499999726880446, 168.2552932293087906, 9.630534252274372875 ) ) ;
#19646=CARTESIAN_POINT ( 'NONE',  ( 38.02499999726881441, 160.0630714827496206, 15.58253174999999402 ) ) ;
#19647=CARTESIAN_POINT ( 'NONE',  ( 39.58867513459482268, 163.8167787843871110, 12.13525491562421621 ) ) ;
#19650=CARTESIAN_POINT ( 'NONE',  ( 37.97499999726881015, 169.8198683612136222, 4.815267126137181997 ) ) ;
#19653=CARTESIAN_POINT ( 'NONE',  ( 59.70000000000000284, 146.4771138417591203, 11.73074641843673227 ) ) ;
#19658=CARTESIAN_POINT ( 'NONE',  ( 65.72499999726881015, 169.8198683612136222, 4.815267126137181997 ) ) ;
#19663=CARTESIAN_POINT ( 'NONE',  ( 86.07499999726880446, 168.2552932293087906, 9.630534252274372875 ) ) ;
#19665=CARTESIAN_POINT ( 'NONE',  ( 42.78867513459481842, 155.0000000000000000, -15.00000000000002487 ) ) ;
#19666=ORIENTED_EDGE ( 'NONE', *, *, #5524, .F. ) ;
#19670=DIRECTION ( 'NONE',  ( 0.000000000000000000, 0.000000000000000000, -1.000000000000000000 ) ) ;
#19674=CARTESIAN_POINT ( 'NONE',  ( 63.11132485994280472, 140.7341522555726669, 4.635254915624211769 ) ) ;
#19680=CARTESIAN_POINT ( 'NONE',  ( 86.72499999726882436, 140.1801316387863778, -4.815267126137194431 ) ) ;
#19681=VERTEX_POINT ( 'NONE', #24202 ) ;
#19682=CARTESIAN_POINT ( 'NONE',  ( 68.88867513459483405, 159.8737954434937478, -14.99999999999993072 ) ) ;
#19683=CARTESIAN_POINT ( 'NONE',  ( 73.52499999726882152, 169.8198683612136222, -4.815267126137197984 ) ) ;
#19686=CARTESIAN_POINT ( 'NONE',  ( 75.58867513459482268, 163.8167787843871110, 12.13525491562421621 ) ) ;
#19689=CARTESIAN_POINT ( 'NONE',  ( 44.40000000000000568, 150.2886644046228639, -14.50000000000000888 ) ) ;
#19692=CARTESIAN_POINT ( 'NONE',  ( 32.50000000000000000, 155.0000000000000000, 15.00000000000001243 ) ) ;
#19693=LINE ( 'NONE', #24809, #25131 ) ;
#19694=CARTESIAN_POINT ( 'NONE',  ( 49.92499999726881299, 164.1591823560292198, 12.60653300113718167 ) ) ;
#19695=CARTESIAN_POINT ( 'NONE',  ( 65.87499999726880162, 171.3844434931184253, -7.942151717890132712E-15 ) ) ;
#19697=FACE_OUTER_BOUND ( 'NONE', #20898, .T. ) ;
#19703=CARTESIAN_POINT ( 'NONE',  ( 87.49999999453764588, 139.7537977485451393, -4.138211985947621020E-15 ) ) ;
#19711=CARTESIAN_POINT ( 'NONE',  ( 69.17499999726881299, 145.8408176439707802, -12.60653300113719588 ) ) ;
#19713=CIRCLE ( 'NONE', #5038, 27.99999999999999645 ) ;
#19716=CARTESIAN_POINT ( 'NONE',  ( 84.77499999726880731, 140.1801316387863778, 4.815267126137185549 ) ) ;
#19722=ORIENTED_EDGE ( 'NONE', *, *, #27084, .F. ) ;
#19724=EDGE_CURVE ( 'NONE', #25792, #31511, #16866, .T. ) ;
#19728=CARTESIAN_POINT ( 'NONE',  ( 85.81132485994280046, 159.8737954434936057, -15.00000000000002665 ) ) ;
#19732=CARTESIAN_POINT ( 'NONE',  ( 67.68867513459483121, 159.8737954434934352, 15.00000000000015277 ) ) ;
#19737=CARTESIAN_POINT ( 'NONE',  ( 43.92499999726881299, 164.1591823560292198, 12.60653300113718167 ) ) ;
#19739=CARTESIAN_POINT ( 'NONE',  ( 87.50000000000001421, 157.3337595323334028, -15.27490146385892267 ) ) ;
#19749=CARTESIAN_POINT ( 'NONE',  ( 68.39999999453763735, 168.7903194862797420, -4.480746418436745593 ) ) ;
#19750=ORIENTED_EDGE ( 'NONE', *, *, #17637, .F. ) ;
#19753=EDGE_CURVE ( 'NONE', #19681, #9541, #14144, .T. ) ;
#19755=CARTESIAN_POINT ( 'NONE',  ( 45.21132485994280614, 139.2280666364260071, -4.041636747397287284E-15 ) ) ;
#19760=CARTESIAN_POINT ( 'NONE',  ( 41.78867513459481842, 155.0000000000000000, 15.00000000000001243 ) ) ;
#19762=VERTEX_POINT ( 'NONE', #16193 ) ;
#19769=CARTESIAN_POINT ( 'NONE',  ( 59.67499999726880588, 168.2552932293087906, -9.630534252274387086 ) ) ;
#19775=CARTESIAN_POINT ( 'NONE',  ( 57.97499999726881015, 169.8198683612136222, 4.815267126137181997 ) ) ;
#19782=CARTESIAN_POINT ( 'NONE',  ( 77.40000000000000568, 159.7113355953771077, 14.49999999999999289 ) ) ;
#19787=CARTESIAN_POINT ( 'NONE',  ( 43.87499999726880162, 171.3844434931184253, -7.942151717890132712E-15 ) ) ;
#19791=CARTESIAN_POINT ( 'NONE',  ( 86.42499999726881299, 141.7447067706911810, 9.630534252274376428 ) ) ;
#19794=VECTOR ( 'NONE', #30692, 1000.000000000000000 ) ;
#19795=CARTESIAN_POINT ( 'NONE',  ( 49.69999999453763451, 142.6655632788954620, -8.961492836873480528 ) ) ;
#19800=DIRECTION ( 'NONE',  ( 1.000000000000000000, 0.000000000000000000, 0.000000000000000000 ) ) ;
#19801=DIRECTION ( 'NONE',  ( 0.000000000000000000, 0.000000000000000000, -1.000000000000000000 ) ) ;
#19807=CARTESIAN_POINT ( 'NONE',  ( 117.5000000000000142, 155.0000000000000000, -6.938893903907228378E-15 ) ) ;
#19810=DIRECTION ( 'NONE',  ( 0.000000000000000000, 0.000000000000000000, -1.000000000000000000 ) ) ;
#19814=CARTESIAN_POINT ( 'NONE',  ( 38.32499999726881157, 145.8408176439707802, 12.60653300113718345 ) ) ;
#19818=CARTESIAN_POINT ( 'NONE',  ( 41.97499999726881015, 169.8198683612136222, 4.815267126137181997 ) ) ;
#19822=CARTESIAN_POINT ( 'NONE',  ( 59.59999999999999432, 150.2886644046228639, 14.49999999999999645 ) ) ;
#19828=CARTESIAN_POINT ( 'NONE',  ( 65.02499999726882152, 149.9369285172503510, -15.58253175000000823 ) ) ;
#19832=CARTESIAN_POINT ( 'NONE',  ( 80.77499999726880731, 140.1801316387863778, 4.815267126137185549 ) ) ;
#19834=CARTESIAN_POINT ( 'NONE',  ( 87.50000000000001421, 155.0000000000000000, -6.938893903907228378E-15 ) ) ;
#19835=EDGE_LOOP ( 'NONE', ( #2099, #31175, #4837, #21392 ) ) ;
#19841=CARTESIAN_POINT ( 'NONE',  ( 65.98867513459482836, 146.1832212156128890, 12.13525491562421976 ) ) ;
#19848=CARTESIAN_POINT ( 'NONE',  ( 82.02499999726879309, 160.0630714827496206, 15.58253174999999224 ) ) ;
#19849=VERTEX_POINT ( 'NONE', #26750 ) ;
#19851=CARTESIAN_POINT ( 'NONE',  ( 75.52499999726880731, 169.8198683612136222, -4.815267126137197984 ) ) ;
#19855=CARTESIAN_POINT ( 'NONE',  ( 39.30000000000000426, 163.5228861582408797, 11.73074641843673049 ) ) ;
#19860=CARTESIAN_POINT ( 'NONE',  ( 53.72499999726881015, 169.8198683612136222, 4.815267126137181997 ) ) ;
#19861=CARTESIAN_POINT ( 'NONE',  ( 66.87499999726880162, 138.6155565068815463, -3.929120461958505118E-15 ) ) ;
#19863=DIRECTION ( 'NONE',  ( 0.000000000000000000, 0.000000000000000000, -1.000000000000000000 ) ) ;
#19879=CARTESIAN_POINT ( 'NONE',  ( 72.37499999726881583, 155.0000000000000000, 15.58253174999999402 ) ) ;
#19882=CARTESIAN_POINT ( 'NONE',  ( 82.67499999726881299, 141.7447067706911810, 9.630534252274376428 ) ) ;
#19884=DIRECTION ( 'NONE',  ( -1.000000000000000000, 0.000000000000000000, -0.000000000000000000 ) ) ;
#19885=DIRECTION ( 'NONE',  ( -1.000000000000000000, 0.000000000000000000, -0.000000000000000000 ) ) ;
#19899=CARTESIAN_POINT ( 'NONE',  ( 44.22499999726880304, 149.9369285172503510, 15.58253174999999580 ) ) ;
#19901=CARTESIAN_POINT ( 'NONE',  ( 87.50000000000002842, 145.7452232778646817, -11.80462230752951136 ) ) ;
#19911=CARTESIAN_POINT ( 'NONE',  ( 71.89999999453765156, 150.2886644046228639, -14.50000000000000888 ) ) ;
#19916=VECTOR ( 'NONE', #30443, 1000.000000000000000 ) ;
#19929=CARTESIAN_POINT ( 'NONE',  ( 85.41132485994282320, 142.2402378747194405, -9.270509831248439525 ) ) ;
#19931=CARTESIAN_POINT ( 'NONE',  ( 55.17499999726881299, 145.8408176439707802, -12.60653300113719588 ) ) ;
#19934=CARTESIAN_POINT ( 'NONE',  ( 32.50000000000000000, 155.0000000000000000, 15.00000000000001243 ) ) ;
#19936=CARTESIAN_POINT ( 'NONE',  ( 56.81132485994281467, 150.1262045565064227, 15.00000000000001599 ) ) ;
#19939=CARTESIAN_POINT ( 'NONE',  ( 64.27499999726880731, 160.0630714827496206, 15.58253174999999402 ) ) ;
#19945=CARTESIAN_POINT ( 'NONE',  ( 82.40000000000000568, 150.2886644046228639, -14.50000000000000888 ) ) ;
#19950=CARTESIAN_POINT ( 'NONE',  ( 49.57499999726881157, 164.1591823560292198, -12.60653300113719766 ) ) ;
#19954=CARTESIAN_POINT ( 'NONE',  ( 82.92499999726882720, 145.8408176439707802, -12.60653300113719588 ) ) ;
#19957=CARTESIAN_POINT ( 'NONE',  ( 50.59999999453762598, 168.7903194862797420, 4.480746418436729606 ) ) ;
#19962=CARTESIAN_POINT ( 'NONE',  ( 65.81132485994281467, 159.8737954434934920, -15.00000000000012434 ) ) ;
#19966=ADVANCED_FACE ( 'NONE', ( #17034 ), #12095, .T. ) ;
#19968=CARTESIAN_POINT ( 'NONE',  ( 125.5000000000000000, 261.0000000000000000, 0.000000000000000000 ) ) ;
#19974=CARTESIAN_POINT ( 'NONE',  ( 37.67499999726881299, 168.2552932293087906, -9.630534252274387086 ) ) ;
#19977=CARTESIAN_POINT ( 'NONE',  ( 47.42499999726879878, 168.2552932293087906, -9.630534252274385310 ) ) ;
#19979=CARTESIAN_POINT ( 'NONE',  ( 54.31132485994280756, 169.2658477444273331, 4.635254915624208216 ) ) ;
#19982=CARTESIAN_POINT ( 'NONE',  ( 45.17499999726881299, 145.8408176439707802, -12.60653300113719588 ) ) ;
#19986=CARTESIAN_POINT ( 'NONE',  ( 61.90000000000000568, 141.2096805137202580, 4.480746418436733158 ) ) ;
#19991=DIRECTION ( 'NONE',  ( 0.000000000000000000, 0.000000000000000000, -1.000000000000000000 ) ) ;
#19994=CARTESIAN_POINT ( 'NONE',  ( 61.52499999726881441, 169.8198683612136222, -4.815267126137197984 ) ) ;
#19997=ORIENTED_EDGE ( 'NONE', *, *, #1615, .F. ) ;
#19999=CARTESIAN_POINT ( 'NONE',  ( 42.81132485994281467, 150.1262045565064511, 15.00000000000004086 ) ) ;
#20000=CARTESIAN_POINT ( 'NONE',  ( 84.47499999726881015, 149.9369285172503510, 15.58253174999999580 ) ) ;
#20004=ORIENTED_EDGE ( 'NONE', *, *, #21426, .T. ) ;
#20013=EDGE_LOOP ( 'NONE', ( #14648, #1620, #26070, #12012 ) ) ;
#20021=ORIENTED_EDGE ( 'NONE', *, *, #25595, .F. ) ;
#20023=CARTESIAN_POINT ( 'NONE',  ( 74.22499999726881015, 149.9369285172503510, 15.58253174999999580 ) ) ;
#20026=CARTESIAN_POINT ( 'NONE',  ( 87.50000000000002842, 169.3860439379083402, -5.988074444788474615 ) ) ;
#20029=CARTESIAN_POINT ( 'NONE',  ( 41.00000000000000711, 170.2462022514548323, -7.872454543227099337E-15 ) ) ;
#20034=CARTESIAN_POINT ( 'NONE',  ( 48.62499999726880162, 138.6155565068815747, -3.929120461958505118E-15 ) ) ;
#20035=CARTESIAN_POINT ( 'NONE',  ( 60.97499999726881015, 140.1801316387863778, -4.815267126137194431 ) ) ;
#20037=CYLINDRICAL_SURFACE ( 'NONE', #32538, 15.00000000000001776 ) ;
#20041=VECTOR ( 'NONE', #28406, 1000.000000000000000 ) ;
#20046=CARTESIAN_POINT ( 'NONE',  ( 74.78867513459483973, 155.0000000000000000, -15.00000000000002487 ) ) ;
#20052=ORIENTED_EDGE ( 'NONE', *, *, #21018, .T. ) ;
#20053=CARTESIAN_POINT ( 'NONE',  ( 79.27499999726880731, 149.9369285172503510, -15.58253175000000823 ) ) ;
#20055=ORIENTED_EDGE ( 'NONE', *, *, #26661, .F. ) ;
#20056=CARTESIAN_POINT ( 'NONE',  ( 82.97499999726881015, 140.1801316387863778, -4.815267126137194431 ) ) ;
#20060=CARTESIAN_POINT ( 'NONE',  ( 57.62499999726880873, 171.3844434931184253, -7.942151717890132712E-15 ) ) ;
#20069=CARTESIAN_POINT ( 'NONE',  ( 125.5000000000000000, 231.4735983853249763, -73.43303922622312996 ) ) ;
#20077=CARTESIAN_POINT ( 'NONE',  ( 52.82499999726880446, 141.7447067706911810, -9.630534252274385310 ) ) ;
#20079=CARTESIAN_POINT ( 'NONE',  ( 87.50000000000000000, 153.3135855332814401, -15.21687184359932132 ) ) ;
#20085=CARTESIAN_POINT ( 'NONE',  ( 54.38867513459481984, 140.7341522555726669, -4.635254915624220651 ) ) ;
#20088=CARTESIAN_POINT ( 'NONE',  ( 73.89999999453763735, 150.2886644046228639, -14.50000000000000888 ) ) ;
#20089=VERTEX_POINT ( 'NONE', #30670 ) ;
#20098=CARTESIAN_POINT ( 'NONE',  ( 57.98867513459482836, 146.1832212156128890, 12.13525491562421976 ) ) ;
#20100=EDGE_LOOP ( 'NONE', ( #22823, #21681, #10716, #19136 ) ) ;
#20101=( BOUNDED_CURVE ( )  B_SPLINE_CURVE ( 2, ( #2218, #12947, #12601, #20775, #28286, #15828, #31171, #7843, #28785, #28618, #5270 ),
 .UNSPECIFIED., .F., .F. ) 
 B_SPLINE_CURVE_WITH_KNOTS ( ( 3, 2, 2, 2, 2, 3 ),
 ( 0.8571428571428572063, 0.8607142857142858761, 0.8642857142857144348, 0.8678571428571429935, 0.8714285714285715523, 0.8750000000000001110 ),
 .UNSPECIFIED. ) 
 CURVE ( )  GEOMETRIC_REPRESENTATION_ITEM ( )  RATIONAL_B_SPLINE_CURVE ( ( 0.9999999999999984457, 0.9510565162951549745, 1.000000000000000000, 0.9510565162951534202, 1.000000000000000000, 0.9510565162951534202, 1.000000000000000000, 0.9510565162951534202, 1.000000000000000000, 0.9510565162951518658, 1.000000000000001554 ) ) 
 REPRESENTATION_ITEM ( '' )  );
#20103=CYLINDRICAL_SURFACE ( 'NONE', #30307, 98.00000000000000000 ) ;
#20106=CARTESIAN_POINT ( 'NONE',  ( 58.77499999726881441, 140.1801316387863778, 4.815267126137185549 ) ) ;
#20109=LINE ( 'NONE', #32541, #5277 ) ;
#20113=CARTESIAN_POINT ( 'NONE',  ( 64.67499999726878457, 141.7447067706911810, 9.630534252274376428 ) ) ;
#20115=DIRECTION ( 'NONE',  ( -1.000000000000000000, 0.000000000000000000, 0.000000000000000000 ) ) ;
#20118=CARTESIAN_POINT ( 'NONE',  ( 81.69999999999998863, 146.4771138417591203, 11.73074641843673227 ) ) ;
#20121=DIRECTION ( 'NONE',  ( -1.000000000000000000, -0.000000000000000000, -0.000000000000000000 ) ) ;
#20122=CARTESIAN_POINT ( 'NONE',  ( 52.07499999726881157, 168.2552932293087906, 9.630534252274372875 ) ) ;
#20124=CARTESIAN_POINT ( 'NONE',  ( 83.52499999726880731, 169.8198683612136222, -4.815267126137197984 ) ) ;
#20125=CARTESIAN_POINT ( 'NONE',  ( 42.41132485994280898, 167.7597621252805880, 9.270509831248428867 ) ) ;
#20127=CARTESIAN_POINT ( 'NONE',  ( 53.99999999453762456, 155.0000000000000000, -14.50000000000000711 ) ) ;
#20132=CARTESIAN_POINT ( 'NONE',  ( 32.50000000000000000, 155.0000000000000000, -15.00000000000002487 ) ) ;
#20136=ADVANCED_FACE ( 'NONE', ( #23339 ), #5439, .T. ) ;
#20142=EDGE_CURVE ( 'NONE', #10102, #15361, #31978, .T. ) ;
#20145=CARTESIAN_POINT ( 'NONE',  ( 34.87499999726881583, 138.6155565068815747, -3.929120461958505118E-15 ) ) ;
#20147=CARTESIAN_POINT ( 'NONE',  ( 41.42499999726881299, 168.2552932293087906, -9.630534252274385310 ) ) ;
#20148=CARTESIAN_POINT ( 'NONE',  ( 53.91132485994280898, 163.8167787843871110, -12.13525491562423397 ) ) ;
#20150=CARTESIAN_POINT ( 'NONE',  ( 45.37499999726880873, 155.0000000000000000, -15.58253175000000823 ) ) ;
#20153=CARTESIAN_POINT ( 'NONE',  ( 53.71132485994279904, 155.0000000000000000, -15.00000000000002487 ) ) ;
#20155=CARTESIAN_POINT ( 'NONE',  ( 58.99999999999999289, 170.2462022514548323, -7.872454543227099337E-15 ) ) ;
#20161=DIRECTION ( 'NONE',  ( 0.000000000000000000, 0.000000000000000000, -1.000000000000000000 ) ) ;
#20163=CARTESIAN_POINT ( 'NONE',  ( 61.02499999726880020, 149.9369285172503510, -15.58253175000000823 ) ) ;
#20167=CARTESIAN_POINT ( 'NONE',  ( 87.97499999726882436, 169.8198683612136222, 4.815267126137181997 ) ) ;
#20169=EDGE_CURVE ( 'NONE', #2726, #12310, #21441, .T. ) ;
#20188=CARTESIAN_POINT ( 'NONE',  ( 72.77499999726882152, 140.1801316387863778, 4.815267126137185549 ) ) ;
#20189=CARTESIAN_POINT ( 'NONE',  ( 80.52499999726880731, 140.1801316387863778, 4.815267126137185549 ) ) ;
#20194=CARTESIAN_POINT ( 'NONE',  ( 39.00000000000000000, 170.2462022514548323, -7.872454543227099337E-15 ) ) ;
#20199=CARTESIAN_POINT ( 'NONE',  ( 78.18867513459481700, 140.7341522555726669, 4.635254915624211769 ) ) ;
#20201=CARTESIAN_POINT ( 'NONE',  ( 60.42499999726881299, 141.7447067706911810, 9.630534252274376428 ) ) ;
#20202=CARTESIAN_POINT ( 'NONE',  ( 66.17499999726881299, 164.1591823560292198, 12.60653300113718167 ) ) ;
#20221=CARTESIAN_POINT ( 'NONE',  ( 79.57499999726881867, 164.1591823560292198, -12.60653300113719766 ) ) ;
#20224=CARTESIAN_POINT ( 'NONE',  ( 73.72499999726881015, 169.8198683612136222, 4.815267126137181997 ) ) ;
#20228=CARTESIAN_POINT ( 'NONE',  ( 64.82499999726881867, 141.7447067706911810, -9.630534252274385310 ) ) ;
#20238=DIRECTION ( 'NONE',  ( 1.000000000000000000, 0.000000000000000000, 0.000000000000000000 ) ) ;
#20243=CARTESIAN_POINT ( 'NONE',  ( 36.02499999726881441, 160.0630714827496206, 15.58253174999999224 ) ) ;
#20246=( BOUNDED_CURVE ( )  B_SPLINE_CURVE ( 2, ( #3758, #11258, #13974, #8698, #26583, #10931, #13808, #11099, #21642, #24030, #21805 ),
 .UNSPECIFIED., .F., .T. ) 
 B_SPLINE_CURVE_WITH_KNOTS ( ( 3, 2, 2, 2, 2, 3 ),
 ( 0.2857142857142856984, 0.2892857142857143127, 0.2928571428571428714, 0.2964285714285714302, 0.2999999999999999889, 0.3035714285714285476 ),
 .UNSPECIFIED. ) 
 CURVE ( )  GEOMETRIC_REPRESENTATION_ITEM ( )  RATIONAL_B_SPLINE_CURVE ( ( 1.000000000000000000, 0.9510565162951534202, 1.000000000000000000, 0.9510565162951534202, 1.000000000000000000, 0.9510565162951534202, 1.000000000000000000, 0.9510565162951534202, 1.000000000000000000, 0.9510565162951534202, 1.000000000000000000 ) ) 
 REPRESENTATION_ITEM ( '' )  );
#20250=CARTESIAN_POINT ( 'NONE',  ( 53.88867513459484115, 150.1262045565061385, 14.99999999999982947 ) ) ;
#20253=CARTESIAN_POINT ( 'NONE',  ( 71.39999999453763735, 141.2096805137202580, 4.480746418436733158 ) ) ;
#20260=DIRECTION ( 'NONE',  ( -1.000000000000000000, 0.000000000000000000, -0.000000000000000000 ) ) ;
#20261=EDGE_LOOP ( 'NONE', ( #21059, #19750 ) ) ;
#20267=ORIENTED_EDGE ( 'NONE', *, *, #17013, .T. ) ;
#20269=CARTESIAN_POINT ( 'NONE',  ( 55.21132485994282746, 139.2280666364260071, -4.041636747397287284E-15 ) ) ;
#20271=CARTESIAN_POINT ( 'NONE',  ( 59.27499999726882152, 149.9369285172503510, -15.58253175000000823 ) ) ;
#20276=CARTESIAN_POINT ( 'NONE',  ( 125.5000000000000000, 155.0000000000000000, -112.0000000000000711 ) ) ;
#20279=CARTESIAN_POINT ( 'NONE',  ( 63.97499999726881725, 169.8198683612136222, 4.815267126137181997 ) ) ;
#20285=CARTESIAN_POINT ( 'NONE',  ( 33.12499999726880873, 155.0000000000000000, -15.58253175000000823 ) ) ;
#20290=CARTESIAN_POINT ( 'NONE',  ( 49.97499999726881725, 169.8198683612136222, 4.815267126137181997 ) ) ;
#20292=CARTESIAN_POINT ( 'NONE',  ( 87.02499999726879309, 149.9369285172503510, -15.58253175000000823 ) ) ;
#20296=CARTESIAN_POINT ( 'NONE',  ( 56.29999999453762172, 167.3344367211045096, -8.961492836873482304 ) ) ;
#20302=CARTESIAN_POINT ( 'NONE',  ( 60.41132485994281609, 167.7597621252805880, 9.270509831248428867 ) ) ;
#20303=ORIENTED_EDGE ( 'NONE', *, *, #27480, .F. ) ;
#20304=( BOUNDED_CURVE ( )  B_SPLINE_CURVE ( 2, ( #24353, #16680, #10839, #25360, #2671, #2032, #1858, #13212, #17527, #8118, #5540 ),
 .UNSPECIFIED., .F., .F. ) 
 B_SPLINE_CURVE_WITH_KNOTS ( ( 3, 2, 2, 2, 2, 3 ),
 ( 0.03571428571428574700, 0.03928571428571427104, 0.04285714285714279509, 0.04642857142857131914, 0.04999999999999984318, 0.05357142857142836723 ),
 .UNSPECIFIED. ) 
 CURVE ( )  GEOMETRIC_REPRESENTATION_ITEM ( )  RATIONAL_B_SPLINE_CURVE ( ( 0.9999999999999993339, 0.9510565162951540863, 1.000000000000000000, 0.9510565162951534202, 1.000000000000000000, 0.9510565162951534202, 1.000000000000000000, 0.9510565162951534202, 1.000000000000000000, 0.9510565162951550855, 0.9999999999999983347 ) ) 
 REPRESENTATION_ITEM ( '' )  );
#20308=ORIENTED_EDGE ( 'NONE', *, *, #28899, .F. ) ;
#20311=CARTESIAN_POINT ( 'NONE',  ( 117.5000000000000142, 155.0000000000000000, -6.938893903907228378E-15 ) ) ;
#20312=VERTEX_POINT ( 'NONE', #8173 ) ;
#20315=CARTESIAN_POINT ( 'NONE',  ( 36.17499999726880588, 164.1591823560292198, 12.60653300113718167 ) ) ;
#20317=CARTESIAN_POINT ( 'NONE',  ( 42.32499999726881157, 145.8408176439707802, 12.60653300113718345 ) ) ;
#20323=CARTESIAN_POINT ( 'NONE',  ( 49.37499999726880873, 155.0000000000000000, -15.58253175000000823 ) ) ;
#20326=CARTESIAN_POINT ( 'NONE',  ( 58.01132485994281751, 167.7597621252805880, -9.270509831248443078 ) ) ;
#20329=CARTESIAN_POINT ( 'NONE',  ( 68.70000000000001705, 163.5228861582408797, -11.73074641843674470 ) ) ;
#20335=CARTESIAN_POINT ( 'NONE',  ( 34.87499999726880873, 138.6155565068815463, -3.929120461958505118E-15 ) ) ;
#20338=CARTESIAN_POINT ( 'NONE',  ( 65.82499999726881867, 168.2552932293087906, 9.630534252274372875 ) ) ;
#20342=CARTESIAN_POINT ( 'NONE',  ( 36.29999999453763593, 167.3344367211045096, -8.961492836873482304 ) ) ;
#20362=ORIENTED_EDGE ( 'NONE', *, *, #19519, .F. ) ;
#20363=CARTESIAN_POINT ( 'NONE',  ( 34.31132485994280756, 169.2658477444273331, 4.635254915624208216 ) ) ;
#20367=CARTESIAN_POINT ( 'NONE',  ( 82.72499999726881015, 140.1801316387863778, -4.815267126137194431 ) ) ;
#20373=CARTESIAN_POINT ( 'NONE',  ( 42.50000000000000000, 155.0000000000000000, -14.50000000000000711 ) ) ;
#20380=CARTESIAN_POINT ( 'NONE',  ( 56.02499999726880731, 160.0630714827496206, 15.58253174999999224 ) ) ;
#20381=CARTESIAN_POINT ( 'NONE',  ( 72.37499999726881583, 155.0000000000000000, 15.58253174999999402 ) ) ;
#20390=DIRECTION ( 'NONE',  ( 1.000000000000000000, 0.000000000000000000, 0.000000000000000000 ) ) ;
#20397=ORIENTED_EDGE ( 'NONE', *, *, #7919, .T. ) ;
#20398=CARTESIAN_POINT ( 'NONE',  ( 79.87499999726880162, 171.3844434931184253, -7.942151717890132712E-15 ) ) ;
#20402=CARTESIAN_POINT ( 'NONE',  ( 70.82499999726881867, 141.7447067706911810, -9.630534252274387086 ) ) ;
#20405=CARTESIAN_POINT ( 'NONE',  ( 66.02499999726879309, 160.0630714827496206, 15.58253174999999402 ) ) ;
#20422=CARTESIAN_POINT ( 'NONE',  ( 36.82499999726881157, 141.7447067706911810, -9.630534252274387086 ) ) ;
#20430=CARTESIAN_POINT ( 'NONE',  ( 70.09999999453762598, 159.7113355953771077, -14.50000000000000888 ) ) ;
#20441=CARTESIAN_POINT ( 'NONE',  ( 50.78867513459482552, 155.0000000000000000, -15.00000000000002487 ) ) ;
#20444=EDGE_CURVE ( 'NONE', #12386, #18911, #23617, .T. ) ;
#20447=CARTESIAN_POINT ( 'NONE',  ( 55.27499999726881441, 149.9369285172503510, -15.58253175000000823 ) ) ;
#20454=CARTESIAN_POINT ( 'NONE',  ( 65.97499999726881015, 169.8198683612136222, 4.815267126137181997 ) ) ;
#20456=( BOUNDED_CURVE ( )  B_SPLINE_CURVE ( 2, ( #6504, #16715, #21496, #5818, #6153, #14165, #11279, #21662, #717, #1058, #3432 ),
 .UNSPECIFIED., .F., .T. ) 
 B_SPLINE_CURVE_WITH_KNOTS ( ( 3, 2, 2, 2, 2, 3 ),
 ( 0.3928571428571426827, 0.3964285714285712414, 0.3999999999999998002, 0.4035714285714283589, 0.4071428571428570287, 0.4107142857142855874 ),
 .UNSPECIFIED. ) 
 CURVE ( )  GEOMETRIC_REPRESENTATION_ITEM ( )  RATIONAL_B_SPLINE_CURVE ( ( 1.000000000000001554, 0.9510565162951518658, 1.000000000000000000, 0.9510565162951534202, 1.000000000000000000, 0.9510565162951534202, 1.000000000000000000, 0.9510565162951534202, 1.000000000000000000, 0.9510565162951549745, 0.9999999999999984457 ) ) 
 REPRESENTATION_ITEM ( '' )  );
#20460=CARTESIAN_POINT ( 'NONE',  ( 84.50000000000000000, 155.0000000000000000, -14.50000000000000711 ) ) ;
#20464=CARTESIAN_POINT ( 'NONE',  ( 63.88867513459482694, 150.1262045565063659, 14.99999999999997158 ) ) ;
#20465=CARTESIAN_POINT ( 'NONE',  ( 49.37499999726880873, 155.0000000000000000, -15.58253175000000823 ) ) ;
#20467=FACE_OUTER_BOUND ( 'NONE', #31373, .T. ) ;
#20468=CARTESIAN_POINT ( 'NONE',  ( 77.71132485994280614, 155.0000000000000000, -15.00000000000002487 ) ) ;
#20469=CARTESIAN_POINT ( 'NONE',  ( 127.5000000000000000, 155.0000000000010800, 106.0000000000000142 ) ) ;
#20470=CARTESIAN_POINT ( 'NONE',  ( 57.19999999453763451, 146.4771138417591203, 11.73074641843673227 ) ) ;
#20475=CARTESIAN_POINT ( 'NONE',  ( 60.61132485994281183, 159.8737954434935489, 15.00000000000006040 ) ) ;
#20486=CARTESIAN_POINT ( 'NONE',  ( 37.87499999726880873, 171.3844434931184253, -7.942151717890134290E-15 ) ) ;
#20488=CARTESIAN_POINT ( 'NONE',  ( 42.92499999726881299, 145.8408176439707802, -12.60653300113719588 ) ) ;
#20493=CARTESIAN_POINT ( 'NONE',  ( 44.27499999726881441, 160.0630714827496206, 15.58253174999999402 ) ) ;
#20497=EDGE_CURVE ( 'NONE', #31619, #9541, #7421, .T. ) ;
#20498=AXIS2_PLACEMENT_3D ( 'NONE', #7304, #32668, #22447 ) ;
#20499=CARTESIAN_POINT ( 'NONE',  ( 69.70000000000001705, 146.4771138417591203, 11.73074641843673227 ) ) ;
#20506=CARTESIAN_POINT ( 'NONE',  ( 73.22499999726881015, 160.0630714827496206, -15.58253175000000823 ) ) ;
#20507=ORIENTED_EDGE ( 'NONE', *, *, #8927, .T. ) ;
#20509=CARTESIAN_POINT ( 'NONE',  ( 34.89999999453762314, 159.7113355953771077, 14.49999999999999289 ) ) ;
#20511=FACE_BOUND ( 'NONE', #33116, .T. ) ;
#20525=CARTESIAN_POINT ( 'NONE',  ( 87.50000000000002842, 169.3860439379083402, -5.988074444788474615 ) ) ;
#20529=CARTESIAN_POINT ( 'NONE',  ( 82.92499999726882720, 145.8408176439707802, -12.60653300113719588 ) ) ;
#20530=DIRECTION ( 'NONE',  ( 0.000000000000000000, 0.000000000000000000, -1.000000000000000000 ) ) ;
#20535=CARTESIAN_POINT ( 'NONE',  ( 47.80000000000000426, 142.6655632788954620, 8.961492836873471646 ) ) ;
#20537=CARTESIAN_POINT ( 'NONE',  ( 38.61132485994280472, 159.8737954434936910, 14.99999999999996447 ) ) ;
#20543=CARTESIAN_POINT ( 'NONE',  ( 56.82499999726881157, 141.7447067706911810, -9.630534252274387086 ) ) ;
#20544=CARTESIAN_POINT ( 'NONE',  ( 71.37499999726881583, 155.0000000000000000, -15.58253175000000823 ) ) ;
#20546=CARTESIAN_POINT ( 'NONE',  ( 46.71132485994281325, 155.0000000000000000, 15.00000000000001243 ) ) ;
#20564=CARTESIAN_POINT ( 'NONE',  ( 77.27499999726880731, 149.9369285172503510, -15.58253175000000823 ) ) ;
#20569=CARTESIAN_POINT ( 'NONE',  ( 71.92499999726881299, 164.1591823560292198, 12.60653300113718167 ) ) ;
#20572=CARTESIAN_POINT ( 'NONE',  ( 61.52499999726881441, 169.8198683612136222, -4.815267126137197984 ) ) ;
#20576=ORIENTED_EDGE ( 'NONE', *, *, #27010, .F. ) ;
#20585=AXIS2_PLACEMENT_3D ( 'NONE', #14609, #11889, #4211 ) ;
#20592=CARTESIAN_POINT ( 'NONE',  ( 39.42499999726881299, 168.2552932293087906, -9.630534252274387086 ) ) ;
#20600=CARTESIAN_POINT ( 'NONE',  ( 70.79999999453761461, 163.5228861582408797, 11.73074641843673049 ) ) ;
#20606=CARTESIAN_POINT ( 'NONE',  ( 74.71132485994280614, 155.0000000000000000, 15.00000000000001243 ) ) ;
#20617=VERTEX_POINT ( 'NONE', #17498 ) ;
#20620=CARTESIAN_POINT ( 'NONE',  ( 60.27499999726881441, 160.0630714827496206, 15.58253174999999224 ) ) ;
#20631=CARTESIAN_POINT ( 'NONE',  ( 33.72499999726881725, 169.8198683612136222, 4.815267126137181997 ) ) ;
#20636=CARTESIAN_POINT ( 'NONE',  ( 52.17499999726880588, 164.1591823560292198, 12.60653300113718167 ) ) ;
#20640=DIRECTION ( 'NONE',  ( 0.000000000000000000, -1.000000000000000000, 1.290957005378097920E-14 ) ) ;
#20642=CARTESIAN_POINT ( 'NONE',  ( 78.41132485994280898, 167.7597621252805880, 9.270509831248428867 ) ) ;
#20644=CARTESIAN_POINT ( 'NONE',  ( 50.99999999453763166, 155.0000000000000000, 14.49999999999999467 ) ) ;
#20650=LINE ( 'NONE', #28139, #7283 ) ;
#20652=CARTESIAN_POINT ( 'NONE',  ( 60.01132485994281041, 167.7597621252805880, -9.270509831248443078 ) ) ;
#20659=CARTESIAN_POINT ( 'NONE',  ( 78.77499999726880731, 140.1801316387863778, 4.815267126137185549 ) ) ;
#20664=CARTESIAN_POINT ( 'NONE',  ( 36.57499999726881157, 145.8408176439707802, 12.60653300113718345 ) ) ;
#20666=CARTESIAN_POINT ( 'NONE',  ( 44.22499999726880304, 149.9369285172503510, 15.58253174999999580 ) ) ;
#20670=CARTESIAN_POINT ( 'NONE',  ( 46.47499999726880304, 149.9369285172503510, 15.58253174999999580 ) ) ;
#20671=CARTESIAN_POINT ( 'NONE',  ( 79.01132485994281751, 142.2402378747194405, 9.270509831248432420 ) ) ;
#20673=CARTESIAN_POINT ( 'NONE',  ( 65.00000000000000000, 170.2462022514548323, -7.872454543227099337E-15 ) ) ;
#20680=CARTESIAN_POINT ( 'NONE',  ( 67.42499999726879878, 168.2552932293087906, -9.630534252274385310 ) ) ;
#20683=CARTESIAN_POINT ( 'NONE',  ( 36.49999999453763166, 170.2462022514548323, -7.872454543227099337E-15 ) ) ;
#20691=ORIENTED_EDGE ( 'NONE', *, *, #24584, .T. ) ;
#20700=CARTESIAN_POINT ( 'NONE',  ( 82.42499999726882720, 141.7447067706911810, 9.630534252274376428 ) ) ;
#20703=DIRECTION ( 'NONE',  ( -1.000000000000000000, 0.000000000000000000, 0.000000000000000000 ) ) ;
#20704=CARTESIAN_POINT ( 'NONE',  ( 50.20000000000000284, 142.6655632788954620, -8.961492836873480528 ) ) ;
#20707=CARTESIAN_POINT ( 'NONE',  ( 52.12499999726881583, 155.0000000000000000, 15.58253174999999402 ) ) ;
#20711=CARTESIAN_POINT ( 'NONE',  ( 59.62499999726881583, 171.3844434931184253, -7.942151717890134290E-15 ) ) ;
#20712=CARTESIAN_POINT ( 'NONE',  ( 72.17499999726881299, 164.1591823560292198, 12.60653300113718167 ) ) ;
#20729=ORIENTED_EDGE ( 'NONE', *, *, #18464, .T. ) ;
#20730=CARTESIAN_POINT ( 'NONE',  ( 80.17499999726881299, 164.1591823560292198, 12.60653300113718167 ) ) ;
#20732=ORIENTED_EDGE ( 'NONE', *, *, #22599, .T. ) ;
#20733=CARTESIAN_POINT ( 'NONE',  ( 73.62499999726883004, 171.3844434931184253, -7.942151717890134290E-15 ) ) ;
#20735=DIRECTION ( 'NONE',  ( -1.000000000000000000, 0.000000000000000000, -0.000000000000000000 ) ) ;
#20737=CARTESIAN_POINT ( 'NONE',  ( 61.82499999726881157, 168.2552932293087906, 9.630534252274372875 ) ) ;
#20742=CARTESIAN_POINT ( 'NONE',  ( 127.5000000000000000, 152.8500000000011028, 106.0000000000000426 ) ) ;
#20745=CARTESIAN_POINT ( 'NONE',  ( 45.48867513459483547, 167.7597621252805880, 9.270509831248428867 ) ) ;
#20751=CARTESIAN_POINT ( 'NONE',  ( 41.32499999726881157, 164.1591823560292198, -12.60653300113719766 ) ) ;
#20760=CARTESIAN_POINT ( 'NONE',  ( 78.69999999453762030, 167.3344367211045096, 8.961492836873468093 ) ) ;
#20765=CARTESIAN_POINT ( 'NONE',  ( 63.78867513459482552, 155.0000000000000000, 15.00000000000001243 ) ) ;
#20768=ORIENTED_EDGE ( 'NONE', *, *, #28307, .T. ) ;
#20775=CARTESIAN_POINT ( 'NONE',  ( 82.01132485994281751, 167.7597621252805880, -9.270509831248443078 ) ) ;
#20777=CARTESIAN_POINT ( 'NONE',  ( 61.77499999726881441, 169.8198683612136222, -4.815267126137197984 ) ) ;
#20780=CARTESIAN_POINT ( 'NONE',  ( 32.50000000000000000, 155.0000000000000000, -6.938893903907228378E-15 ) ) ;
#20784=DIRECTION ( 'NONE',  ( -1.000000000000000000, 0.000000000000000000, 0.000000000000000000 ) ) ;
#20790=CARTESIAN_POINT ( 'NONE',  ( 35.12499999726881583, 155.0000000000000000, -15.58253175000000823 ) ) ;
#20794=CARTESIAN_POINT ( 'NONE',  ( 64.18867513459483121, 140.7341522555726669, 4.635254915624211769 ) ) ;
#20795=CARTESIAN_POINT ( 'NONE',  ( 54.37499999726881583, 155.0000000000000000, 15.58253174999999402 ) ) ;
#20796=EDGE_CURVE ( 'NONE', #20089, #2726, #2005, .T. ) ;
#20798=DIRECTION ( 'NONE',  ( 0.000000000000000000, 0.000000000000000000, -1.000000000000000000 ) ) ;
#20799=CARTESIAN_POINT ( 'NONE',  ( 42.51132485994281751, 163.8167787843871110, 12.13525491562421621 ) ) ;
#20801=CARTESIAN_POINT ( 'NONE',  ( 55.49999999453763166, 139.7537977485451393, -4.138211985947621020E-15 ) ) ;
#20811=ORIENTED_EDGE ( 'NONE', *, *, #19498, .F. ) ;
#20813=CARTESIAN_POINT ( 'NONE',  ( 44.51132485994280330, 163.8167787843871110, 12.13525491562421621 ) ) ;
#20817=EDGE_CURVE ( 'NONE', #32748, #19344, #3418, .T. ) ;
#20820=CARTESIAN_POINT ( 'NONE',  ( 41.87499999726880873, 171.3844434931184253, -7.942151717890134290E-15 ) ) ;
#20822=CARTESIAN_POINT ( 'NONE',  ( 51.72499999726881725, 169.8198683612136222, 4.815267126137181997 ) ) ;
#20826=CARTESIAN_POINT ( 'NONE',  ( 51.17499999726880588, 145.8408176439707802, -12.60653300113719588 ) ) ;
#20830=EDGE_CURVE ( 'NONE', #22913, #11543, #22440, .T. ) ;
#20831=AXIS2_PLACEMENT_3D ( 'NONE', #12798, #2241, #20798 ) ;
#20832=CARTESIAN_POINT ( 'NONE',  ( 65.60000000000000853, 150.2886644046228639, 14.49999999999999645 ) ) ;
#20836=CARTESIAN_POINT ( 'NONE',  ( 57.28867513459483263, 170.7719333635740497, -7.904646289410545231E-15 ) ) ;
#20840=CARTESIAN_POINT ( 'NONE',  ( 68.62499999726880162, 138.6155565068815463, -3.929120461958505118E-15 ) ) ;
#20842=CARTESIAN_POINT ( 'NONE',  ( 84.71132485994282035, 155.0000000000000000, 15.00000000000001243 ) ) ;
#20843=VECTOR ( 'NONE', #12169, 1000.000000000000000 ) ;
#20844=CARTESIAN_POINT ( 'NONE',  ( 37.89999999453763024, 150.2886644046228639, -14.50000000000000888 ) ) ;
#20853=CARTESIAN_POINT ( 'NONE',  ( 32.50000000000000000, 155.0000000000000000, -15.00000000000002487 ) ) ;
#20865=CARTESIAN_POINT ( 'NONE',  ( 56.01132485994281041, 167.7597621252805880, -9.270509831248443078 ) ) ;
#20870=CARTESIAN_POINT ( 'NONE',  ( 85.22499999726882436, 160.0630714827496206, -15.58253175000000823 ) ) ;
#20876=CARTESIAN_POINT ( 'NONE',  ( 46.30000000000000426, 146.4771138417591203, -11.73074641843674470 ) ) ;
#20878=CARTESIAN_POINT ( 'NONE',  ( 84.71132485994282035, 155.0000000000000000, 15.00000000000001243 ) ) ;
#20879=CARTESIAN_POINT ( 'NONE',  ( 52.02499999726880020, 160.0630714827496206, 15.58253174999999402 ) ) ;
#20883=CARTESIAN_POINT ( 'NONE',  ( 57.52499999726881441, 169.8198683612136222, -4.815267126137197984 ) ) ;
#20884=CARTESIAN_POINT ( 'NONE',  ( 73.27499999726882152, 149.9369285172503510, -15.58253175000000823 ) ) ;
#20886=CARTESIAN_POINT ( 'NONE',  ( 45.91132485994280898, 163.8167787843871110, -12.13525491562423397 ) ) ;
#20892=AXIS2_PLACEMENT_3D ( 'NONE', #22667, #25225, #1890 ) ;
#20898=EDGE_LOOP ( 'NONE', ( #14760, #12187, #11499, #12559 ) ) ;
#20905=CARTESIAN_POINT ( 'NONE',  ( 69.72499999726881015, 169.8198683612136222, 4.815267126137181997 ) ) ;
#20909=CARTESIAN_POINT ( 'NONE',  ( 64.02499999726880731, 160.0630714827496206, 15.58253174999999402 ) ) ;
#20912=VERTEX_POINT ( 'NONE', #28741 ) ;
#20926=CARTESIAN_POINT ( 'NONE',  ( 35.52499999726880731, 169.8198683612136222, -4.815267126137197984 ) ) ;
#20928=DIRECTION ( 'NONE',  ( 1.000000000000000000, 0.000000000000000000, 0.000000000000000000 ) ) ;
#20934=CARTESIAN_POINT ( 'NONE',  ( 80.19999999453763451, 163.5228861582408797, -11.73074641843674470 ) ) ;
#20941=ORIENTED_EDGE ( 'NONE', *, *, #28526, .T. ) ;
#20942=VERTEX_POINT ( 'NONE', #13232 ) ;
#20948=CARTESIAN_POINT ( 'NONE',  ( 64.17499999726879878, 164.1591823560292198, 12.60653300113718167 ) ) ;
#20949=ORIENTED_EDGE ( 'NONE', *, *, #6664, .T. ) ;
#20961=CARTESIAN_POINT ( 'NONE',  ( 83.60000000000000853, 150.2886644046228639, 14.49999999999999645 ) ) ;
#20965=CARTESIAN_POINT ( 'NONE',  ( 56.37499999726880873, 155.0000000000000000, 15.58253174999999402 ) ) ;
#20968=CYLINDRICAL_SURFACE ( 'NONE', #21906, 2.149999999999985256 ) ;
#20972=CARTESIAN_POINT ( 'NONE',  ( 59.79999999453762882, 146.4771138417591203, -11.73074641843674470 ) ) ;
#20973=VERTEX_POINT ( 'NONE', #5066 ) ;
#20977=CARTESIAN_POINT ( 'NONE',  ( 44.71132485994280614, 155.0000000000000000, 15.00000000000001243 ) ) ;
#20987=CARTESIAN_POINT ( 'NONE',  ( 44.57499999726881157, 145.8408176439707802, 12.60653300113718345 ) ) ;
#20989=CARTESIAN_POINT ( 'NONE',  ( 53.22499999726879594, 160.0630714827496206, -15.58253175000000823 ) ) ;
#20990=DIRECTION ( 'NONE',  ( 1.000000000000000000, 0.000000000000000000, 0.000000000000000000 ) ) ;
#20993=CARTESIAN_POINT ( 'NONE',  ( 52.67499999726880588, 141.7447067706911810, 9.630534252274376428 ) ) ;
#20996=CARTESIAN_POINT ( 'NONE',  ( 44.78867513459481842, 155.0000000000000000, -15.00000000000002487 ) ) ;
#20997=EDGE_CURVE ( 'NONE', #19344, #32748, #7794, .T. ) ;
#20998=CARTESIAN_POINT ( 'NONE',  ( 67.90000000000000568, 141.2096805137202580, 4.480746418436733158 ) ) ;
#21002=CARTESIAN_POINT ( 'NONE',  ( 86.28867513459482552, 139.2280666364260071, -4.041636747397287284E-15 ) ) ;
#21003=CARTESIAN_POINT ( 'NONE',  ( 37.07499999726881157, 141.7447067706911810, -9.630534252274385310 ) ) ;
#21005=CARTESIAN_POINT ( 'NONE',  ( 69.12499999726881583, 155.0000000000000000, -15.58253175000000823 ) ) ;
#21007=DIRECTION ( 'NONE',  ( 1.000000000000000000, 0.000000000000000000, 0.000000000000000000 ) ) ;
#21008=CARTESIAN_POINT ( 'NONE',  ( 40.49999999453763166, 170.2462022514548323, -7.872454543227099337E-15 ) ) ;
#21017=EDGE_LOOP ( 'NONE', ( #12989, #2438, #27104, #16094 ) ) ;
#21018=EDGE_CURVE ( 'NONE', #8859, #31412, #19642, .T. ) ;
#21022=ORIENTED_EDGE ( 'NONE', *, *, #20997, .T. ) ;
#21026=CIRCLE ( 'NONE', #6329, 2.149999999999994138 ) ;
#21029=CARTESIAN_POINT ( 'NONE',  ( 34.87499999726880873, 138.6155565068815463, -3.929120461958505118E-15 ) ) ;
#21033=CARTESIAN_POINT ( 'NONE',  ( 46.20000000000000995, 142.6655632788954620, -8.961492836873480528 ) ) ;
#21037=CARTESIAN_POINT ( 'NONE',  ( 51.82499999726881157, 168.2552932293087906, 9.630534252274372875 ) ) ;
#21041=CARTESIAN_POINT ( 'NONE',  ( 63.52499999726880731, 169.8198683612136222, -4.815267126137197984 ) ) ;
#21042=CARTESIAN_POINT ( 'NONE',  ( 66.97499999726881015, 140.1801316387863778, -4.815267126137194431 ) ) ;
#21059=ORIENTED_EDGE ( 'NONE', *, *, #2945, .F. ) ;
#21065=CARTESIAN_POINT ( 'NONE',  ( 80.32499999726880446, 145.8408176439707802, 12.60653300113718345 ) ) ;
#21068=CARTESIAN_POINT ( 'NONE',  ( 68.22499999726881015, 149.9369285172503510, 15.58253174999999580 ) ) ;
#21076=FACE_BOUND ( 'NONE', #16490, .T. ) ;
#21082=CARTESIAN_POINT ( 'NONE',  ( 45.22499999726881015, 160.0630714827496206, -15.58253175000000823 ) ) ;
#21092=CARTESIAN_POINT ( 'NONE',  ( 77.39999999453762314, 141.2096805137202580, 4.480746418436733158 ) ) ;
#21101=ORIENTED_EDGE ( 'NONE', *, *, #22599, .F. ) ;
#21103=CARTESIAN_POINT ( 'NONE',  ( 87.18867513459483121, 169.2658477444273331, -4.635254915624224203 ) ) ;
#21110=CARTESIAN_POINT ( 'NONE',  ( 64.47499999726881015, 149.9369285172503510, 15.58253174999999580 ) ) ;
#21111=ORIENTED_EDGE ( 'NONE', *, *, #28609, .T. ) ;
#21112=CARTESIAN_POINT ( 'NONE',  ( 41.08867513459482979, 167.7597621252805880, -9.270509831248443078 ) ) ;
#21113=SHAPE_REPRESENTATION_RELATIONSHIP ( 'NONE' , 'NONE' ,  #32415, #32336 ) ;
#21119=CARTESIAN_POINT ( 'NONE',  ( 86.27499999726880731, 160.0630714827496206, 15.58253174999999402 ) ) ;
#21123=CARTESIAN_POINT ( 'NONE',  ( 37.62499999726880162, 171.3844434931184253, -7.942151717890132712E-15 ) ) ;
#21127=CARTESIAN_POINT ( 'NONE',  ( 57.67499999726880588, 168.2552932293087906, -9.630534252274385310 ) ) ;
#21132=CARTESIAN_POINT ( 'NONE',  ( 63.49999999453763166, 139.7537977485451393, -4.138211985947621020E-15 ) ) ;
#21135=CARTESIAN_POINT ( 'NONE',  ( 36.88867513459483405, 159.8737954434939752, -14.99999999999974420 ) ) ;
#21145=CARTESIAN_POINT ( 'NONE',  ( 80.28867513459483973, 139.2280666364260071, -4.041636747397287284E-15 ) ) ;
#21146=ORIENTED_EDGE ( 'NONE', *, *, #25531, .T. ) ;
#21149=CARTESIAN_POINT ( 'NONE',  ( 40.67499999726880588, 141.7447067706911810, 9.630534252274376428 ) ) ;
#21151=CARTESIAN_POINT ( 'NONE',  ( 53.92499999726881299, 164.1591823560292198, 12.60653300113718167 ) ) ;
#21156=CARTESIAN_POINT ( 'NONE',  ( 54.47499999726880304, 149.9369285172503510, 15.58253174999999580 ) ) ;
#21160=CARTESIAN_POINT ( 'NONE',  ( 75.80000000000001137, 142.6655632788954620, 8.961492836873471646 ) ) ;
#21164=LINE ( 'NONE', #15722, #14016 ) ;
#21165=CARTESIAN_POINT ( 'NONE',  ( 40.57499999726881157, 145.8408176439707802, 12.60653300113718345 ) ) ;
#21168=AXIS2_PLACEMENT_3D ( 'NONE', #20469, #7018, #17402 ) ;
#21169=CARTESIAN_POINT ( 'NONE',  ( 70.82499999726883289, 141.7447067706911810, -9.630534252274385310 ) ) ;
#21172=CARTESIAN_POINT ( 'NONE',  ( 40.69999999453762030, 167.3344367211045096, 8.961492836873468093 ) ) ;
#21174=CARTESIAN_POINT ( 'NONE',  ( 39.71132485994280614, 155.0000000000000000, -15.00000000000002487 ) ) ;
#21176=EDGE_LOOP ( 'NONE', ( #2169, #5548, #33392, #5349 ) ) ;
#21185=CARTESIAN_POINT ( 'NONE',  ( 74.51132485994280330, 163.8167787843871110, 12.13525491562421621 ) ) ;
#21186=ORIENTED_EDGE ( 'NONE', *, *, #11249, .T. ) ;
#21192=ADVANCED_FACE ( 'NONE', ( #31468 ), #27142, .T. ) ;
#21193=( BOUNDED_CURVE ( )  B_SPLINE_CURVE ( 2, ( #16246, #257, #2648, #20865, #31425, #31586, #15908, #16075, #24077, #5359, #13031 ),
 .UNSPECIFIED., .F., .F. ) 
 B_SPLINE_CURVE_WITH_KNOTS ( ( 3, 2, 2, 2, 2, 3 ),
 ( 0.3928571428571428492, 0.3964285714285714080, 0.4000000000000000222, 0.4035714285714285809, 0.4071428571428571397, 0.4107142857142856984 ),
 .UNSPECIFIED. ) 
 CURVE ( )  GEOMETRIC_REPRESENTATION_ITEM ( )  RATIONAL_B_SPLINE_CURVE ( ( 1.000000000000000000, 0.9510565162951534202, 1.000000000000000000, 0.9510565162951534202, 1.000000000000000000, 0.9510565162951534202, 1.000000000000000000, 0.9510565162951534202, 1.000000000000000000, 0.9510565162951534202, 1.000000000000000000 ) ) 
 REPRESENTATION_ITEM ( '' )  );
#21194=CARTESIAN_POINT ( 'NONE',  ( 86.12499999726881583, 155.0000000000000000, 15.58253174999999402 ) ) ;
#21198=CARTESIAN_POINT ( 'NONE',  ( 47.99999999999999289, 139.7537977485451393, -4.138211985947621020E-15 ) ) ;
#21201=CARTESIAN_POINT ( 'NONE',  ( 84.21132485994282035, 170.7719333635740497, -7.904646289410545231E-15 ) ) ;
#21203=CARTESIAN_POINT ( 'NONE',  ( 51.42499999726879878, 168.2552932293087906, -9.630534252274385310 ) ) ;
#21207=CARTESIAN_POINT ( 'NONE',  ( 66.82499999726881867, 141.7447067706911810, -9.630534252274387086 ) ) ;
#21208=CARTESIAN_POINT ( 'NONE',  ( 76.07499999726879025, 168.2552932293087906, 9.630534252274372875 ) ) ;
#21211=EDGE_CURVE ( 'NONE', #11454, #5515, #30653, .T. ) ;
#21224=DIRECTION ( 'NONE',  ( 0.000000000000000000, 0.000000000000000000, -1.000000000000000000 ) ) ;
#21226=ORIENTED_EDGE ( 'NONE', *, *, #744, .F. ) ;
#21228=CARTESIAN_POINT ( 'NONE',  ( 76.62499999726880162, 138.6155565068815747, -3.929120461958505118E-15 ) ) ;
#21232=CARTESIAN_POINT ( 'NONE',  ( 67.32499999726881867, 164.1591823560292198, -12.60653300113719766 ) ) ;
#21248=CARTESIAN_POINT ( 'NONE',  ( 42.22499999726880304, 149.9369285172503510, 15.58253174999999580 ) ) ;
#21256=CARTESIAN_POINT ( 'NONE',  ( 76.79999999453762882, 163.5228861582408797, 11.73074641843673049 ) ) ;
#21260=DIRECTION ( 'NONE',  ( 1.000000000000000000, 0.000000000000000000, 0.000000000000000000 ) ) ;
#21265=ORIENTED_EDGE ( 'NONE', *, *, #30492, .T. ) ;
#21266=ORIENTED_EDGE ( 'NONE', *, *, #15216, .T. ) ;
#21267=CARTESIAN_POINT ( 'NONE',  ( 76.57499999726881867, 145.8408176439707802, 12.60653300113718345 ) ) ;
#21268=CARTESIAN_POINT ( 'NONE',  ( 87.08867513459483689, 167.7597621252805880, -9.270509831248443078 ) ) ;
#21269=CARTESIAN_POINT ( 'NONE',  ( 59.78867513459481842, 155.0000000000000000, 15.00000000000001243 ) ) ;
#21273=CARTESIAN_POINT ( 'NONE',  ( 66.07499999726881867, 168.2552932293087906, 9.630534252274372875 ) ) ;
#21275=CARTESIAN_POINT ( 'NONE',  ( 35.91132485994280898, 163.8167787843871110, -12.13525491562423397 ) ) ;
#21283=CARTESIAN_POINT ( 'NONE',  ( 87.27499999726880731, 149.9369285172503510, -15.58253175000000823 ) ) ;
#21286=CARTESIAN_POINT ( 'NONE',  ( 40.22499999726880304, 149.9369285172503510, 15.58253174999999580 ) ) ;
#21288=CYLINDRICAL_SURFACE ( 'NONE', #31611, 15.00000000000001776 ) ;
#21291=CARTESIAN_POINT ( 'NONE',  ( 57.57499999726881157, 164.1591823560292198, -12.60653300113719766 ) ) ;
#21294=DIRECTION ( 'NONE',  ( -1.000000000000000000, 0.000000000000000000, 0.000000000000000000 ) ) ;
#21297=CARTESIAN_POINT ( 'NONE',  ( 60.39999999453763024, 168.7903194862797420, -4.480746418436745593 ) ) ;
#21302=CARTESIAN_POINT ( 'NONE',  ( 71.38867513459481984, 169.2658477444273331, 4.635254915624208216 ) ) ;
#21313=CARTESIAN_POINT ( 'NONE',  ( 46.07499999726881157, 168.2552932293087906, 9.630534252274372875 ) ) ;
#21314=ORIENTED_EDGE ( 'NONE', *, *, #5845, .F. ) ;
#21315=CARTESIAN_POINT ( 'NONE',  ( 48.02499999726879309, 160.0630714827496206, 15.58253174999999402 ) ) ;
#21319=CARTESIAN_POINT ( 'NONE',  ( 56.37499999726880873, 155.0000000000000000, 15.58253174999999402 ) ) ;
#21321=CARTESIAN_POINT ( 'NONE',  ( 32.50000000000000000, 155.0000000000000000, 15.00000000000001243 ) ) ;
#21322=CARTESIAN_POINT ( 'NONE',  ( 73.20000000000001705, 167.3344367211045096, 8.961492836873468093 ) ) ;
#21327=CARTESIAN_POINT ( 'NONE',  ( 41.27499999726880731, 149.9369285172503510, -15.58253175000000823 ) ) ;
#21330=CARTESIAN_POINT ( 'NONE',  ( 78.12499999726883004, 155.0000000000000000, 15.58253174999999402 ) ) ;
#21333=CARTESIAN_POINT ( 'NONE',  ( 43.49999999453763166, 139.7537977485451393, -4.138211985947621020E-15 ) ) ;
#21334=( BOUNDED_SURFACE ( )  B_SPLINE_SURFACE ( 1, 2, ( 
 ( #2278, #28173, #5002, #30558, #30906, #25273, #15222, #4831, #12500, #15390, #12327, #33111, #22889, #9948, #7220, #20335, #29171, #13170, #10628, #31887, #23565, #2954, #24052, #13659, #721, #11125, #8070, #8397, #559, #11283, #26608, #7903, #16054, #21500, #5822, #29005, #8554, #21003, #18783, #18948, #388, #16217, #26443, #5332, #3436, #21667, #234, #5666, #18455, #18284, #13833, #15723, #3271, #2790, #29344, #5991, #26122, #28673, #10952, #16379, #31401, #26771, #28842, #5498, #13497, #15887, #31724, #26281, #13333, #24223, #23725, #10791, #21165, #31562, #886, #8229, #18618, #3108, #23891, #21327, #24736, #11617, #25066, #27612, #9391, #1558, #22337, #19282, #27283, #22006, #11778, #6157, #4106, #14498, #14672, #32556, #11954, #30010, #14169, #32221, #1390, #32389, #9230, #9053, #32724, #19787, #32061, #16552, #12120, #30182, #29849, #6326, #3605, #6839, #16719, #19445, #1720, #8886, #19620, #1062, #8723, #19113, #16886, #6672, #17225, #6508, #3940, #29674, #17059, #14340, #29503, #27121, #3782, #4281, #26946, #27452, #13999, #11451, #24396, #21830, #24562, #24897, #1219, #22168, #25740, #22677, #23016, #15181, #25908, #7529, #22511, #30696, #15350, #10088, #9908, #4962, #1898, #33414, #2411, #15009, #20465, #7359, #19950, #18077, #2581, #14836, #20290, #33064, #32898, #28473, #30349, #30865, #17398, #17915, #12796, #7012, #9558, #25574, #23187, #27784, #28306, #12285, #9734, #28127, #4448, #12622, #25235, #20122, #20636, #7181, #30516, #25398, #17565, #33581, #27958, #4627, #10260, #2070, #12458, #2239, #22850, #15517, #5129, #31035, #7694, #33242, #17738, #4788, #26237, #26406, #20795, #18743, #29129, #29297, #13454, #16172, #10914, #28806, #13129, #16014, #13293, #23847, #2908, #13618, #679, #12967, #31196, #26733, #24015, #10747, #20965, #18247, #3232, #31359, #23685, #5949, #23522, #522, #15684, #23363, #26, #31526, #21291, #21127, #10423, #5291, #28964, #8195, #346, #31684, #26086, #5622, #2754, #3065, #18580, #8355, #5777, #190, #26562, #11081, #21462, #31844, #10588, #8508, #18902, #16339, #8028, #18413, #7862, #28636, #5462, #15848, #6111, #27861, #8679, #32640, #20035, #9640, #30435, #7095, #3565, #4364, #30259, #7267, #22588, #3394, #12028, #17476, #25140, #24985, #4533, #16508, #14747, #14926, #30088, #1804, #22416, #846, #33158, #17650, #29460, #1636, #13955, #13789, #9821, #11234, #12201, #32015, #32974, #25314, #21621, #24184, #6921, #1978, #19071, #12369, #26907, #24346, #9473, #1471, #27702, #11866, #22253, #22765, #9303, #19695, #6753, #17141, #20202, #27527, #4188, #30602, #14584, #32806, #17312, #19861, #21042, #23607, #5375, #31282, #18324, #15262, #23269, #7611, #7774, #2156, #103, #10505, #10666, #28559, #7942, #25995, #10161, #28214, #31112, #28386, #5207, #17995, #28719, #15763, #28038, #12539, #8113, #26158, #25829, #2321, #33324, #2824, #12708, #5043, #31445, #4873, #15593, #30773, #4699, #15089, #12876, #2665, #2493, #25482, #20544, #17816, #13208, #22929, #25654, #13048, #23104, #9994, #20712, #15433, #20381, #271, #7435, #33492, #30946, #33664, #10340, #18165, #23438, #20884, #24257, #927, #1102, #18993, #21709, #16421, #595, #18657, #21536, #18818, #29383, #31766, #19151, #6202, #18495, #2989, #32265, #29548, #16261, #26483, #23766, #8763, #3152, #29212, #11495, #29047, #6029, #21208, #28880, #5536, #3311, #26817, #26647, #15926, #10833, #762, #13695, #8432, #3481, #31602, #11161, #16591, #24095, #5864, #16089, #13872, #31926, #21873, #5701, #13539, #26983, #3647, #11325, #431, #8269, #14042, #23933, #10991, #32100, #24438, #26324, #13369, #21370, #8597, #1603, #12333, #27662, #8933, #17111, #1767, #30228, #30053, #25106, #22047, #19832, #22559, #1433, #6883, #27495, #6374, #4496, #22730, #1270, #6720, #9097, #19323, #14887, #16765, #17273, #3819, #4329, #12167, #27163, #29712, #11994, #32944, #14211, #14713, #32430, #19493, #14547, #24608, #32769, #11663, #29893, #7060, #27325, #6547, #9605, #16930, #4150, #20000, #30399, #24946, #17442, #3990, #27826, #25280, #11829, #1944, #22380, #14387, #24777, #22215, #32604, #9442, #9269, #19663, #28678, #7227, #7740, #28004, #10307, #2630, #30564, #33118, #25794, #23407, #9783, #18125, #22895, #9955, #5007, #4670, #23232, #13176, #20167, #31246, #17781, #17617, #25618 ),
 ( #15730, #12669, #10129, #15054, #10470, #25449, #17963, #33288, #5339, #20509, #2124, #12840, #7400, #2285, #18289, #13015, #12507, #5172, #23065, #15229, #28181, #26127, #7577, #20342, #33628, #20683, #15396, #2795, #30741, #28353, #33457, #4839, #30912, #28523, #2459, #15558, #70, #31081, #25953, #20844, #7908, #26614, #8076, #6163, #23572, #393, #16224, #19119, #8235, #31892, #26952, #18623, #3113, #21505, #8728, #23730, #241, #5828, #15892, #24228, #3441, #5671, #3276, #13504, #13663, #21008, #29349, #21172, #23897, #10797, #29178, #18461, #24058, #3611, #10633, #21675, #29011, #31406, #16060, #13339, #891, #28848, #31567, #729, #26449, #5503, #11130, #564, #16557, #29509, #11288, #26777, #13839, #10957, #18789, #21333, #8560, #26287, #5997, #16384, #2960, #18955, #32068, #31730, #8402, #14176, #17066, #14347, #24902, #27290, #14677, #1725, #14004, #32228, #27789, #25071, #11785, #22012, #19287, #4288, #32395, #24742, #7019, #24569, #1565, #16724, #24403, #1068, #32564, #11958, #22173, #11456, #6333, #30016, #9235, #3947, #22342, #27127, #6679, #12125, #19625, #1396, #11626, #32729, #27457, #17403, #1227, #9059, #22518, #32905, #9398, #29679, #3788, #9563, #19452, #29856, #30188, #19795, #6844, #17232, #6514, #14504, #4112, #21835, #27617, #8891, #19957, #30354, #16893, #25580, #20644, #17571, #15356, #18083, #30701, #25745, #12627, #1905, #33, #7868, #30521, #2245, #4632, #4453, #10429, #12291, #12801, #33070, #2417, #7700, #22684, #14842, #30872, #28480, #25240, #23193, #27964, #9742, #28312, #18252, #20127, #2587, #22856, #7186, #7364, #15015, #15522, #25405, #2076, #4968, #12464, #33247, #7536, #17743, #31203, #20801, #25914, #5135, #12974, #9913, #33419, #28134, #17923, #20296, #10266, #31041, #4794, #33587, #23370, #15189, #23022, #10093, #20470, #28971, #5784, #8201, #29304, #16345, #28641, #13136, #8687, #5956, #26413, #2916, #198, #18910, #13300, #5631, #21630, #28811, #16180, #31367, #5297, #15688, #13462, #26569, #3074, #26091, #20972, #10921, #23853, #18586, #3238, #8035, #21297, #26739, #528, #16022, #26245, #13625, #31691, #32023, #5468, #23692, #3401, #13797, #24022, #10596, #18419, #24191, #15854, #354, #11088, #685, #21468, #31852, #10754, #29136, #8361, #2759, #8517, #23529, #18752, #853, #11245, #21132, #31531, #32187, #29978, #32686, #11578, #6635, #27247, #16515, #14638, #22471, #11418, #6471, #19247, #19079, #25035, #26914, #27415, #13961, #17021, #22305, #3572, #29467, #11744, #9353, #6119, #4075, #8847, #29642, #24699, #9194, #32862, #24356, #17190, #3743, #1023, #21968, #6289, #30146, #21795, #16683, #19584, #27080, #14132, #22131, #32356, #12080, #1687, #6803, #19749, #27575, #24527, #14297, #9021, #32521, #1182, #24860, #1523, #19410, #14463, #4241, #11919, #29812, #16854, #3901, #1356, #20430, #22816, #10218, #31002, #9524, #27751, #23323, #20600, #7325, #17530, #14800, #33542, #27918, #20253, #2544, #9696, #30823, #12250, #19911, #30311, #28089, #7490, #17701, #6978, #1861, #25536, #4752, #33207, #17874, #22638, #2204, #7658, #15143, #30658, #7146, #28269, #9871, #12928, #20088, #4590, #18042, #28435, #4924, #25193, #33026, #5092, #30483, #14976, #25702, #15311, #2375, #12764, #25363, #10053, #12586, #17365, #23154, #4415, #22979, #15487, #25878, #33379, #2035, #12422, #10881, #13588, #26204, #21256, #8161, #31157, #29261, #3359, #26048, #21092, #151, #9203, #5912, #7825, #8316, #28604, #31650, #3200, #18213, #10387, #26372, #23981, #20760, #18710, #23486, #10555, #5585, #5255, #13417, #15649, #5744, #16136, #16307, #484, #643, #29096, #15810, #20934, #3032, #312, #26529, #13257, #11040, #21423, #2718, #13095, #13749, #31809, #31494, #7992, #31326, #8474, #18378, #10711, #26696, #28770, #18863, #5425, #2871, #23653, #18543, #28926, #15980, #23812, #16469, #6427, #32314, #14087, #1318, #26869, #16808, #1480, #21918, #1143, #21753, #22091, #24481, #17148, #24304, #8804, #22261, #24817, #11706, #29425, #3526, #14424, #6074, #19201, #6589, #29935, #16972, #27368, #975, #24652, #27204, #27534, #9145, #24145, #8980, #4035, #32476, #11536, #11876, #13919, #19542, #32648, #16637, #9310, #19367, #21580, #19703, #4196, #11374, #29761, #32142, #811, #30096, #31975, #6763, #19036, #11201, #8645, #29600, #6250, #3860, #27033 ) ),
 .UNSPECIFIED., .F., .F., .T. ) 
 B_SPLINE_SURFACE_WITH_KNOTS ( ( 2, 2 ),
 ( 3, 2, 2, 2, 2, 2, 2, 2, 2, 2, 2, 2, 2, 2, 2, 2, 2, 2, 2, 2, 2, 2, 2, 2, 2, 2, 2, 2, 2, 2, 2, 2, 2, 2, 2, 2, 2, 2, 2, 2, 2, 2, 2, 2, 2, 2, 2, 2, 2, 2, 2, 2, 2, 2, 2, 2, 2, 2, 2, 2, 2, 2, 2, 2, 2, 2, 2, 2, 2, 2, 2, 2, 2, 2, 2, 2, 2, 2, 2, 2, 2, 2, 2, 2, 2, 2, 2, 2, 2, 2, 2, 2, 2, 2, 2, 2, 2, 2, 2, 2, 2, 2, 2, 2, 2, 2, 2, 2, 2, 2, 2, 2, 2, 2, 2, 2, 2, 2, 2, 2, 2, 2, 2, 2, 2, 2, 2, 2, 2, 2, 2, 2, 2, 2, 2, 2, 2, 2, 2, 2, 2, 2, 2, 2, 2, 2, 2, 2, 2, 2, 2, 2, 2, 2, 2, 2, 2, 2, 2, 2, 2, 2, 2, 2, 2, 2, 2, 2, 2, 2, 2, 2, 2, 2, 2, 2, 2, 2, 2, 2, 2, 2, 2, 2, 2, 2, 2, 2, 2, 2, 2, 2, 2, 2, 2, 2, 2, 2, 2, 2, 2, 2, 2, 2, 2, 2, 2, 2, 2, 2, 2, 2, 2, 2, 2, 2, 2, 2, 2, 2, 2, 2, 2, 2, 2, 2, 2, 2, 2, 2, 2, 2, 2, 2, 2, 2, 2, 2, 2, 2, 2, 2, 2, 2, 2, 2, 2, 2, 2, 2, 2, 2, 2, 2, 2, 2, 2, 2, 2, 2, 2, 2, 2, 2, 2, 2, 2, 2, 2, 2, 2, 2, 2, 2, 2, 3 ),
 ( 0.000000000000000000, 1.000000000000000000 ),
 ( 0.000000000000000000, 0.003571428571428571317, 0.007142857142857142634, 0.01071428571428571438, 0.01428571428571428527, 0.01785714285714285615, 0.02142857142857142877, 0.02500000000000000139, 0.02857142857142857054, 0.03214285714285713969, 0.03571428571428571230, 0.03928571428571428492, 0.04285714285714285754, 0.04642857142857143016, 0.05000000000000000278, 0.05357142857142856845, 0.05714285714285714107, 0.06071428571428571369, 0.06428571428571427937, 0.06785714285714285199, 0.07142857142857142461, 0.07499999999999999722, 0.07857142857142856984, 0.08214285714285714246, 0.08571428571428571508, 0.08928571428571428770, 0.09285714285714286031, 0.09642857142857143293, 0.1000000000000000056, 0.1035714285714285782, 0.1071428571428571369, 0.1107142857142857095, 0.1142857142857142821, 0.1178571428571428548, 0.1214285714285714274, 0.1250000000000000000, 0.1285714285714285587, 0.1321428571428571452, 0.1357142857142857040, 0.1392857142857142905, 0.1428571428571428492, 0.1464285714285714357, 0.1499999999999999944, 0.1535714285714285809, 0.1571428571428571397, 0.1607142857142857262, 0.1642857142857142849, 0.1678571428571428437, 0.1714285714285714302, 0.1749999999999999889, 0.1785714285714285754, 0.1821428571428571341, 0.1857142857142857206, 0.1892857142857142794, 0.1928571428571428659, 0.1964285714285714246, 0.2000000000000000111, 0.2035714285714285698, 0.2071428571428571563, 0.2107142857142857151, 0.2142857142857142738, 0.2178571428571428603, 0.2214285714285714191, 0.2250000000000000056, 0.2285714285714285643, 0.2321428571428571508, 0.2357142857142857095, 0.2392857142857142960, 0.2428571428571428548, 0.2464285714285714413, 0.2500000000000000000, 0.2535714285714285587, 0.2571428571428571175, 0.2607142857142857317, 0.2642857142857142905, 0.2678571428571428492, 0.2714285714285714080, 0.2750000000000000222, 0.2785714285714285809, 0.2821428571428571397, 0.2857142857142856984, 0.2892857142857143127, 0.2928571428571428714, 0.2964285714285714302, 0.2999999999999999889, 0.3035714285714285476, 0.3071428571428571619, 0.3107142857142857206, 0.3142857142857142794, 0.3178571428571428381, 0.3214285714285714524, 0.3250000000000000111, 0.3285714285714285698, 0.3321428571428571286, 0.3357142857142856873, 0.3392857142857143016, 0.3428571428571428603, 0.3464285714285714191, 0.3499999999999999778, 0.3535714285714285920, 0.3571428571428571508, 0.3607142857142857095, 0.3642857142857142683, 0.3678571428571428825, 0.3714285714285714413, 0.3750000000000000000, 0.3785714285714285587, 0.3821428571428571175, 0.3857142857142857317, 0.3892857142857142905, 0.3928571428571428492, 0.3964285714285714080, 0.4000000000000000222, 0.4035714285714285809, 0.4071428571428571397, 0.4107142857142856984, 0.4142857142857143127, 0.4178571428571428714, 0.4214285714285714302, 0.4249999999999999889, 0.4285714285714285476, 0.4321428571428571619, 0.4357142857142857206, 0.4392857142857142794, 0.4428571428571428381, 0.4464285714285714524, 0.4500000000000000111, 0.4535714285714285698, 0.4571428571428571286, 0.4607142857142856873, 0.4642857142857143016, 0.4678571428571428603, 0.4714285714285714191, 0.4749999999999999778, 0.4785714285714285920, 0.4821428571428571508, 0.4857142857142857095, 0.4892857142857142683, 0.4928571428571428825, 0.4964285714285714413, 0.5000000000000000000, 0.5035714285714285587, 0.5071428571428571175, 0.5107142857142856762, 0.5142857142857142350, 0.5178571428571429047, 0.5214285714285714635, 0.5250000000000000222, 0.5285714285714285809, 0.5321428571428571397, 0.5357142857142856984, 0.5392857142857142572, 0.5428571428571428159, 0.5464285714285713746, 0.5500000000000000444, 0.5535714285714286031, 0.5571428571428571619, 0.5607142857142857206, 0.5642857142857142794, 0.5678571428571428381, 0.5714285714285713969, 0.5749999999999999556, 0.5785714285714286254, 0.5821428571428571841, 0.5857142857142857428, 0.5892857142857143016, 0.5928571428571428603, 0.5964285714285714191, 0.5999999999999999778, 0.6035714285714285365, 0.6071428571428570953, 0.6107142857142857650, 0.6142857142857143238, 0.6178571428571428825, 0.6214285714285714413, 0.6250000000000000000, 0.6285714285714285587, 0.6321428571428571175, 0.6357142857142856762, 0.6392857142857142350, 0.6428571428571429047, 0.6464285714285714635, 0.6500000000000000222, 0.6535714285714285809, 0.6571428571428571397, 0.6607142857142856984, 0.6642857142857142572, 0.6678571428571428159, 0.6714285714285713746, 0.6750000000000000444, 0.6785714285714286031, 0.6821428571428571619, 0.6857142857142857206, 0.6892857142857142794, 0.6928571428571428381, 0.6964285714285713969, 0.6999999999999999556, 0.7035714285714286254, 0.7071428571428571841, 0.7107142857142857428, 0.7142857142857143016, 0.7178571428571428603, 0.7214285714285714191, 0.7249999999999999778, 0.7285714285714285365, 0.7321428571428570953, 0.7357142857142857650, 0.7392857142857143238, 0.7428571428571428825, 0.7464285714285714413, 0.7500000000000000000, 0.7535714285714285587, 0.7571428571428571175, 0.7607142857142856762, 0.7642857142857142350, 0.7678571428571429047, 0.7714285714285714635, 0.7750000000000000222, 0.7785714285714285809, 0.7821428571428571397, 0.7857142857142856984, 0.7892857142857142572, 0.7928571428571428159, 0.7964285714285713746, 0.8000000000000000444, 0.8035714285714286031, 0.8071428571428571619, 0.8107142857142857206, 0.8142857142857142794, 0.8178571428571428381, 0.8214285714285713969, 0.8249999999999999556, 0.8285714285714286254, 0.8321428571428571841, 0.8357142857142857428, 0.8392857142857143016, 0.8428571428571428603, 0.8464285714285714191, 0.8499999999999999778, 0.8535714285714285365, 0.8571428571428570953, 0.8607142857142857650, 0.8642857142857143238, 0.8678571428571428825, 0.8714285714285714413, 0.8750000000000000000, 0.8785714285714285587, 0.8821428571428571175, 0.8857142857142856762, 0.8892857142857142350, 0.8928571428571429047, 0.8964285714285714635, 0.9000000000000000222, 0.9035714285714285809, 0.9071428571428571397, 0.9107142857142856984, 0.9142857142857142572, 0.9178571428571428159, 0.9214285714285713746, 0.9250000000000000444, 0.9285714285714286031, 0.9321428571428571619, 0.9357142857142857206, 0.9392857142857142794, 0.9428571428571428381, 0.9464285714285713969, 0.9499999999999999556, 0.9535714285714286254, 0.9571428571428571841, 0.9607142857142857428, 0.9642857142857143016, 0.9678571428571428603, 0.9714285714285714191, 0.9749999999999999778, 0.9785714285714285365, 0.9821428571428570953 ),
 .UNSPECIFIED. ) 
 GEOMETRIC_REPRESENTATION_ITEM ( )  RATIONAL_B_SPLINE_SURFACE ( (
 ( 1.000000000000000000, 0.9510565162951535312, 1.000000000000000000, 0.9510565162951535312, 1.000000000000000000, 0.9510565162951535312, 1.000000000000000000, 0.9510565162951535312, 1.000000000000000000, 0.9510565162951535312, 1.000000000000000000, 0.9510565162951535312, 1.000000000000000000, 0.9510565162951535312, 1.000000000000000000, 0.9510565162951535312, 1.000000000000000000, 0.9510565162951535312, 1.000000000000000000, 0.9510565162951535312, 1.000000000000000000, 0.9510565162951535312, 1.000000000000000000, 0.9510565162951535312, 1.000000000000000000, 0.9510565162951535312, 1.000000000000000000, 0.9510565162951535312, 1.000000000000000000, 0.9510565162951535312, 1.000000000000000000, 0.9510565162951535312, 1.000000000000000000, 0.9510565162951535312, 1.000000000000000000, 0.9510565162951535312, 1.000000000000000000, 0.9510565162951535312, 1.000000000000000000, 0.9510565162951535312, 1.000000000000000000, 0.9510565162951535312, 1.000000000000000000, 0.9510565162951535312, 1.000000000000000000, 0.9510565162951535312, 1.000000000000000000, 0.9510565162951535312, 1.000000000000000000, 0.9510565162951535312, 1.000000000000000000, 0.9510565162951535312, 1.000000000000000000, 0.9510565162951535312, 1.000000000000000000, 0.9510565162951535312, 1.000000000000000000, 0.9510565162951535312, 1.000000000000000000, 0.9510565162951535312, 1.000000000000000000, 0.9510565162951535312, 1.000000000000000000, 0.9510565162951535312, 1.000000000000000000, 0.9510565162951535312, 1.000000000000000000, 0.9510565162951535312, 1.000000000000000000, 0.9510565162951535312, 1.000000000000000000, 0.9510565162951535312, 1.000000000000000000, 0.9510565162951535312, 1.000000000000000000, 0.9510565162951535312, 1.000000000000000000, 0.9510565162951535312, 1.000000000000000000, 0.9510565162951535312, 1.000000000000000000, 0.9510565162951535312, 1.000000000000000000, 0.9510565162951535312, 1.000000000000000000, 0.9510565162951535312, 1.000000000000000000, 0.9510565162951535312, 1.000000000000000000, 0.9510565162951535312, 1.000000000000000000, 0.9510565162951535312, 1.000000000000000000, 0.9510565162951535312, 1.000000000000000000, 0.9510565162951535312, 1.000000000000000000, 0.9510565162951535312, 1.000000000000000000, 0.9510565162951535312, 1.000000000000000000, 0.9510565162951535312, 1.000000000000000000, 0.9510565162951535312, 1.000000000000000000, 0.9510565162951535312, 1.000000000000000000, 0.9510565162951535312, 1.000000000000000000, 0.9510565162951535312, 1.000000000000000000, 0.9510565162951535312, 1.000000000000000000, 0.9510565162951535312, 1.000000000000000000, 0.9510565162951535312, 1.000000000000000000, 0.9510565162951535312, 1.000000000000000000, 0.9510565162951535312, 1.000000000000000000, 0.9510565162951535312, 1.000000000000000000, 0.9510565162951535312, 1.000000000000000000, 0.9510565162951535312, 1.000000000000000000, 0.9510565162951535312, 1.000000000000000000, 0.9510565162951535312, 1.000000000000000000, 0.9510565162951535312, 1.000000000000000000, 0.9510565162951535312, 1.000000000000000000, 0.9510565162951535312, 1.000000000000000000, 0.9510565162951535312, 1.000000000000000000, 0.9510565162951535312, 1.000000000000000000, 0.9510565162951535312, 1.000000000000000000, 0.9510565162951535312, 1.000000000000000000, 0.9510565162951535312, 1.000000000000000000, 0.9510565162951535312, 1.000000000000000000, 0.9510565162951535312, 1.000000000000000000, 0.9510565162951535312, 1.000000000000000000, 0.9510565162951535312, 1.000000000000000000, 0.9510565162951535312, 1.000000000000000000, 0.9510565162951535312, 1.000000000000000000, 0.9510565162951535312, 1.000000000000000000, 0.9510565162951535312, 1.000000000000000000, 0.9510565162951535312, 1.000000000000000000, 0.9510565162951535312, 1.000000000000000000, 0.9510565162951535312, 1.000000000000000000, 0.9510565162951535312, 1.000000000000000000, 0.9510565162951535312, 1.000000000000000000, 0.9510565162951535312, 1.000000000000000000, 0.9510565162951535312, 1.000000000000000000, 0.9510565162951535312, 1.000000000000000000, 0.9510565162951535312, 1.000000000000000000, 0.9510565162951535312, 1.000000000000000000, 0.9510565162951535312, 1.000000000000000000, 0.9510565162951535312, 1.000000000000000000, 0.9510565162951535312, 1.000000000000000000, 0.9510565162951535312, 1.000000000000000000, 0.9510565162951535312, 1.000000000000000000, 0.9510565162951535312, 1.000000000000000000, 0.9510565162951535312, 1.000000000000000000, 0.9510565162951535312, 1.000000000000000000, 0.9510565162951535312, 1.000000000000000000, 0.9510565162951535312, 1.000000000000000000, 0.9510565162951535312, 1.000000000000000000, 0.9510565162951535312, 1.000000000000000000, 0.9510565162951535312, 1.000000000000000000, 0.9510565162951535312, 1.000000000000000000, 0.9510565162951535312, 1.000000000000000000, 0.9510565162951535312, 1.000000000000000000, 0.9510565162951535312, 1.000000000000000000, 0.9510565162951535312, 1.000000000000000000, 0.9510565162951535312, 1.000000000000000000, 0.9510565162951535312, 1.000000000000000000, 0.9510565162951535312, 1.000000000000000000, 0.9510565162951535312, 1.000000000000000000, 0.9510565162951535312, 1.000000000000000000, 0.9510565162951535312, 1.000000000000000000, 0.9510565162951535312, 1.000000000000000000, 0.9510565162951535312, 1.000000000000000000, 0.9510565162951535312, 1.000000000000000000, 0.9510565162951535312, 1.000000000000000000, 0.9510565162951535312, 1.000000000000000000, 0.9510565162951535312, 1.000000000000000000, 0.9510565162951535312, 1.000000000000000000, 0.9510565162951535312, 1.000000000000000000, 0.9510565162951535312, 1.000000000000000000, 0.9510565162951535312, 1.000000000000000000, 0.9510565162951535312, 1.000000000000000000, 0.9510565162951535312, 1.000000000000000000, 0.9510565162951535312, 1.000000000000000000, 0.9510565162951535312, 1.000000000000000000, 0.9510565162951535312, 1.000000000000000000, 0.9510565162951535312, 1.000000000000000000, 0.9510565162951535312, 1.000000000000000000, 0.9510565162951535312, 1.000000000000000000, 0.9510565162951535312, 1.000000000000000000, 0.9510565162951535312, 1.000000000000000000, 0.9510565162951535312, 1.000000000000000000, 0.9510565162951535312, 1.000000000000000000, 0.9510565162951535312, 1.000000000000000000, 0.9510565162951535312, 1.000000000000000000, 0.9510565162951535312, 1.000000000000000000, 0.9510565162951535312, 1.000000000000000000, 0.9510565162951535312, 1.000000000000000000, 0.9510565162951535312, 1.000000000000000000, 0.9510565162951535312, 1.000000000000000000, 0.9510565162951535312, 1.000000000000000000, 0.9510565162951535312, 1.000000000000000000, 0.9510565162951535312, 1.000000000000000000, 0.9510565162951535312, 1.000000000000000000, 0.9510565162951535312, 1.000000000000000000, 0.9510565162951535312, 1.000000000000000000, 0.9510565162951535312, 1.000000000000000000, 0.9510565162951535312, 1.000000000000000000, 0.9510565162951535312, 1.000000000000000000, 0.9510565162951535312, 1.000000000000000000, 0.9510565162951535312, 1.000000000000000000, 0.9510565162951535312, 1.000000000000000000, 0.9510565162951535312, 1.000000000000000000, 0.9510565162951535312, 1.000000000000000000, 0.9510565162951535312, 1.000000000000000000, 0.9510565162951535312, 1.000000000000000000, 0.9510565162951535312, 1.000000000000000000, 0.9510565162951535312, 1.000000000000000000, 0.9510565162951535312, 1.000000000000000000, 0.9510565162951535312, 1.000000000000000000, 0.9510565162951535312, 1.000000000000000000, 0.9510565162951535312, 1.000000000000000000, 0.9510565162951535312, 1.000000000000000000, 0.9510565162951535312, 1.000000000000000000, 0.9510565162951535312, 1.000000000000000000, 0.9510565162951535312, 1.000000000000000000, 0.9510565162951535312, 1.000000000000000000, 0.9510565162951535312, 1.000000000000000000, 0.9510565162951535312, 1.000000000000000000, 0.9510565162951535312, 1.000000000000000000, 0.9510565162951535312, 1.000000000000000000, 0.9510565162951535312, 1.000000000000000000, 0.9510565162951535312, 1.000000000000000000, 0.9510565162951535312, 1.000000000000000000, 0.9510565162951535312, 1.000000000000000000, 0.9510565162951535312, 1.000000000000000000, 0.9510565162951535312, 1.000000000000000000, 0.9510565162951535312, 1.000000000000000000, 0.9510565162951535312, 1.000000000000000000, 0.9510565162951535312, 1.000000000000000000, 0.9510565162951535312, 1.000000000000000000, 0.9510565162951535312, 1.000000000000000000, 0.9510565162951535312, 1.000000000000000000, 0.9510565162951535312, 1.000000000000000000, 0.9510565162951535312, 1.000000000000000000, 0.9510565162951535312, 1.000000000000000000, 0.9510565162951535312, 1.000000000000000000, 0.9510565162951535312, 1.000000000000000000, 0.9510565162951535312, 1.000000000000000000, 0.9510565162951535312, 1.000000000000000000, 0.9510565162951535312, 1.000000000000000000, 0.9510565162951535312, 1.000000000000000000, 0.9510565162951535312, 1.000000000000000000, 0.9510565162951535312, 1.000000000000000000, 0.9510565162951535312, 1.000000000000000000, 0.9510565162951535312, 1.000000000000000000, 0.9510565162951535312, 1.000000000000000000, 0.9510565162951535312, 1.000000000000000000, 0.9510565162951535312, 1.000000000000000000, 0.9510565162951535312, 1.000000000000000000, 0.9510565162951535312, 1.000000000000000000, 0.9510565162951535312, 1.000000000000000000, 0.9510565162951535312, 1.000000000000000000, 0.9510565162951535312, 1.000000000000000000, 0.9510565162951535312, 1.000000000000000000, 0.9510565162951535312, 1.000000000000000000, 0.9510565162951535312, 1.000000000000000000, 0.9510565162951535312, 1.000000000000000000, 0.9510565162951535312, 1.000000000000000000, 0.9510565162951535312, 1.000000000000000000, 0.9510565162951535312, 1.000000000000000000, 0.9510565162951535312, 1.000000000000000000, 0.9510565162951535312, 1.000000000000000000, 0.9510565162951535312, 1.000000000000000000, 0.9510565162951535312, 1.000000000000000000, 0.9510565162951535312, 1.000000000000000000, 0.9510565162951535312, 1.000000000000000000, 0.9510565162951535312, 1.000000000000000000, 0.9510565162951535312, 1.000000000000000000, 0.9510565162951535312, 1.000000000000000000, 0.9510565162951535312, 1.000000000000000000, 0.9510565162951535312, 1.000000000000000000, 0.9510565162951535312, 1.000000000000000000, 0.9510565162951535312, 1.000000000000000000, 0.9510565162951535312, 1.000000000000000000, 0.9510565162951535312, 1.000000000000000000, 0.9510565162951535312, 1.000000000000000000, 0.9510565162951535312, 1.000000000000000000, 0.9510565162951535312, 1.000000000000000000, 0.9510565162951535312, 1.000000000000000000, 0.9510565162951535312, 1.000000000000000000, 0.9510565162951535312, 1.000000000000000000, 0.9510565162951535312, 1.000000000000000000, 0.9510565162951535312, 1.000000000000000000, 0.9510565162951535312, 1.000000000000000000, 0.9510565162951535312, 1.000000000000000000, 0.9510565162951535312, 1.000000000000000000, 0.9510565162951535312, 1.000000000000000000, 0.9510565162951535312, 1.000000000000000000, 0.9510565162951535312, 1.000000000000000000, 0.9510565162951535312, 1.000000000000000000, 0.9510565162951535312, 1.000000000000000000, 0.9510565162951535312, 1.000000000000000000, 0.9510565162951535312, 1.000000000000000000, 0.9510565162951535312, 1.000000000000000000, 0.9510565162951535312, 1.000000000000000000, 0.9510565162951535312, 1.000000000000000000, 0.9510565162951535312, 1.000000000000000000, 0.9510565162951535312, 1.000000000000000000, 0.9510565162951535312, 1.000000000000000000, 0.9510565162951535312, 1.000000000000000000, 0.9510565162951535312, 1.000000000000000000, 0.9510565162951535312, 1.000000000000000000, 0.9510565162951535312, 1.000000000000000000, 0.9510565162951535312, 1.000000000000000000, 0.9510565162951535312, 1.000000000000000000, 0.9510565162951535312, 1.000000000000000000, 0.9510565162951535312, 1.000000000000000000, 0.9510565162951535312, 1.000000000000000000, 0.9510565162951535312, 1.000000000000000000, 0.9510565162951535312, 1.000000000000000000, 0.9510565162951535312, 1.000000000000000000, 0.9510565162951535312, 1.000000000000000000, 0.9510565162951535312, 1.000000000000000000, 0.9510565162951535312, 1.000000000000000000, 0.9510565162951535312, 1.000000000000000000, 0.9510565162951535312, 1.000000000000000000, 0.9510565162951535312, 1.000000000000000000, 0.9510565162951535312, 1.000000000000000000, 0.9510565162951535312, 1.000000000000000000, 0.9510565162951535312, 1.000000000000000000),
 ( 1.000000000000000000, 0.9510565162951535312, 1.000000000000000000, 0.9510565162951535312, 1.000000000000000000, 0.9510565162951535312, 1.000000000000000000, 0.9510565162951535312, 1.000000000000000000, 0.9510565162951535312, 1.000000000000000000, 0.9510565162951535312, 1.000000000000000000, 0.9510565162951535312, 1.000000000000000000, 0.9510565162951535312, 1.000000000000000000, 0.9510565162951535312, 1.000000000000000000, 0.9510565162951535312, 1.000000000000000000, 0.9510565162951535312, 1.000000000000000000, 0.9510565162951535312, 1.000000000000000000, 0.9510565162951535312, 1.000000000000000000, 0.9510565162951535312, 1.000000000000000000, 0.9510565162951535312, 1.000000000000000000, 0.9510565162951535312, 1.000000000000000000, 0.9510565162951535312, 1.000000000000000000, 0.9510565162951535312, 1.000000000000000000, 0.9510565162951535312, 1.000000000000000000, 0.9510565162951535312, 1.000000000000000000, 0.9510565162951535312, 1.000000000000000000, 0.9510565162951535312, 1.000000000000000000, 0.9510565162951535312, 1.000000000000000000, 0.9510565162951535312, 1.000000000000000000, 0.9510565162951535312, 1.000000000000000000, 0.9510565162951535312, 1.000000000000000000, 0.9510565162951535312, 1.000000000000000000, 0.9510565162951535312, 1.000000000000000000, 0.9510565162951535312, 1.000000000000000000, 0.9510565162951535312, 1.000000000000000000, 0.9510565162951535312, 1.000000000000000000, 0.9510565162951535312, 1.000000000000000000, 0.9510565162951535312, 1.000000000000000000, 0.9510565162951535312, 1.000000000000000000, 0.9510565162951535312, 1.000000000000000000, 0.9510565162951535312, 1.000000000000000000, 0.9510565162951535312, 1.000000000000000000, 0.9510565162951535312, 1.000000000000000000, 0.9510565162951535312, 1.000000000000000000, 0.9510565162951535312, 1.000000000000000000, 0.9510565162951535312, 1.000000000000000000, 0.9510565162951535312, 1.000000000000000000, 0.9510565162951535312, 1.000000000000000000, 0.9510565162951535312, 1.000000000000000000, 0.9510565162951535312, 1.000000000000000000, 0.9510565162951535312, 1.000000000000000000, 0.9510565162951535312, 1.000000000000000000, 0.9510565162951535312, 1.000000000000000000, 0.9510565162951535312, 1.000000000000000000, 0.9510565162951535312, 1.000000000000000000, 0.9510565162951535312, 1.000000000000000000, 0.9510565162951535312, 1.000000000000000000, 0.9510565162951535312, 1.000000000000000000, 0.9510565162951535312, 1.000000000000000000, 0.9510565162951535312, 1.000000000000000000, 0.9510565162951535312, 1.000000000000000000, 0.9510565162951535312, 1.000000000000000000, 0.9510565162951535312, 1.000000000000000000, 0.9510565162951535312, 1.000000000000000000, 0.9510565162951535312, 1.000000000000000000, 0.9510565162951535312, 1.000000000000000000, 0.9510565162951535312, 1.000000000000000000, 0.9510565162951535312, 1.000000000000000000, 0.9510565162951535312, 1.000000000000000000, 0.9510565162951535312, 1.000000000000000000, 0.9510565162951535312, 1.000000000000000000, 0.9510565162951535312, 1.000000000000000000, 0.9510565162951535312, 1.000000000000000000, 0.9510565162951535312, 1.000000000000000000, 0.9510565162951535312, 1.000000000000000000, 0.9510565162951535312, 1.000000000000000000, 0.9510565162951535312, 1.000000000000000000, 0.9510565162951535312, 1.000000000000000000, 0.9510565162951535312, 1.000000000000000000, 0.9510565162951535312, 1.000000000000000000, 0.9510565162951535312, 1.000000000000000000, 0.9510565162951535312, 1.000000000000000000, 0.9510565162951535312, 1.000000000000000000, 0.9510565162951535312, 1.000000000000000000, 0.9510565162951535312, 1.000000000000000000, 0.9510565162951535312, 1.000000000000000000, 0.9510565162951535312, 1.000000000000000000, 0.9510565162951535312, 1.000000000000000000, 0.9510565162951535312, 1.000000000000000000, 0.9510565162951535312, 1.000000000000000000, 0.9510565162951535312, 1.000000000000000000, 0.9510565162951535312, 1.000000000000000000, 0.9510565162951535312, 1.000000000000000000, 0.9510565162951535312, 1.000000000000000000, 0.9510565162951535312, 1.000000000000000000, 0.9510565162951535312, 1.000000000000000000, 0.9510565162951535312, 1.000000000000000000, 0.9510565162951535312, 1.000000000000000000, 0.9510565162951535312, 1.000000000000000000, 0.9510565162951535312, 1.000000000000000000, 0.9510565162951535312, 1.000000000000000000, 0.9510565162951535312, 1.000000000000000000, 0.9510565162951535312, 1.000000000000000000, 0.9510565162951535312, 1.000000000000000000, 0.9510565162951535312, 1.000000000000000000, 0.9510565162951535312, 1.000000000000000000, 0.9510565162951535312, 1.000000000000000000, 0.9510565162951535312, 1.000000000000000000, 0.9510565162951535312, 1.000000000000000000, 0.9510565162951535312, 1.000000000000000000, 0.9510565162951535312, 1.000000000000000000, 0.9510565162951535312, 1.000000000000000000, 0.9510565162951535312, 1.000000000000000000, 0.9510565162951535312, 1.000000000000000000, 0.9510565162951535312, 1.000000000000000000, 0.9510565162951535312, 1.000000000000000000, 0.9510565162951535312, 1.000000000000000000, 0.9510565162951535312, 1.000000000000000000, 0.9510565162951535312, 1.000000000000000000, 0.9510565162951535312, 1.000000000000000000, 0.9510565162951535312, 1.000000000000000000, 0.9510565162951535312, 1.000000000000000000, 0.9510565162951535312, 1.000000000000000000, 0.9510565162951535312, 1.000000000000000000, 0.9510565162951535312, 1.000000000000000000, 0.9510565162951535312, 1.000000000000000000, 0.9510565162951535312, 1.000000000000000000, 0.9510565162951535312, 1.000000000000000000, 0.9510565162951535312, 1.000000000000000000, 0.9510565162951535312, 1.000000000000000000, 0.9510565162951535312, 1.000000000000000000, 0.9510565162951535312, 1.000000000000000000, 0.9510565162951535312, 1.000000000000000000, 0.9510565162951535312, 1.000000000000000000, 0.9510565162951535312, 1.000000000000000000, 0.9510565162951535312, 1.000000000000000000, 0.9510565162951535312, 1.000000000000000000, 0.9510565162951535312, 1.000000000000000000, 0.9510565162951535312, 1.000000000000000000, 0.9510565162951535312, 1.000000000000000000, 0.9510565162951535312, 1.000000000000000000, 0.9510565162951535312, 1.000000000000000000, 0.9510565162951535312, 1.000000000000000000, 0.9510565162951535312, 1.000000000000000000, 0.9510565162951535312, 1.000000000000000000, 0.9510565162951535312, 1.000000000000000000, 0.9510565162951535312, 1.000000000000000000, 0.9510565162951535312, 1.000000000000000000, 0.9510565162951535312, 1.000000000000000000, 0.9510565162951535312, 1.000000000000000000, 0.9510565162951535312, 1.000000000000000000, 0.9510565162951535312, 1.000000000000000000, 0.9510565162951535312, 1.000000000000000000, 0.9510565162951535312, 1.000000000000000000, 0.9510565162951535312, 1.000000000000000000, 0.9510565162951535312, 1.000000000000000000, 0.9510565162951535312, 1.000000000000000000, 0.9510565162951535312, 1.000000000000000000, 0.9510565162951535312, 1.000000000000000000, 0.9510565162951535312, 1.000000000000000000, 0.9510565162951535312, 1.000000000000000000, 0.9510565162951535312, 1.000000000000000000, 0.9510565162951535312, 1.000000000000000000, 0.9510565162951535312, 1.000000000000000000, 0.9510565162951535312, 1.000000000000000000, 0.9510565162951535312, 1.000000000000000000, 0.9510565162951535312, 1.000000000000000000, 0.9510565162951535312, 1.000000000000000000, 0.9510565162951535312, 1.000000000000000000, 0.9510565162951535312, 1.000000000000000000, 0.9510565162951535312, 1.000000000000000000, 0.9510565162951535312, 1.000000000000000000, 0.9510565162951535312, 1.000000000000000000, 0.9510565162951535312, 1.000000000000000000, 0.9510565162951535312, 1.000000000000000000, 0.9510565162951535312, 1.000000000000000000, 0.9510565162951535312, 1.000000000000000000, 0.9510565162951535312, 1.000000000000000000, 0.9510565162951535312, 1.000000000000000000, 0.9510565162951535312, 1.000000000000000000, 0.9510565162951535312, 1.000000000000000000, 0.9510565162951535312, 1.000000000000000000, 0.9510565162951535312, 1.000000000000000000, 0.9510565162951535312, 1.000000000000000000, 0.9510565162951535312, 1.000000000000000000, 0.9510565162951535312, 1.000000000000000000, 0.9510565162951535312, 1.000000000000000000, 0.9510565162951535312, 1.000000000000000000, 0.9510565162951535312, 1.000000000000000000, 0.9510565162951535312, 1.000000000000000000, 0.9510565162951535312, 1.000000000000000000, 0.9510565162951535312, 1.000000000000000000, 0.9510565162951535312, 1.000000000000000000, 0.9510565162951535312, 1.000000000000000000, 0.9510565162951535312, 1.000000000000000000, 0.9510565162951535312, 1.000000000000000000, 0.9510565162951535312, 1.000000000000000000, 0.9510565162951535312, 1.000000000000000000, 0.9510565162951535312, 1.000000000000000000, 0.9510565162951535312, 1.000000000000000000, 0.9510565162951535312, 1.000000000000000000, 0.9510565162951535312, 1.000000000000000000, 0.9510565162951535312, 1.000000000000000000, 0.9510565162951535312, 1.000000000000000000, 0.9510565162951535312, 1.000000000000000000, 0.9510565162951535312, 1.000000000000000000, 0.9510565162951535312, 1.000000000000000000, 0.9510565162951535312, 1.000000000000000000, 0.9510565162951535312, 1.000000000000000000, 0.9510565162951535312, 1.000000000000000000, 0.9510565162951535312, 1.000000000000000000, 0.9510565162951535312, 1.000000000000000000, 0.9510565162951535312, 1.000000000000000000, 0.9510565162951535312, 1.000000000000000000, 0.9510565162951535312, 1.000000000000000000, 0.9510565162951535312, 1.000000000000000000, 0.9510565162951535312, 1.000000000000000000, 0.9510565162951535312, 1.000000000000000000, 0.9510565162951535312, 1.000000000000000000, 0.9510565162951535312, 1.000000000000000000, 0.9510565162951535312, 1.000000000000000000, 0.9510565162951535312, 1.000000000000000000, 0.9510565162951535312, 1.000000000000000000, 0.9510565162951535312, 1.000000000000000000, 0.9510565162951535312, 1.000000000000000000, 0.9510565162951535312, 1.000000000000000000, 0.9510565162951535312, 1.000000000000000000, 0.9510565162951535312, 1.000000000000000000, 0.9510565162951535312, 1.000000000000000000, 0.9510565162951535312, 1.000000000000000000, 0.9510565162951535312, 1.000000000000000000, 0.9510565162951535312, 1.000000000000000000, 0.9510565162951535312, 1.000000000000000000, 0.9510565162951535312, 1.000000000000000000, 0.9510565162951535312, 1.000000000000000000, 0.9510565162951535312, 1.000000000000000000, 0.9510565162951535312, 1.000000000000000000, 0.9510565162951535312, 1.000000000000000000, 0.9510565162951535312, 1.000000000000000000, 0.9510565162951535312, 1.000000000000000000, 0.9510565162951535312, 1.000000000000000000, 0.9510565162951535312, 1.000000000000000000, 0.9510565162951535312, 1.000000000000000000, 0.9510565162951535312, 1.000000000000000000, 0.9510565162951535312, 1.000000000000000000, 0.9510565162951535312, 1.000000000000000000, 0.9510565162951535312, 1.000000000000000000, 0.9510565162951535312, 1.000000000000000000, 0.9510565162951535312, 1.000000000000000000, 0.9510565162951535312, 1.000000000000000000, 0.9510565162951535312, 1.000000000000000000, 0.9510565162951535312, 1.000000000000000000, 0.9510565162951535312, 1.000000000000000000, 0.9510565162951535312, 1.000000000000000000, 0.9510565162951535312, 1.000000000000000000, 0.9510565162951535312, 1.000000000000000000, 0.9510565162951535312, 1.000000000000000000, 0.9510565162951535312, 1.000000000000000000, 0.9510565162951535312, 1.000000000000000000, 0.9510565162951535312, 1.000000000000000000, 0.9510565162951535312, 1.000000000000000000, 0.9510565162951535312, 1.000000000000000000, 0.9510565162951535312, 1.000000000000000000, 0.9510565162951535312, 1.000000000000000000, 0.9510565162951535312, 1.000000000000000000, 0.9510565162951535312, 1.000000000000000000, 0.9510565162951535312, 1.000000000000000000, 0.9510565162951535312, 1.000000000000000000, 0.9510565162951535312, 1.000000000000000000, 0.9510565162951535312, 1.000000000000000000, 0.9510565162951535312, 1.000000000000000000, 0.9510565162951535312, 1.000000000000000000, 0.9510565162951535312, 1.000000000000000000, 0.9510565162951535312, 1.000000000000000000, 0.9510565162951535312, 1.000000000000000000, 0.9510565162951535312, 1.000000000000000000, 0.9510565162951535312, 1.000000000000000000, 0.9510565162951535312, 1.000000000000000000, 0.9510565162951535312, 1.000000000000000000, 0.9510565162951535312, 1.000000000000000000) ) ) 
 REPRESENTATION_ITEM ( '' )  SURFACE ( )  );
#21337=ORIENTED_EDGE ( 'NONE', *, *, #15407, .F. ) ;
#21341=CYLINDRICAL_SURFACE ( 'NONE', #23574, 15.00000000000001776 ) ;
#21344=VECTOR ( 'NONE', #15098, 1000.000000000000000 ) ;
#21355=CARTESIAN_POINT ( 'NONE',  ( 34.97499999726881015, 140.1801316387863778, -4.815267126137194431 ) ) ;
#21360=CARTESIAN_POINT ( 'NONE',  ( 57.79999999999999716, 142.6655632788954620, 8.961492836873471646 ) ) ;
#21362=CARTESIAN_POINT ( 'NONE',  ( 84.31132485994280046, 169.2658477444273331, 4.635254915624208216 ) ) ;
#21365=CARTESIAN_POINT ( 'NONE',  ( 60.52499999726881441, 140.1801316387863778, 4.815267126137185549 ) ) ;
#21368=CARTESIAN_POINT ( 'NONE',  ( 36.71132485994280614, 155.0000000000000000, 15.00000000000001243 ) ) ;
#21369=CARTESIAN_POINT ( 'NONE',  ( 64.42499999726879878, 141.7447067706911810, 9.630534252274376428 ) ) ;
#21370=CARTESIAN_POINT ( 'NONE',  ( 79.57499999726881867, 164.1591823560292198, -12.60653300113719766 ) ) ;
#21386=AXIS2_PLACEMENT_3D ( 'NONE', #26436, #6501, #24725 ) ;
#21388=CARTESIAN_POINT ( 'NONE',  ( 32.50000000000000000, 155.0000000000000000, -6.938893903907228378E-15 ) ) ;
#21392=ORIENTED_EDGE ( 'NONE', *, *, #16983, .T. ) ;
#21393=ADVANCED_FACE ( 'NONE', ( #12483 ), #4305, .T. ) ;
#21395=CARTESIAN_POINT ( 'NONE',  ( 79.72499999726881015, 169.8198683612136222, 4.815267126137181997 ) ) ;
#21397=CYLINDRICAL_SURFACE ( 'NONE', #16244, 15.00000000000001776 ) ;
#21399=CARTESIAN_POINT ( 'NONE',  ( 72.32499999726880446, 145.8408176439707802, 12.60653300113718345 ) ) ;
#21405=CARTESIAN_POINT ( 'NONE',  ( 36.29999999999999716, 146.4771138417591203, -11.73074641843674470 ) ) ;
#21413=AXIS2_PLACEMENT_3D ( 'NONE', #17092, #11977, #9585 ) ;
#21415=CARTESIAN_POINT ( 'NONE',  ( 45.92499999726881299, 164.1591823560292198, 12.60653300113718167 ) ) ;
#21423=CARTESIAN_POINT ( 'NONE',  ( 80.79999999453762882, 163.5228861582408797, 11.73074641843673049 ) ) ;
#21426=EDGE_CURVE ( 'NONE', #31727, #6290, #14859, .T. ) ;
#21436=CARTESIAN_POINT ( 'NONE',  ( 76.17499999726881299, 164.1591823560292198, 12.60653300113718167 ) ) ;
#21437=CARTESIAN_POINT ( 'NONE',  ( 53.31132485994280756, 140.7341522555726669, -4.635254915624220651 ) ) ;
#21441=CIRCLE ( 'NONE', #28517, 2.149999999999985256 ) ;
#21443=( NAMED_UNIT ( * ) SI_UNIT ( $, .STERADIAN. ) SOLID_ANGLE_UNIT ( ) );
#21445=CARTESIAN_POINT ( 'NONE',  ( 68.47499999726879594, 149.9369285172503510, 15.58253174999999580 ) ) ;
#21447=CARTESIAN_POINT ( 'NONE',  ( 41.38867513459481984, 169.2658477444273331, 4.635254915624208216 ) ) ;
#21451=CARTESIAN_POINT ( 'NONE',  ( 83.68867513459485963, 159.8737954434934636, 15.00000000000014211 ) ) ;
#21453=CARTESIAN_POINT ( 'NONE',  ( 87.77499999726882152, 169.8198683612136222, -4.815267126137197984 ) ) ;
#21455=( GEOMETRIC_REPRESENTATION_CONTEXT ( 3 ) GLOBAL_UNCERTAINTY_ASSIGNED_CONTEXT ( ( #17525 ) ) GLOBAL_UNIT_ASSIGNED_CONTEXT ( ( #12784, #31345, #13437 ) ) REPRESENTATION_CONTEXT ( 'NONE', 'WORKASPACE' ) );
#21457=CARTESIAN_POINT ( 'NONE',  ( 36.12499999726881583, 155.0000000000000000, 15.58253174999999402 ) ) ;
#21458=CARTESIAN_POINT ( 'NONE',  ( 80.78867513459482552, 155.0000000000000000, -15.00000000000002487 ) ) ;
#21462=CARTESIAN_POINT ( 'NONE',  ( 59.37499999726881583, 155.0000000000000000, -15.58253175000000823 ) ) ;
#21468=CARTESIAN_POINT ( 'NONE',  ( 62.39999999453763024, 168.7903194862797420, -4.480746418436745593 ) ) ;
#21471=DIRECTION ( 'NONE',  ( 1.000000000000000000, 0.000000000000000000, 0.000000000000000000 ) ) ;
#21479=CARTESIAN_POINT ( 'NONE',  ( 127.5000000000000000, 154.9999999999996305, -106.0000000000000142 ) ) ;
#21485=CARTESIAN_POINT ( 'NONE',  ( 43.47499999726881015, 160.0630714827496206, -15.58253175000000823 ) ) ;
#21487=CARTESIAN_POINT ( 'NONE',  ( 56.12499999726880873, 155.0000000000000000, 15.58253174999999402 ) ) ;
#21489=CARTESIAN_POINT ( 'NONE',  ( 60.88867513459483405, 159.8737954434936910, -14.99999999999998046 ) ) ;
#21492=CARTESIAN_POINT ( 'NONE',  ( 54.87499999726880162, 138.6155565068815463, -3.929120461958505118E-15 ) ) ;
#21495=CARTESIAN_POINT ( 'NONE',  ( 74.40000000000000568, 150.2886644046228639, -14.50000000000000888 ) ) ;
#21496=CARTESIAN_POINT ( 'NONE',  ( 65.58867513459482268, 163.8167787843871110, 12.13525491562421621 ) ) ;
#21497=FACE_OUTER_BOUND ( 'NONE', #17670, .T. ) ;
#21500=CARTESIAN_POINT ( 'NONE',  ( 36.67499999726879878, 141.7447067706911810, 9.630534252274376428 ) ) ;
#21502=CARTESIAN_POINT ( 'NONE',  ( 77.72499999726881015, 169.8198683612136222, 4.815267126137181997 ) ) ;
#21504=CARTESIAN_POINT ( 'NONE',  ( 48.11132485994281183, 169.2658477444273331, -4.635254915624224203 ) ) ;
#21505=CARTESIAN_POINT ( 'NONE',  ( 39.29999999453762882, 142.6655632788954620, 8.961492836873471646 ) ) ;
#21510=ORIENTED_EDGE ( 'NONE', *, *, #19724, .T. ) ;
#21515=EDGE_LOOP ( 'NONE', ( #1114, #33687 ) ) ;
#21524=CARTESIAN_POINT ( 'NONE',  ( 86.92499999726881299, 145.8408176439707802, -12.60653300113719588 ) ) ;
#21528=CARTESIAN_POINT ( 'NONE',  ( 53.79999999999999005, 142.6655632788954620, 8.961492836873471646 ) ) ;
#21531=( BOUNDED_CURVE ( )  B_SPLINE_CURVE ( 2, ( #9508, #19732, #23097, #17988, #30129, #4868, #25019, #32845, #17350, #19395, #24511 ),
 .UNSPECIFIED., .F., .T. ) 
 B_SPLINE_CURVE_WITH_KNOTS ( ( 3, 2, 2, 2, 2, 3 ),
 ( 0.3571428571428569287, 0.3607142857142854875, 0.3642857142857140462, 0.3678571428571425495, 0.3714285714285711082, 0.3749999999999997780 ),
 .UNSPECIFIED. ) 
 CURVE ( )  GEOMETRIC_REPRESENTATION_ITEM ( )  RATIONAL_B_SPLINE_CURVE ( ( 1.000000000000002220, 0.9510565162951510887, 1.000000000000000000, 0.9510565162951534202, 1.000000000000000000, 0.9510565162951534202, 1.000000000000000000, 0.9510565162951534202, 1.000000000000000000, 0.9510565162951564178, 0.9999999999999970024 ) ) 
 REPRESENTATION_ITEM ( '' )  );
#21532=CARTESIAN_POINT ( 'NONE',  ( 60.82499999726881867, 141.7447067706911810, -9.630534252274385310 ) ) ;
#21534=CARTESIAN_POINT ( 'NONE',  ( 79.78867513459482552, 155.0000000000000000, 15.00000000000001243 ) ) ;
#21535=CARTESIAN_POINT ( 'NONE',  ( 62.92499999726880588, 145.8408176439707802, -12.60653300113719588 ) ) ;
#21536=CARTESIAN_POINT ( 'NONE',  ( 74.17499999726881299, 164.1591823560292198, 12.60653300113718167 ) ) ;
#21553=ORIENTED_EDGE ( 'NONE', *, *, #10381, .F. ) ;
#21555=CARTESIAN_POINT ( 'NONE',  ( 77.02499999726880731, 149.9369285172503510, -15.58253175000000823 ) ) ;
#21559=CARTESIAN_POINT ( 'NONE',  ( 72.72499999726881015, 140.1801316387863778, -4.815267126137194431 ) ) ;
#21564=CARTESIAN_POINT ( 'NONE',  ( 34.80000000000000426, 167.3344367211045096, -8.961492836873482304 ) ) ;
#21573=CARTESIAN_POINT ( 'NONE',  ( 46.02499999726880731, 160.0630714827496206, 15.58253174999999224 ) ) ;
#21580=CARTESIAN_POINT ( 'NONE',  ( 87.39999999453762314, 141.2096805137202580, 4.480746418436733158 ) ) ;
#21588=ORIENTED_EDGE ( 'NONE', *, *, #20497, .F. ) ;
#21593=VERTEX_POINT ( 'NONE', #32938 ) ;
#21596=CARTESIAN_POINT ( 'NONE',  ( 78.47499999726881015, 149.9369285172503510, 15.58253174999999580 ) ) ;
#21597=CARTESIAN_POINT ( 'NONE',  ( 86.88867513459483405, 159.8737954434935489, -15.00000000000009237 ) ) ;
#21601=CARTESIAN_POINT ( 'NONE',  ( 70.37499999726881583, 155.0000000000000000, 15.58253174999999402 ) ) ;
#21602=ORIENTED_EDGE ( 'NONE', *, *, #13220, .F. ) ;
#21606=CARTESIAN_POINT ( 'NONE',  ( 42.98867513459482836, 163.8167787843871110, -12.13525491562423397 ) ) ;
#21612=CARTESIAN_POINT ( 'NONE',  ( 82.17499999726882720, 164.1591823560292198, 12.60653300113718167 ) ) ;
#21616=CARTESIAN_POINT ( 'NONE',  ( 36.02499999726881441, 160.0630714827496206, 15.58253174999999402 ) ) ;
#21617=CARTESIAN_POINT ( 'NONE',  ( 80.88867513459481984, 159.8737954434937762, -14.99999999999989519 ) ) ;
#21621=CARTESIAN_POINT ( 'NONE',  ( 64.37499999726881583, 155.0000000000000000, 15.58253174999999402 ) ) ;
#21630=CARTESIAN_POINT ( 'NONE',  ( 58.79999999453762882, 163.5228861582408797, 11.73074641843673049 ) ) ;
#21636=CARTESIAN_POINT ( 'NONE',  ( 71.18867513459481700, 169.2658477444273331, -4.635254915624224203 ) ) ;
#21637=ORIENTED_EDGE ( 'NONE', *, *, #19354, .T. ) ;
#21642=CARTESIAN_POINT ( 'NONE',  ( 50.51132485994281041, 163.8167787843871110, 12.13525491562421621 ) ) ;
#21648=CARTESIAN_POINT ( 'NONE',  ( 52.07499999726881157, 168.2552932293087906, 9.630534252274372875 ) ) ;
#21650=CARTESIAN_POINT ( 'NONE',  ( 55.42499999726879878, 168.2552932293087906, -9.630534252274385310 ) ) ;
#21655=CARTESIAN_POINT ( 'NONE',  ( 59.57499999726881157, 164.1591823560292198, -12.60653300113719766 ) ) ;
#21657=CARTESIAN_POINT ( 'NONE',  ( 73.28867513459483973, 170.7719333635740497, -7.904646289410545231E-15 ) ) ;
#21661=CARTESIAN_POINT ( 'NONE',  ( 76.39999999999996305, 150.2886644046228639, -14.50000000000000888 ) ) ;
#21662=CARTESIAN_POINT ( 'NONE',  ( 65.08867513459482268, 167.7597621252805880, -9.270509831248443078 ) ) ;
#21665=CIRCLE ( 'NONE', #11869, 100.0000000000000284 ) ;
#21667=CARTESIAN_POINT ( 'NONE',  ( 37.87499999726880873, 171.3844434931184253, -7.942151717890132712E-15 ) ) ;
#21672=CARTESIAN_POINT ( 'NONE',  ( 77.32499999726881867, 164.1591823560292198, -12.60653300113719766 ) ) ;
#21675=CARTESIAN_POINT ( 'NONE',  ( 41.49999999453762456, 139.7537977485451393, -4.138211985947621020E-15 ) ) ;
#21678=CARTESIAN_POINT ( 'NONE',  ( 39.91132485994280898, 163.8167787843871110, -12.13525491562423397 ) ) ;
#21679=AXIS2_PLACEMENT_3D ( 'NONE', #5249, #23647, #15304 ) ;
#21681=ORIENTED_EDGE ( 'NONE', *, *, #31027, .T. ) ;
#21694=CARTESIAN_POINT ( 'NONE',  ( 39.42499999726881299, 168.2552932293087906, -9.630534252274385310 ) ) ;
#21697=CARTESIAN_POINT ( 'NONE',  ( 34.57499999726881157, 145.8408176439707802, 12.60653300113718345 ) ) ;
#21700=CIRCLE ( 'NONE', #21168, 2.149999999999985256 ) ;
#21701=CARTESIAN_POINT ( 'NONE',  ( 56.09999999999999432, 141.2096805137202580, -4.480746418436742040 ) ) ;
#21703=CARTESIAN_POINT ( 'NONE',  ( 127.5000000000000000, 261.0000000000000000, 0.000000000000000000 ) ) ;
#21704=CARTESIAN_POINT ( 'NONE',  ( 56.62499999726880162, 138.6155565068815463, -3.929120461958505118E-15 ) ) ;
#21707=CARTESIAN_POINT ( 'NONE',  ( 37.21132485994281325, 139.2280666364260071, -4.041636747397287284E-15 ) ) ;
#21708=CARTESIAN_POINT ( 'NONE',  ( 65.32499999726881867, 164.1591823560292198, -12.60653300113719766 ) ) ;
#21709=CARTESIAN_POINT ( 'NONE',  ( 73.77499999726882152, 169.8198683612136222, -4.815267126137197984 ) ) ;
#21728=CARTESIAN_POINT ( 'NONE',  ( 81.42499999726882720, 168.2552932293087906, -9.630534252274387086 ) ) ;
#21730=CARTESIAN_POINT ( 'NONE',  ( 68.98867513459482836, 163.8167787843871110, -12.13525491562423397 ) ) ;
#21732=CARTESIAN_POINT ( 'NONE',  ( 71.62499999726881583, 171.3844434931184253, -7.942151717890132712E-15 ) ) ;
#21733=( BOUNDED_CURVE ( )  B_SPLINE_CURVE ( 2, ( #14187, #11303, #3960, #11142, #14017, #32576, #16571, #31904, #1241, #18967, #32079 ),
 .UNSPECIFIED., .F., .T. ) 
 B_SPLINE_CURVE_WITH_KNOTS ( ( 3, 2, 2, 2, 2, 3 ),
 ( 0.3035714285714285476, 0.3071428571428571619, 0.3107142857142857761, 0.3142857142857143349, 0.3178571428571429491, 0.3214285714285715634 ),
 .UNSPECIFIED. ) 
 CURVE ( )  GEOMETRIC_REPRESENTATION_ITEM ( )  RATIONAL_B_SPLINE_CURVE ( ( 1.000000000000000000, 0.9510565162951534202, 1.000000000000000000, 0.9510565162951534202, 1.000000000000000000, 0.9510565162951534202, 1.000000000000000000, 0.9510565162951534202, 1.000000000000000000, 0.9510565162951518658, 1.000000000000001554 ) ) 
 REPRESENTATION_ITEM ( '' )  );
#21736=CARTESIAN_POINT ( 'NONE',  ( 57.91132485994280898, 163.8167787843871110, -12.13525491562423397 ) ) ;
#21737=CARTESIAN_POINT ( 'NONE',  ( 37.70000000000000284, 146.4771138417591203, 11.73074641843673227 ) ) ;
#21744=CARTESIAN_POINT ( 'NONE',  ( 81.78867513459482552, 155.0000000000000000, 15.00000000000001243 ) ) ;
#21745=CARTESIAN_POINT ( 'NONE',  ( 47.02499999726881441, 149.9369285172503510, -15.58253175000000823 ) ) ;
#21753=CARTESIAN_POINT ( 'NONE',  ( 83.89999999453763735, 150.2886644046228639, -14.50000000000000888 ) ) ;
#21761=CARTESIAN_POINT ( 'NONE',  ( 70.07499999726881867, 168.2552932293087906, 9.630534252274372875 ) ) ;
#21764=CARTESIAN_POINT ( 'NONE',  ( 73.97499999726881015, 169.8198683612136222, 4.815267126137181997 ) ) ;
#21771=CARTESIAN_POINT ( 'NONE',  ( 70.87499999726880162, 138.6155565068815747, -3.929120461958505118E-15 ) ) ;
#21780=CARTESIAN_POINT ( 'NONE',  ( 85.47499999726879594, 160.0630714827496206, -15.58253175000000823 ) ) ;
#21783=CARTESIAN_POINT ( 'NONE',  ( 41.12499999726880873, 155.0000000000000000, -15.58253175000000823 ) ) ;
#21784=DIRECTION ( 'NONE',  ( 1.000000000000000000, 0.000000000000000000, 0.000000000000000000 ) ) ;
#21785=FACE_OUTER_BOUND ( 'NONE', #8414, .T. ) ;
#21795=CARTESIAN_POINT ( 'NONE',  ( 67.39999999453763735, 141.2096805137202580, 4.480746418436733158 ) ) ;
#21799=CARTESIAN_POINT ( 'NONE',  ( 83.21132485994282035, 139.2280666364260071, -4.041636747397287284E-15 ) ) ;
#21805=CARTESIAN_POINT ( 'NONE',  ( 50.71132485994280614, 155.0000000000000000, 15.00000000000001243 ) ) ;
#21807=ORIENTED_EDGE ( 'NONE', *, *, #29729, .F. ) ;
#21809=EDGE_CURVE ( 'NONE', #7596, #18104, #32598, .T. ) ;
#21810=FACE_OUTER_BOUND ( 'NONE', #5555, .T. ) ;
#21812=CARTESIAN_POINT ( 'NONE',  ( 51.17499999726880588, 145.8408176439707802, -12.60653300113719588 ) ) ;
#21814=CARTESIAN_POINT ( 'NONE',  ( 55.62499999726881583, 171.3844434931184253, -7.942151717890132712E-15 ) ) ;
#21816=CARTESIAN_POINT ( 'NONE',  ( 87.50000000000000000, 160.9457742543943652, -14.40357817542362540 ) ) ;
#21817=AXIS2_PLACEMENT_3D ( 'NONE', #22801, #20238, #26514 ) ;
#21821=CARTESIAN_POINT ( 'NONE',  ( 58.67499999726882010, 141.7447067706911810, 9.630534252274376428 ) ) ;
#21823=CARTESIAN_POINT ( 'NONE',  ( 73.18867513459481700, 169.2658477444273331, -4.635254915624224203 ) ) ;
#21825=CARTESIAN_POINT ( 'NONE',  ( 71.70000000000000284, 146.4771138417591203, 11.73074641843673227 ) ) ;
#21826=CARTESIAN_POINT ( 'NONE',  ( 61.81132485994281467, 159.8737954434936057, -15.00000000000002665 ) ) ;
#21829=CARTESIAN_POINT ( 'NONE',  ( 33.68867513459484542, 159.8737954434934920, 15.00000000000010836 ) ) ;
#21830=CARTESIAN_POINT ( 'NONE',  ( 47.27499999726880731, 149.9369285172503510, -15.58253175000000823 ) ) ;
#21832=CARTESIAN_POINT ( 'NONE',  ( 73.82499999726879025, 168.2552932293087906, 9.630534252274372875 ) ) ;
#21835=CARTESIAN_POINT ( 'NONE',  ( 50.29999999453763593, 167.3344367211045096, -8.961492836873482304 ) ) ;
#21839=EDGE_LOOP ( 'NONE', ( #1191, #32357, #26584, #8090 ) ) ;
#21846=EDGE_CURVE ( 'NONE', #30153, #7020, #8486, .T. ) ;
#21856=CARTESIAN_POINT ( 'NONE',  ( 40.72499999726881725, 140.1801316387863778, -4.815267126137194431 ) ) ;
#21859=CARTESIAN_POINT ( 'NONE',  ( 40.77499999726881441, 140.1801316387863778, 4.815267126137185549 ) ) ;
#21862=CARTESIAN_POINT ( 'NONE',  ( 52.59999999999999432, 159.7113355953771077, -14.50000000000000888 ) ) ;
#21863=FACE_BOUND ( 'NONE', #28235, .T. ) ;
#21867=CARTESIAN_POINT ( 'NONE',  ( 57.32499999726881157, 164.1591823560292198, -12.60653300113719766 ) ) ;
#21872=CARTESIAN_POINT ( 'NONE',  ( 68.12499999726881583, 155.0000000000000000, 15.58253174999999402 ) ) ;
#21873=CARTESIAN_POINT ( 'NONE',  ( 78.07499999726880446, 168.2552932293087906, 9.630534252274372875 ) ) ;
#21886=ORIENTED_EDGE ( 'NONE', *, *, #28982, .T. ) ;
#21888=CARTESIAN_POINT ( 'NONE',  ( 39.31132485994280756, 140.7341522555726669, -4.635254915624220651 ) ) ;
#21892=ORIENTED_EDGE ( 'NONE', *, *, #27707, .T. ) ;
#21893=CARTESIAN_POINT ( 'NONE',  ( 87.02499999726880731, 149.9369285172503510, -15.58253175000000823 ) ) ;
#21898=CARTESIAN_POINT ( 'NONE',  ( 79.02499999726879309, 149.9369285172503510, -15.58253175000000823 ) ) ;
#21902=CARTESIAN_POINT ( 'NONE',  ( 36.10000000000000142, 141.2096805137202580, -4.480746418436742040 ) ) ;
#21906=AXIS2_PLACEMENT_3D ( 'NONE', #15352, #25742, #20640 ) ;
#21910=CARTESIAN_POINT ( 'NONE',  ( 52.62499999726880873, 138.6155565068815747, -3.929120461958505118E-15 ) ) ;
#21913=PRODUCT_DEFINITION_SHAPE ( 'NONE', 'NONE',  #13732 ) ;
#21918=CARTESIAN_POINT ( 'NONE',  ( 83.69999999453763451, 142.6655632788954620, -8.961492836873480528 ) ) ;
#21929=CARTESIAN_POINT ( 'NONE',  ( 73.87499999726881583, 171.3844434931184253, -7.942151717890132712E-15 ) ) ;
#21932=CARTESIAN_POINT ( 'NONE',  ( 80.97499999726881015, 140.1801316387863778, -4.815267126137194431 ) ) ;
#21938=DIRECTION ( 'NONE',  ( 1.000000000000000000, 0.000000000000000000, 0.000000000000000000 ) ) ;
#21941=CARTESIAN_POINT ( 'NONE',  ( 71.07499999726880446, 141.7447067706911810, -9.630534252274387086 ) ) ;
#21942=EDGE_LOOP ( 'NONE', ( #19285, #26098, #23203 ) ) ;
#21946=CYLINDRICAL_SURFACE ( 'NONE', #11470, 15.00000000000001776 ) ;
#21955=CARTESIAN_POINT ( 'NONE',  ( 48.02499999726879309, 160.0630714827496206, 15.58253174999999402 ) ) ;
#21957=DIRECTION ( 'NONE',  ( 0.000000000000000000, 0.7071067811865411334, -0.7071067811865540120 ) ) ;
#21958=DIRECTION ( 'NONE',  ( 0.000000000000000000, 0.000000000000000000, -1.000000000000000000 ) ) ;
#21968=CARTESIAN_POINT ( 'NONE',  ( 67.09999999453762598, 150.2886644046228639, 14.49999999999999645 ) ) ;
#21978=AXIS2_PLACEMENT_3D ( 'NONE', #18053, #2732, #4 ) ;
#21986=CARTESIAN_POINT ( 'NONE',  ( 52.27499999726880731, 160.0630714827496206, 15.58253174999999224 ) ) ;
#21988=CARTESIAN_POINT ( 'NONE',  ( 55.02499999726881441, 149.9369285172503510, -15.58253175000000823 ) ) ;
#21995=CARTESIAN_POINT ( 'NONE',  ( 62.97499999726881015, 140.1801316387863778, -4.815267126137194431 ) ) ;
#22001=CARTESIAN_POINT ( 'NONE',  ( 79.10000000000000853, 168.7903194862797420, 4.480746418436729606 ) ) ;
#22006=CARTESIAN_POINT ( 'NONE',  ( 42.27499999726880731, 160.0630714827496206, 15.58253174999999402 ) ) ;
#22008=CARTESIAN_POINT ( 'NONE',  ( 77.62499999726880162, 171.3844434931184253, -7.942151717890132712E-15 ) ) ;
#22009=ORIENTED_EDGE ( 'NONE', *, *, #23088, .F. ) ;
#22012=CARTESIAN_POINT ( 'NONE',  ( 45.69999999453763451, 142.6655632788954620, -8.961492836873480528 ) ) ;
#22014=CARTESIAN_POINT ( 'NONE',  ( 127.5000000000000000, 155.0000000000000000, -6.938893903907228378E-15 ) ) ;
#22020=ADVANCED_FACE ( 'NONE', ( #23402 ), #21334, .F. ) ;
#22031=CARTESIAN_POINT ( 'NONE',  ( 38.12499999726880873, 155.0000000000000000, 15.58253174999999402 ) ) ;
#22034=CARTESIAN_POINT ( 'NONE',  ( 42.67499999726880588, 141.7447067706911810, 9.630534252274376428 ) ) ;
#22037=CARTESIAN_POINT ( 'NONE',  ( 62.89999999999999858, 168.7903194862797420, -4.480746418436745593 ) ) ;
#22042=EDGE_CURVE ( 'NONE', #26876, #3255, #14545, .T. ) ;
#22043=CARTESIAN_POINT ( 'NONE',  ( 59.72499999726881015, 169.8198683612136222, 4.815267126137181997 ) ) ;
#22046=DIRECTION ( 'NONE',  ( -1.000000000000000000, 0.000000000000000000, 0.000000000000000000 ) ) ;
#22047=CARTESIAN_POINT ( 'NONE',  ( 80.67499999726881299, 141.7447067706911810, 9.630534252274376428 ) ) ;
#22050=CARTESIAN_POINT ( 'NONE',  ( 32.50000000000000000, 155.0000000000000000, 15.00000000000001243 ) ) ;
#22056=DIRECTION ( 'NONE',  ( 1.000000000000000000, 0.000000000000000000, 0.000000000000000000 ) ) ;
#22064=LINE ( 'NONE', #16781, #420 ) ;
#22067=CARTESIAN_POINT ( 'NONE',  ( 83.22499999726881015, 160.0630714827496206, -15.58253175000000823 ) ) ;
#22070=CARTESIAN_POINT ( 'NONE',  ( 75.22499999726879594, 160.0630714827496206, -15.58253175000000823 ) ) ;
#22073=CARTESIAN_POINT ( 'NONE',  ( 87.50000000000000000, 170.0518911780263807, 2.651152351506866012 ) ) ;
#22074=CARTESIAN_POINT ( 'NONE',  ( 36.90000000000000568, 168.7903194862797420, -4.480746418436745593 ) ) ;
#22082=CARTESIAN_POINT ( 'NONE',  ( 49.12499999726880873, 155.0000000000000000, -15.58253175000000823 ) ) ;
#22091=CARTESIAN_POINT ( 'NONE',  ( 83.99999999453763166, 155.0000000000000000, -14.50000000000000711 ) ) ;
#22099=CARTESIAN_POINT ( 'NONE',  ( 74.87499999726880162, 138.6155565068815463, -3.929120461958505118E-15 ) ) ;
#22103=CARTESIAN_POINT ( 'NONE',  ( 81.07499999726880446, 141.7447067706911810, -9.630534252274387086 ) ) ;
#22104=DIRECTION ( 'NONE',  ( 0.000000000000000000, 0.000000000000000000, -1.000000000000000000 ) ) ;
#22109=CARTESIAN_POINT ( 'NONE',  ( 71.87499999726881583, 171.3844434931184253, -7.942151717890134290E-15 ) ) ;
#22114=CARTESIAN_POINT ( 'NONE',  ( 86.61132485994281183, 159.8737954434933499, 15.00000000000019895 ) ) ;
#22120=CARTESIAN_POINT ( 'NONE',  ( 44.72499999726881015, 140.1801316387863778, -4.815267126137194431 ) ) ;
#22122=CARTESIAN_POINT ( 'NONE',  ( 87.50000000000000000, 153.6504441981042532, -15.26259659777053912 ) ) ;
#22127=CARTESIAN_POINT ( 'NONE',  ( 76.78867513459483973, 155.0000000000000000, -15.00000000000002487 ) ) ;
#22131=CARTESIAN_POINT ( 'NONE',  ( 67.89999999453763735, 150.2886644046228639, -14.50000000000000888 ) ) ;
#22136=CARTESIAN_POINT ( 'NONE',  ( 45.41132485994281609, 142.2402378747194405, -9.270509831248439525 ) ) ;
#22138=EDGE_LOOP ( 'NONE', ( #19266, #10840, #1154, #14223 ) ) ;
#22141=CARTESIAN_POINT ( 'NONE',  ( 87.49999999999997158, 168.5097963921330120, -7.831877679450401253 ) ) ;
#22149=CARTESIAN_POINT ( 'NONE',  ( 47.97499999726881015, 169.8198683612136222, 4.815267126137181997 ) ) ;
#22153=AXIS2_PLACEMENT_3D ( 'NONE', #1834, #14775, #22613 ) ;
#22157=CARTESIAN_POINT ( 'NONE',  ( 61.37499999726880873, 155.0000000000000000, -15.58253175000000823 ) ) ;
#22163=CARTESIAN_POINT ( 'NONE',  ( 81.59999999999999432, 150.2886644046228639, 14.49999999999999645 ) ) ;
#22168=CARTESIAN_POINT ( 'NONE',  ( 47.67499999726880588, 168.2552932293087906, -9.630534252274385310 ) ) ;
#22170=CARTESIAN_POINT ( 'NONE',  ( 82.02499999726879309, 160.0630714827496206, 15.58253174999999402 ) ) ;
#22173=CARTESIAN_POINT ( 'NONE',  ( 46.99999999453763166, 155.0000000000000000, 14.49999999999999467 ) ) ;
#22178=CARTESIAN_POINT ( 'NONE',  ( 60.71132485994280614, 155.0000000000000000, 15.00000000000001243 ) ) ;
#22181=CARTESIAN_POINT ( 'NONE',  ( 66.51132485994278909, 163.8167787843871110, 12.13525491562421621 ) ) ;
#22182=ORIENTED_EDGE ( 'NONE', *, *, #26661, .T. ) ;
#22195=CARTESIAN_POINT ( 'NONE',  ( 36.22499999726881015, 149.9369285172503510, 15.58253174999999580 ) ) ;
#22200=CARTESIAN_POINT ( 'NONE',  ( 43.57499999726881157, 164.1591823560292198, -12.60653300113719766 ) ) ;
#22205=CARTESIAN_POINT ( 'NONE',  ( 60.99999999999999289, 170.2462022514548323, -7.872454543227099337E-15 ) ) ;
#22211=CARTESIAN_POINT ( 'NONE',  ( 66.42499999726879878, 141.7447067706911810, 9.630534252274376428 ) ) ;
#22214=DIRECTION ( 'NONE',  ( 0.000000000000000000, 0.7071067811865442421, -0.7071067811865506814 ) ) ;
#22215=CARTESIAN_POINT ( 'NONE',  ( 85.67499999726879878, 168.2552932293087906, -9.630534252274385310 ) ) ;
#22223=CYLINDRICAL_SURFACE ( 'NONE', #2876, 15.00000000000001776 ) ;
#22229=EDGE_CURVE ( 'NONE', #12386, #6526, #12036, .T. ) ;
#22235=CARTESIAN_POINT ( 'NONE',  ( 86.52499999726882152, 140.1801316387863778, 4.815267126137185549 ) ) ;
#22238=CARTESIAN_POINT ( 'NONE',  ( 77.32499999726881867, 164.1591823560292198, -12.60653300113719766 ) ) ;
#22242=CARTESIAN_POINT ( 'NONE',  ( 75.78867513459483973, 155.0000000000000000, 15.00000000000001243 ) ) ;
#22243=CARTESIAN_POINT ( 'NONE',  ( 39.69999999999999574, 146.4771138417591203, 11.73074641843673227 ) ) ;
#22250=CARTESIAN_POINT ( 'NONE',  ( 72.91132485994280898, 146.1832212156128890, 12.13525491562421976 ) ) ;
#22251=DIRECTION ( 'NONE',  ( 1.000000000000000000, 0.000000000000000000, 0.000000000000000000 ) ) ;
#22252=CARTESIAN_POINT ( 'NONE',  ( 54.12499999726881583, 155.0000000000000000, 15.58253174999999402 ) ) ;
#22253=CARTESIAN_POINT ( 'NONE',  ( 65.57499999726881867, 164.1591823560292198, -12.60653300113719766 ) ) ;
#22261=CARTESIAN_POINT ( 'NONE',  ( 84.49999999453764588, 170.2462022514548323, -7.872454543227099337E-15 ) ) ;
#22270=CARTESIAN_POINT ( 'NONE',  ( 70.77499999726880731, 140.1801316387863778, 4.815267126137185549 ) ) ;
#22275=CARTESIAN_POINT ( 'NONE',  ( 84.97499999726882436, 140.1801316387863778, -4.815267126137194431 ) ) ;
#22284=( BOUNDED_CURVE ( )  B_SPLINE_CURVE ( 2, ( #7016, #6332, #3787, #12625, #33245, #33585, #25578, #18081, #30699, #12289, #25403 ),
 .UNSPECIFIED., .F., .F. ) 
 B_SPLINE_CURVE_WITH_KNOTS ( ( 3, 2, 2, 2, 2, 3 ),
 ( 0.3214285714285715634, 0.3250000000000000666, 0.3285714285714285698, 0.3321428571428571286, 0.3357142857142856318, 0.3392857142857141906 ),
 .UNSPECIFIED. ) 
 CURVE ( )  GEOMETRIC_REPRESENTATION_ITEM ( )  RATIONAL_B_SPLINE_CURVE ( ( 0.9999999999999984457, 0.9510565162951549745, 1.000000000000000000, 0.9510565162951534202, 1.000000000000000000, 0.9510565162951534202, 1.000000000000000000, 0.9510565162951534202, 1.000000000000000000, 0.9510565162951549745, 0.9999999999999984457 ) ) 
 REPRESENTATION_ITEM ( '' )  );
#22286=CARTESIAN_POINT ( 'NONE',  ( 86.11132485994279762, 169.2658477444273331, -4.635254915624224203 ) ) ;
#22291=CARTESIAN_POINT ( 'NONE',  ( 71.71132485994280614, 155.0000000000000000, -15.00000000000002487 ) ) ;
#22294=CARTESIAN_POINT ( 'NONE',  ( 42.62499999726881583, 138.6155565068815463, -3.929120461958505118E-15 ) ) ;
#22296=CARTESIAN_POINT ( 'NONE',  ( 87.49999999999997158, 160.3090467171700482, -14.64008245857240276 ) ) ;
#22298=CARTESIAN_POINT ( 'NONE',  ( 81.88867513459483405, 150.1262045565062806, 14.99999999999992006 ) ) ;
#22301=DIRECTION ( 'NONE',  ( 1.000000000000000000, 0.000000000000000000, 0.000000000000000000 ) ) ;
#22305=CARTESIAN_POINT ( 'NONE',  ( 65.49999999453761745, 139.7537977485451393, -4.138211985947621020E-15 ) ) ;
#22320=CARTESIAN_POINT ( 'NONE',  ( 53.77499999726881441, 169.8198683612136222, -4.815267126137197984 ) ) ;
#22323=CARTESIAN_POINT ( 'NONE',  ( 66.91132485994280898, 146.1832212156128890, 12.13525491562421976 ) ) ;
#22326=CARTESIAN_POINT ( 'NONE',  ( 56.87499999726880162, 138.6155565068815463, -3.929120461958505118E-15 ) ) ;
#22332=CARTESIAN_POINT ( 'NONE',  ( 81.10000000000000853, 168.7903194862797420, 4.480746418436729606 ) ) ;
#22337=CARTESIAN_POINT ( 'NONE',  ( 41.97499999726881015, 169.8198683612136222, 4.815267126137181997 ) ) ;
#22339=CARTESIAN_POINT ( 'NONE',  ( 86.22499999726882436, 149.9369285172503510, 15.58253174999999580 ) ) ;
#22342=CARTESIAN_POINT ( 'NONE',  ( 47.59999999453763309, 141.2096805137202580, -4.480746418436742040 ) ) ;
#22352=FACE_OUTER_BOUND ( 'NONE', #3004, .T. ) ;
#22360=CARTESIAN_POINT ( 'NONE',  ( 37.62499999726880162, 171.3844434931184253, -7.942151717890132712E-15 ) ) ;
#22364=CARTESIAN_POINT ( 'NONE',  ( 39.77499999726881441, 169.8198683612136222, -4.815267126137197984 ) ) ;
#22368=EDGE_CURVE ( 'NONE', #29364, #18797, #19122, .T. ) ;
#22369=CARTESIAN_POINT ( 'NONE',  ( 58.50000000000000000, 155.0000000000000000, -14.50000000000000711 ) ) ;
#22375=CARTESIAN_POINT ( 'NONE',  ( 63.42499999726881299, 168.2552932293087906, -9.630534252274385310 ) ) ;
#22380=CARTESIAN_POINT ( 'NONE',  ( 85.37499999726881583, 155.0000000000000000, -15.58253175000000823 ) ) ;
#22381=B_SPLINE_CURVE_WITH_KNOTS ( 'NONE', 3,
 ( #9685, #22296, #29967, #30135, #24850, #24689, #19739, #17519, #1513, #27237, #11910, #22122, #20079, #32677, #6625, #30474, #9343, #12071, #25025, #19901 ),
 .UNSPECIFIED., .F., .F.,
 ( 4, 2, 2, 2, 2, 2, 2, 2, 2, 4 ),
 ( 0.000000000000000000, 0.002030509116170894305, 0.003045763674256341241, 0.004061018232341788610, 0.006091527348512682481, 0.007106781906598130284, 0.008122036464683577220, 0.01218305469702552456, 0.01421356381319653639, 0.01624407292936754996 ),
 .UNSPECIFIED. ) ;
#22397=CARTESIAN_POINT ( 'NONE',  ( 81.92499999726882720, 164.1591823560292198, 12.60653300113718167 ) ) ;
#22399=LINE ( 'NONE', #30074, #18331 ) ;
#22401=CARTESIAN_POINT ( 'NONE',  ( 77.72499999726881015, 169.8198683612136222, 4.815267126137181997 ) ) ;
#22404=CARTESIAN_POINT ( 'NONE',  ( 74.78867513459483973, 155.0000000000000000, -15.00000000000002487 ) ) ;
#22407=VECTOR ( 'NONE', #30208, 1000.000000000000000 ) ;
#22408=CARTESIAN_POINT ( 'NONE',  ( 41.80000000000000426, 142.6655632788954620, 8.961492836873471646 ) ) ;
#22413=CARTESIAN_POINT ( 'NONE',  ( 77.88867513459483405, 150.1262045565060816, 14.99999999999978328 ) ) ;
#22414=CARTESIAN_POINT ( 'NONE',  ( 32.50000000000000000, 155.0000000000000000, -6.938893903907228378E-15 ) ) ;
#22415=CARTESIAN_POINT ( 'NONE',  ( 53.42499999726880588, 168.2552932293087906, -9.630534252274387086 ) ) ;
#22416=CARTESIAN_POINT ( 'NONE',  ( 62.97499999726881015, 140.1801316387863778, -4.815267126137194431 ) ) ;
#22433=CARTESIAN_POINT ( 'NONE',  ( 69.37499999726881583, 155.0000000000000000, -15.58253175000000823 ) ) ;
#22438=CARTESIAN_POINT ( 'NONE',  ( 86.37499999726881583, 155.0000000000000000, 15.58253174999999402 ) ) ;
#22440=LINE ( 'NONE', #17336, #13229 ) ;
#22442=LINE ( 'NONE', #9165, #5834 ) ;
#22447=DIRECTION ( 'NONE',  ( 0.000000000000000000, 0.000000000000000000, -1.000000000000000000 ) ) ;
#22452=APPLICATION_CONTEXT ( 'automotive_design' ) ;
#22457=CARTESIAN_POINT ( 'NONE',  ( 45.02499999726880731, 149.9369285172503510, -15.58253175000000823 ) ) ;
#22459=CARTESIAN_POINT ( 'NONE',  ( 33.42499999726881299, 168.2552932293087906, -9.630534252274387086 ) ) ;
#22471=CARTESIAN_POINT ( 'NONE',  ( 64.49999999453764588, 170.2462022514548323, -7.872454543227099337E-15 ) ) ;
#22472=ORIENTED_EDGE ( 'NONE', *, *, #23457, .T. ) ;
#22478=ORIENTED_EDGE ( 'NONE', *, *, #9801, .F. ) ;
#22484=CARTESIAN_POINT ( 'NONE',  ( 58.58867513459482268, 146.1832212156128890, -12.13525491562423042 ) ) ;
#22486=VERTEX_POINT ( 'NONE', #29859 ) ;
#22488=( BOUNDED_CURVE ( )  B_SPLINE_CURVE ( 2, ( #3095, #549, #708, #11270, #29329, #29488, #29662, #29156, #13485, #21489, #6311 ),
 .UNSPECIFIED., .F., .T. ) 
 B_SPLINE_CURVE_WITH_KNOTS ( ( 3, 2, 2, 2, 2, 3 ),
 ( 0.4642857142857141906, 0.4678571428571428603, 0.4714285714285714191, 0.4749999999999999223, 0.4785714285714284810, 0.4821428571428570398 ),
 .UNSPECIFIED. ) 
 CURVE ( )  GEOMETRIC_REPRESENTATION_ITEM ( )  RATIONAL_B_SPLINE_CURVE ( ( 1.000000000000000000, 0.9510565162951534202, 1.000000000000000000, 0.9510565162951534202, 1.000000000000000000, 0.9510565162951534202, 1.000000000000000000, 0.9510565162951534202, 1.000000000000000000, 0.9510565162951541973, 0.9999999999999992228 ) ) 
 REPRESENTATION_ITEM ( '' )  );
#22494=CARTESIAN_POINT ( 'NONE',  ( 55.87499999726882294, 171.3844434931184253, -7.942151717890134290E-15 ) ) ;
#22497=CARTESIAN_POINT ( 'NONE',  ( 117.5000000000000142, 155.0000000000000000, -6.938893903907228378E-15 ) ) ;
#22498=CARTESIAN_POINT ( 'NONE',  ( 57.51132485994281041, 146.1832212156128890, -12.13525491562423042 ) ) ;
#22500=CARTESIAN_POINT ( 'NONE',  ( 68.17499999726881299, 164.1591823560292198, 12.60653300113718167 ) ) ;
#22506=CARTESIAN_POINT ( 'NONE',  ( 82.30000000000001137, 146.4771138417591203, -11.73074641843674470 ) ) ;
#22508=LINE ( 'NONE', #27955, #15310 ) ;
#22511=CARTESIAN_POINT ( 'NONE',  ( 48.37499999726880873, 155.0000000000000000, 15.58253174999999402 ) ) ;
#22514=CARTESIAN_POINT ( 'NONE',  ( 82.12499999726881583, 155.0000000000000000, 15.58253174999999402 ) ) ;
#22518=CARTESIAN_POINT ( 'NONE',  ( 48.79999999453762882, 163.5228861582408797, 11.73074641843673049 ) ) ;
#22526=CARTESIAN_POINT ( 'NONE',  ( 65.91132485994280898, 163.8167787843871110, -12.13525491562423397 ) ) ;
#22533=ORIENTED_EDGE ( 'NONE', *, *, #20796, .T. ) ;
#22537=CARTESIAN_POINT ( 'NONE',  ( 39.97499999726881015, 169.8198683612136222, 4.815267126137181997 ) ) ;
#22539=CARTESIAN_POINT ( 'NONE',  ( 46.02499999726880731, 160.0630714827496206, 15.58253174999999402 ) ) ;
#22544=CARTESIAN_POINT ( 'NONE',  ( 48.97499999726881725, 140.1801316387863778, -4.815267126137194431 ) ) ;
#22548=CARTESIAN_POINT ( 'NONE',  ( 59.40000000000000568, 159.7113355953771077, 14.49999999999999289 ) ) ;
#22555=CARTESIAN_POINT ( 'NONE',  ( 67.32499999726881867, 164.1591823560292198, -12.60653300113719766 ) ) ;
#22557=ORIENTED_EDGE ( 'NONE', *, *, #14492, .F. ) ;
#22559=CARTESIAN_POINT ( 'NONE',  ( 80.87499999726881583, 138.6155565068815463, -3.929120461958505118E-15 ) ) ;
#22566=CARTESIAN_POINT ( 'NONE',  ( 32.50000000000000000, 155.0000000000000000, -15.00000000000002487 ) ) ;
#22571=ORIENTED_EDGE ( 'NONE', *, *, #8545, .F. ) ;
#22578=CARTESIAN_POINT ( 'NONE',  ( 76.52499999726880731, 140.1801316387863778, 4.815267126137185549 ) ) ;
#22579=CARTESIAN_POINT ( 'NONE',  ( 32.50000000000000000, 155.0000000000000000, -6.938893903907228378E-15 ) ) ;
#22582=CARTESIAN_POINT ( 'NONE',  ( 44.29999999999999716, 146.4771138417591203, -11.73074641843674470 ) ) ;
#22584=CYLINDRICAL_SURFACE ( 'NONE', #28456, 15.00000000000001776 ) ;
#22587=CARTESIAN_POINT ( 'NONE',  ( 49.52499999726880731, 169.8198683612136222, -4.815267126137197984 ) ) ;
#22588=CARTESIAN_POINT ( 'NONE',  ( 61.77499999726881441, 169.8198683612136222, -4.815267126137197984 ) ) ;
#22595=CARTESIAN_POINT ( 'NONE',  ( 127.5000000000000000, 261.0000000000000000, 0.000000000000000000 ) ) ;
#22599=EDGE_CURVE ( 'NONE', #534, #19849, #24820, .T. ) ;
#22604=VERTEX_POINT ( 'NONE', #1730 ) ;
#22605=CARTESIAN_POINT ( 'NONE',  ( 75.17499999726881299, 145.8408176439707802, -12.60653300113719588 ) ) ;
#22609=CARTESIAN_POINT ( 'NONE',  ( 84.37499999726881583, 155.0000000000000000, 15.58253174999999402 ) ) ;
#22612=CARTESIAN_POINT ( 'NONE',  ( 55.92499999726881299, 164.1591823560292198, 12.60653300113718167 ) ) ;
#22613=DIRECTION ( 'NONE',  ( 0.000000000000000000, 0.000000000000000000, -1.000000000000000000 ) ) ;
#22615=ORIENTED_EDGE ( 'NONE', *, *, #22678, .F. ) ;
#22624=CARTESIAN_POINT ( 'NONE',  ( 49.62499999726880873, 171.3844434931184253, -7.942151717890132712E-15 ) ) ;
#22628=CARTESIAN_POINT ( 'NONE',  ( 32.50000000000000000, 155.0000000000000000, -15.00000000000002487 ) ) ;
#22629=ADVANCED_FACE ( 'NONE', ( #6848 ), #27795, .T. ) ;
#22638=CARTESIAN_POINT ( 'NONE',  ( 72.99999999453763166, 155.0000000000000000, 14.49999999999999467 ) ) ;
#22648=ORIENTED_EDGE ( 'NONE', *, *, #30401, .F. ) ;
#22651=CARTESIAN_POINT ( 'NONE',  ( 58.78867513459481842, 155.0000000000000000, -15.00000000000002487 ) ) ;
#22658=CARTESIAN_POINT ( 'NONE',  ( 54.57499999726881157, 145.8408176439707802, 12.60653300113718345 ) ) ;
#22661=DIRECTION ( 'NONE',  ( -1.000000000000000000, 0.000000000000000000, 0.000000000000000000 ) ) ;
#22665=CARTESIAN_POINT ( 'NONE',  ( 65.77499999726880731, 169.8198683612136222, -4.815267126137197984 ) ) ;
#22667=CARTESIAN_POINT ( 'NONE',  ( 127.5000000000000000, 80.04668119422552763, -74.95331880577366235 ) ) ;
#22672=CARTESIAN_POINT ( 'NONE',  ( 81.39999999999999147, 159.7113355953771077, 14.49999999999999289 ) ) ;
#22676=CARTESIAN_POINT ( 'NONE',  ( 48.58867513459482268, 146.1832212156128890, -12.13525491562423042 ) ) ;
#22677=CARTESIAN_POINT ( 'NONE',  ( 47.87499999726880162, 171.3844434931184253, -7.942151717890132712E-15 ) ) ;
#22678=EDGE_CURVE ( 'NONE', #10286, #8044, #9918, .T. ) ;
#22681=CARTESIAN_POINT ( 'NONE',  ( 82.62499999726881583, 138.6155565068815463, -3.929120461958505118E-15 ) ) ;
#22682=CARTESIAN_POINT ( 'NONE',  ( 41.71132485994280614, 155.0000000000000000, -15.00000000000002487 ) ) ;
#22684=CARTESIAN_POINT ( 'NONE',  ( 52.99999999453762456, 155.0000000000000000, 14.49999999999999467 ) ) ;
#22687=DIRECTION ( 'NONE',  ( 1.000000000000000000, 0.000000000000000000, 0.000000000000000000 ) ) ;
#22697=DIRECTION ( 'NONE',  ( 0.000000000000000000, 0.000000000000000000, -1.000000000000000000 ) ) ;
#22701=EDGE_CURVE ( 'NONE', #33266, #17976, #23027, .T. ) ;
#22704=CARTESIAN_POINT ( 'NONE',  ( 37.07499999726881157, 141.7447067706911810, -9.630534252274387086 ) ) ;
#22707=CARTESIAN_POINT ( 'NONE',  ( 43.12499999726881583, 155.0000000000000000, -15.58253175000000823 ) ) ;
#22708=CARTESIAN_POINT ( 'NONE',  ( 38.78867513459481842, 155.0000000000000000, -15.00000000000002487 ) ) ;
#22711=CARTESIAN_POINT ( 'NONE',  ( 44.47499999726879594, 149.9369285172503510, 15.58253174999999580 ) ) ;
#22716=CARTESIAN_POINT ( 'NONE',  ( 60.00000000000000000, 139.7537977485451393, -4.138211985947621020E-15 ) ) ;
#22718=LINE ( 'NONE', #7217, #26726 ) ;
#22723=EDGE_CURVE ( 'NONE', #3615, #20973, #13284, .T. ) ;
#22726=CARTESIAN_POINT ( 'NONE',  ( 66.12499999726881583, 155.0000000000000000, 15.58253174999999402 ) ) ;
#22728=EDGE_LOOP ( 'NONE', ( #18753, #29066, #20052, #17942 ) ) ;
#22730=CARTESIAN_POINT ( 'NONE',  ( 81.47499999726879594, 160.0630714827496206, -15.58253175000000823 ) ) ;
#22732=CARTESIAN_POINT ( 'NONE',  ( 72.48867513459484258, 142.2402378747194405, -9.270509831248439525 ) ) ;
#22752=CARTESIAN_POINT ( 'NONE',  ( 73.37499999726881583, 155.0000000000000000, -15.58253175000000823 ) ) ;
#22753=CARTESIAN_POINT ( 'NONE',  ( 79.82499999726881867, 168.2552932293087906, 9.630534252274372875 ) ) ;
#22759=CARTESIAN_POINT ( 'NONE',  ( 39.20000000000000284, 167.3344367211045096, 8.961492836873468093 ) ) ;
#22764=CARTESIAN_POINT ( 'NONE',  ( 56.12499999726880873, 155.0000000000000000, 15.58253174999999402 ) ) ;
#22765=CARTESIAN_POINT ( 'NONE',  ( 65.67499999726881299, 168.2552932293087906, -9.630534252274385310 ) ) ;
#22767=CARTESIAN_POINT ( 'NONE',  ( 46.11132485994280472, 169.2658477444273331, -4.635254915624224203 ) ) ;
#22783=EDGE_LOOP ( 'NONE', ( #22478, #32697, #27982, #16404 ) ) ;
#22784=CARTESIAN_POINT ( 'NONE',  ( 79.17499999726881299, 145.8408176439707802, -12.60653300113719588 ) ) ;
#22787=CARTESIAN_POINT ( 'NONE',  ( 68.32499999726881867, 145.8408176439707802, 12.60653300113718345 ) ) ;
#22791=CARTESIAN_POINT ( 'NONE',  ( 63.42499999726881299, 168.2552932293087906, -9.630534252274385310 ) ) ;
#22794=ORIENTED_EDGE ( 'NONE', *, *, #14090, .F. ) ;
#22798=CARTESIAN_POINT ( 'NONE',  ( 86.01132485994283172, 167.7597621252805880, -9.270509831248443078 ) ) ;
#22801=CARTESIAN_POINT ( 'NONE',  ( 32.50000000000000000, 155.0000000000000000, -6.938893903907228378E-15 ) ) ;
#22807=CARTESIAN_POINT ( 'NONE',  ( 37.12499999726881583, 155.0000000000000000, -15.58253175000000823 ) ) ;
#22813=CARTESIAN_POINT ( 'NONE',  ( 34.88867513459481984, 159.8737954434937478, -14.99999999999993072 ) ) ;
#22816=CARTESIAN_POINT ( 'NONE',  ( 70.19999999453763451, 163.5228861582408797, -11.73074641843674470 ) ) ;
#22817=ORIENTED_EDGE ( 'NONE', *, *, #32617, .T. ) ;
#22823=ORIENTED_EDGE ( 'NONE', *, *, #6664, .F. ) ;
#22832=CARTESIAN_POINT ( 'NONE',  ( 57.37499999726880873, 155.0000000000000000, -15.58253175000000823 ) ) ;
#22838=CARTESIAN_POINT ( 'NONE',  ( 67.27499999726879309, 149.9369285172503510, -15.58253175000000823 ) ) ;
#22845=CARTESIAN_POINT ( 'NONE',  ( 85.20000000000000284, 167.3344367211045096, 8.961492836873468093 ) ) ;
#22850=CARTESIAN_POINT ( 'NONE',  ( 53.37499999726881583, 155.0000000000000000, -15.58253175000000823 ) ) ;
#22852=CARTESIAN_POINT ( 'NONE',  ( 84.82499999726880446, 141.7447067706911810, -9.630534252274385310 ) ) ;
#22853=ADVANCED_FACE ( 'NONE', ( #18257 ), #10098, .F. ) ;
#22856=CARTESIAN_POINT ( 'NONE',  ( 54.19999999453763451, 163.5228861582408797, -11.73074641843674470 ) ) ;
#22859=CARTESIAN_POINT ( 'NONE',  ( 61.61132485994281893, 150.1262045565064227, -15.00000000000002665 ) ) ;
#22868=CARTESIAN_POINT ( 'NONE',  ( 125.5000000000000000, 152.8500000000011028, 106.0000000000000426 ) ) ;
#22869=ORIENTED_EDGE ( 'NONE', *, *, #17904, .T. ) ;
#22874=CARTESIAN_POINT ( 'NONE',  ( 36.97499999726881015, 140.1801316387863778, -4.815267126137194431 ) ) ;
#22876=CARTESIAN_POINT ( 'NONE',  ( 44.02499999726881441, 160.0630714827496206, 15.58253174999999402 ) ) ;
#22878=CARTESIAN_POINT ( 'NONE',  ( 54.01132485994280330, 167.7597621252805880, -9.270509831248443078 ) ) ;
#22880=CARTESIAN_POINT ( 'NONE',  ( 44.67499999726881299, 141.7447067706911810, 9.630534252274376428 ) ) ;
#22884=CARTESIAN_POINT ( 'NONE',  ( 67.80000000000001137, 142.6655632788954620, 8.961492836873471646 ) ) ;
#22886=DIRECTION ( 'NONE',  ( -1.000000000000000000, 0.000000000000000000, 0.000000000000000000 ) ) ;
#22888=FACE_OUTER_BOUND ( 'NONE', #23291, .T. ) ;
#22889=CARTESIAN_POINT ( 'NONE',  ( 34.57499999726881157, 145.8408176439707802, 12.60653300113718345 ) ) ;
#22891=CARTESIAN_POINT ( 'NONE',  ( 62.22499999726881725, 149.9369285172503510, 15.58253174999999580 ) ) ;
#22893=ORIENTED_EDGE ( 'NONE', *, *, #11675, .T. ) ;
#22895=CARTESIAN_POINT ( 'NONE',  ( 87.37499999726880162, 155.0000000000000000, -15.58253175000000823 ) ) ;
#22905=CARTESIAN_POINT ( 'NONE',  ( 65.88867513459484826, 150.1262045565062806, 14.99999999999992006 ) ) ;
#22913=VERTEX_POINT ( 'NONE', #2424 ) ;
#22915=CYLINDRICAL_SURFACE ( 'NONE', #17315, 112.0000000000000711 ) ;
#22918=CARTESIAN_POINT ( 'NONE',  ( 79.62499999726881583, 171.3844434931184253, -7.942151717890132712E-15 ) ) ;
#22919=FACE_BOUND ( 'NONE', #18225, .T. ) ;
#22923=CARTESIAN_POINT ( 'NONE',  ( 40.79999999999999716, 167.3344367211045096, -8.961492836873482304 ) ) ;
#22928=CARTESIAN_POINT ( 'NONE',  ( 55.22499999726880304, 160.0630714827496206, -15.58253175000000823 ) ) ;
#22929=CARTESIAN_POINT ( 'NONE',  ( 71.67499999726881299, 168.2552932293087906, -9.630534252274385310 ) ) ;
#22931=FACE_BOUND ( 'NONE', #17755, .T. ) ;
#22941=EDGE_CURVE ( 'NONE', #20617, #29364, #15869, .T. ) ;
#22946=AXIS2_PLACEMENT_3D ( 'NONE', #3105, #26605, #3602 ) ;
#22949=CARTESIAN_POINT ( 'NONE',  ( 80.27499999726879309, 160.0630714827496206, 15.58253174999999402 ) ) ;
#22952=CARTESIAN_POINT ( 'NONE',  ( 69.62499999726881583, 171.3844434931184253, -7.942151717890134290E-15 ) ) ;
#22956=CARTESIAN_POINT ( 'NONE',  ( 62.92499999726880588, 145.8408176439707802, -12.60653300113719588 ) ) ;
#22965=DIRECTION ( 'NONE',  ( 0.000000000000000000, -1.000000000000000000, 0.000000000000000000 ) ) ;
#22971=CARTESIAN_POINT ( 'NONE',  ( 36.62499999726881583, 138.6155565068815747, -3.929120461958505118E-15 ) ) ;
#22979=CARTESIAN_POINT ( 'NONE',  ( 75.89999999453763735, 150.2886644046228639, -14.50000000000000888 ) ) ;
#22989=VERTEX_POINT ( 'NONE', #29311 ) ;
#22991=ADVANCED_FACE ( 'NONE', ( #31858 ), #24363, .T. ) ;
#22992=LINE ( 'NONE', #10064, #6962 ) ;
#22999=CARTESIAN_POINT ( 'NONE',  ( 57.57499999726881157, 164.1591823560292198, -12.60653300113719766 ) ) ;
#23000=ORIENTED_EDGE ( 'NONE', *, *, #16996, .F. ) ;
#23002=CARTESIAN_POINT ( 'NONE',  ( 68.48867513459484258, 142.2402378747194405, -9.270509831248439525 ) ) ;
#23004=CARTESIAN_POINT ( 'NONE',  ( 57.41132485994281609, 142.2402378747194405, -9.270509831248439525 ) ) ;
#23007=CARTESIAN_POINT ( 'NONE',  ( 66.97499999726881015, 140.1801316387863778, -4.815267126137194431 ) ) ;
#23012=CARTESIAN_POINT ( 'NONE',  ( 87.10000000000000853, 168.7903194862797420, 4.480746418436729606 ) ) ;
#23016=CARTESIAN_POINT ( 'NONE',  ( 47.97499999726881015, 169.8198683612136222, 4.815267126137181997 ) ) ;
#23020=CARTESIAN_POINT ( 'NONE',  ( 33.12499999726880873, 155.0000000000000000, -15.58253175000000823 ) ) ;
#23022=CARTESIAN_POINT ( 'NONE',  ( 56.99999999453763166, 155.0000000000000000, 14.49999999999999467 ) ) ;
#23025=CARTESIAN_POINT ( 'NONE',  ( 37.48867513459482836, 167.7597621252805880, 9.270509831248428867 ) ) ;
#23027=LINE ( 'NONE', #20132, #27545 ) ;
#23028=ORIENTED_EDGE ( 'NONE', *, *, #629, .T. ) ;
#23040=CARTESIAN_POINT ( 'NONE',  ( 37.27499999726880731, 149.9369285172503510, -15.58253175000000823 ) ) ;
#23042=CARTESIAN_POINT ( 'NONE',  ( 42.62499999726881583, 138.6155565068815463, -3.929120461958505118E-15 ) ) ;
#23044=EDGE_CURVE ( 'NONE', #18472, #19014, #26129, .T. ) ;
#23049=CARTESIAN_POINT ( 'NONE',  ( 44.07499999726881157, 168.2552932293087906, 9.630534252274372875 ) ) ;
#23055=CARTESIAN_POINT ( 'NONE',  ( 69.40000000000001990, 159.7113355953771077, 14.49999999999999289 ) ) ;
#23062=CARTESIAN_POINT ( 'NONE',  ( 72.72499999726881015, 140.1801316387863778, -4.815267126137194431 ) ) ;
#23065=CARTESIAN_POINT ( 'NONE',  ( 35.79999999453762882, 146.4771138417591203, -11.73074641843674470 ) ) ;
#23067=EDGE_CURVE ( 'NONE', #7672, #3615, #7828, .T. ) ;
#23078=AXIS2_PLACEMENT_3D ( 'NONE', #14964, #4065, #1347 ) ;
#23082=( BOUNDED_CURVE ( )  B_SPLINE_CURVE ( 2, ( #1806, #4029, #12203, #32309, #29756, #27199, #3855, #14247, #28561, #15595, #12541 ),
 .UNSPECIFIED., .F., .T. ) 
 B_SPLINE_CURVE_WITH_KNOTS ( ( 3, 2, 2, 2, 2, 3 ),
 ( 0.1249999999999999722, 0.1285714285714285310, 0.1321428571428571175, 0.1357142857142857040, 0.1392857142857142905, 0.1428571428571428492 ),
 .UNSPECIFIED. ) 
 CURVE ( )  GEOMETRIC_REPRESENTATION_ITEM ( )  RATIONAL_B_SPLINE_CURVE ( ( 1.000000000000000444, 0.9510565162951530871, 1.000000000000000000, 0.9510565162951534202, 1.000000000000000000, 0.9510565162951534202, 1.000000000000000000, 0.9510565162951534202, 1.000000000000000000, 0.9510565162951534202, 1.000000000000000000 ) ) 
 REPRESENTATION_ITEM ( '' )  );
#23086=ORIENTED_EDGE ( 'NONE', *, *, #5025, .T. ) ;
#23088=EDGE_CURVE ( 'NONE', #10286, #7343, #16760, .T. ) ;
#23090=CARTESIAN_POINT ( 'NONE',  ( 84.62499999726880162, 138.6155565068815463, -3.929120461958505118E-15 ) ) ;
#23093=DIRECTION ( 'NONE',  ( 0.000000000000000000, 0.000000000000000000, 1.000000000000000000 ) ) ;
#23095=CARTESIAN_POINT ( 'NONE',  ( 50.60000000000000142, 159.7113355953771077, -14.50000000000000888 ) ) ;
#23097=CARTESIAN_POINT ( 'NONE',  ( 67.58867513459482268, 163.8167787843871110, 12.13525491562421621 ) ) ;
#23103=CARTESIAN_POINT ( 'NONE',  ( 58.82499999726881867, 141.7447067706911810, -9.630534252274387086 ) ) ;
#23104=CARTESIAN_POINT ( 'NONE',  ( 71.97499999726881015, 169.8198683612136222, 4.815267126137181997 ) ) ;
#23106=FACE_BOUND ( 'NONE', #32161, .T. ) ;
#23117=EDGE_LOOP ( 'NONE', ( #28574, #12091, #19491, #21553 ) ) ;
#23121=CARTESIAN_POINT ( 'NONE',  ( 80.37499999726881583, 155.0000000000000000, 15.58253174999999402 ) ) ;
#23124=CARTESIAN_POINT ( 'NONE',  ( 73.12499999726881583, 155.0000000000000000, -15.58253175000000823 ) ) ;
#23127=CARTESIAN_POINT ( 'NONE',  ( 64.72499999726881015, 140.1801316387863778, -4.815267126137194431 ) ) ;
#23128=ADVANCED_FACE ( 'NONE', ( #4420 ), #24534, .T. ) ;
#23130=EDGE_CURVE ( 'NONE', #27498, #25537, #33082, .T. ) ;
#23146=CARTESIAN_POINT ( 'NONE',  ( 40.22499999726881015, 149.9369285172503510, 15.58253174999999580 ) ) ;
#23154=CARTESIAN_POINT ( 'NONE',  ( 75.69999999453764872, 142.6655632788954620, -8.961492836873480528 ) ) ;
#23160=CARTESIAN_POINT ( 'NONE',  ( 70.71132485994280614, 155.0000000000000000, 15.00000000000001243 ) ) ;
#23167=VERTEX_POINT ( 'NONE', #19253 ) ;
#23172=CARTESIAN_POINT ( 'NONE',  ( 62.37499999726880873, 155.0000000000000000, 15.58253174999999402 ) ) ;
#23178=CYLINDRICAL_SURFACE ( 'NONE', #29589, 15.00000000000001776 ) ;
#23182=CARTESIAN_POINT ( 'NONE',  ( 34.32499999726881157, 145.8408176439707802, 12.60653300113718345 ) ) ;
#23187=CARTESIAN_POINT ( 'NONE',  ( 51.17499999726880588, 145.8408176439707802, -12.60653300113719588 ) ) ;
#23191=CARTESIAN_POINT ( 'NONE',  ( 78.21132485994282035, 170.7719333635740497, -7.904646289410545231E-15 ) ) ;
#23192=CARTESIAN_POINT ( 'NONE',  ( 65.21132485994280614, 139.2280666364260071, -4.041636747397287284E-15 ) ) ;
#23193=CARTESIAN_POINT ( 'NONE',  ( 53.49999999453762456, 139.7537977485451393, -4.138211985947621020E-15 ) ) ;
#23196=DIRECTION ( 'NONE',  ( 0.000000000000000000, 0.000000000000000000, -1.000000000000000000 ) ) ;
#23198=CARTESIAN_POINT ( 'NONE',  ( 60.51132485994280330, 163.8167787843871110, 12.13525491562421621 ) ) ;
#23203=ORIENTED_EDGE ( 'NONE', *, *, #21211, .F. ) ;
#23205=CARTESIAN_POINT ( 'NONE',  ( 80.48867513459481415, 142.2402378747194405, -9.270509831248439525 ) ) ;
#23206=CARTESIAN_POINT ( 'NONE',  ( 77.17499999726881299, 145.8408176439707802, -12.60653300113719588 ) ) ;
#23209=VECTOR ( 'NONE', #12807, 1000.000000000000000 ) ;
#23211=CARTESIAN_POINT ( 'NONE',  ( 34.37499999726881583, 155.0000000000000000, 15.58253174999999402 ) ) ;
#23212=ORIENTED_EDGE ( 'NONE', *, *, #6640, .F. ) ;
#23213=CARTESIAN_POINT ( 'NONE',  ( 42.72499999726881015, 140.1801316387863778, -4.815267126137194431 ) ) ;
#23216=CARTESIAN_POINT ( 'NONE',  ( 48.77499999726880731, 140.1801316387863778, 4.815267126137185549 ) ) ;
#23219=LINE ( 'NONE', #17950, #31211 ) ;
#23221=CARTESIAN_POINT ( 'NONE',  ( 69.09999999999999432, 168.7903194862797420, 4.480746418436729606 ) ) ;
#23229=CARTESIAN_POINT ( 'NONE',  ( 69.32499999726881867, 164.1591823560292198, -12.60653300113719766 ) ) ;
#23231=CARTESIAN_POINT ( 'NONE',  ( 43.41132485994280898, 142.2402378747194405, -9.270509831248439525 ) ) ;
#23232=CARTESIAN_POINT ( 'NONE',  ( 87.77499999726882152, 169.8198683612136222, -4.815267126137197984 ) ) ;
#23237=AXIS2_PLACEMENT_3D ( 'NONE', #13640, #29150, #10935 ) ;
#23249=ORIENTED_EDGE ( 'NONE', *, *, #22941, .F. ) ;
#23254=CARTESIAN_POINT ( 'NONE',  ( 82.62499999726881583, 138.6155565068815463, -3.929120461958505118E-15 ) ) ;
#23261=CARTESIAN_POINT ( 'NONE',  ( 48.50000000000000000, 155.0000000000000000, -14.50000000000000711 ) ) ;
#23264=AXIS2_PLACEMENT_3D ( 'NONE', #32220, #19444, #720 ) ;
#23265=CARTESIAN_POINT ( 'NONE',  ( 49.12499999726880873, 155.0000000000000000, -15.58253175000000823 ) ) ;
#23268=CARTESIAN_POINT ( 'NONE',  ( 60.12499999726880873, 155.0000000000000000, 15.58253174999999402 ) ) ;
#23269=CARTESIAN_POINT ( 'NONE',  ( 67.57499999726881867, 164.1591823560292198, -12.60653300113719766 ) ) ;
#23271=FACE_OUTER_BOUND ( 'NONE', #25204, .T. ) ;
#23274=EDGE_CURVE ( 'NONE', #31983, #32748, #15491, .T. ) ;
#23279=( BOUNDED_SURFACE ( )  B_SPLINE_SURFACE ( 1, 2, ( 
 ( #24636, #31793, #13728, #27016, #16621, #8789, #29409, #23963, #3511, #3846, #24127, #796, #32460, #1303, #29580, #13903, #11521, #626, #11693, #27190, #11185, #14238, #31957, #21564, #24287, #11024, #14068, #957, #13572, #26849, #29244, #3677, #5894, #29745, #19525, #3341, #21902, #8625, #21405, #8460, #19021, #24466, #16290, #32299, #22074, #26680, #16790, #9128, #11354, #19185, #29921, #6059, #21737, #32127, #6232, #8960, #19351, #16451, #6409, #6575, #26511, #3180, #30766, #9467, #17469, #20194, #11859, #22759, #19855, #4020, #9633, #15082, #22243, #4181, #27854, #7087, #32967, #30252, #14412, #27692, #28030, #14576, #24976, #22923, #25477, #20029, #4356, #1971, #24805, #2149, #17643, #1629, #4692, #22408, #12021, #14740, #1462, #12533, #32799, #25307, #20373, #6914, #17306, #14917, #33316, #17135, #16959, #30428, #9295, #25132, #12362, #27353, #9986, #1795, #4526, #32633, #33151, #12195, #22582, #19689, #9815, #30081, #6746, #27521, #30595, #7259, #17810, #12699, #5367, #18315, #4865, #15917, #422, #30940, #2982, #26315, #15254, #21033, #20876, #10496, #31275, #13200, #2657, #28708, #7935, #10152, #15754, #7603, #18486, #25647, #25821, #26150, #2485, #20535, #28869, #21198, #28208, #5527, #12867, #7425, #23261, #18157, #13362, #2314, #17986, #2817, #28378, #5035, #10659, #23600, #265, #15425, #13040, #7766, #33655, #10332, #23431, #20704, #31434, #28552, #33484, #23095, #8104, #95, #23757, #10824, #31104, #5198, #15583, #25986, #32092, #11154, #32255, #19313, #31593, #13864, #26973, #11654, #24086, #5855, #3143, #21862, #16254, #3471, #29376, #29702, #1259, #754, #31757, #6360, #18986, #13531, #6021, #21528, #3302, #23922, #8259, #8754, #31917, #16412, #27154, #8589, #26807, #24250, #29203, #29538, #917, #24598, #8424, #26640, #16755, #8922, #19142, #587, #10982, #11316, #21701, #14201, #6194, #3636, #24429, #1092, #18810, #16583, #14032, #18649, #11484, #29040, #3811, #5693, #16082, #13686, #26474, #21360, #30387, #1933, #14534, #32932, #30217, #7215, #22369, #9085, #4483, #17431, #27651, #20155, #15043, #4318, #12322, #22548, #9592, #19822, #19653, #6873, #17602, #22716, #32420, #7050, #11816, #27993, #24936, #17101, #9772, #25435, #1593, #22205, #30552, #9430, #3978, #17261, #11983, #27486, #27315, #2111, #19986, #32758, #14703, #4659, #25095, #1755, #12154, #30043, #27815, #14874, #22037, #32594, #6709, #19483, #33106, #25268, #14377, #24768, #29884, #6538, #16918, #1424, #9260, #4141, #15718, #12657, #13004, #5162, #15882, #31235, #12495, #20673, #5326, #60, #7566, #18279, #13165, #20832, #26117, #4997, #23396, #31070, #31396, #12829, #33276, #28668, #7898, #18114, #10623, #5493, #28512, #2785, #10457, #23559, #10297, #10118, #7728, #8064, #229, #22884, #20998, #2273, #18450, #15385, #17952, #28837, #26277, #9943, #20329, #30900, #30729, #28342, #23221, #7389, #17770, #23055, #28166, #33447, #20499, #4826, #15217, #25608, #25781, #15549, #33616, #2449, #25942, #2616, #16212, #16374, #13654, #29000, #18613, #19109, #31882, #29498, #3431, #23720, #21825, #6152, #16546, #13828, #26603, #3600, #24390, #2948, #18942, #32056, #16714, #29165, #10947, #8224, #26941, #21322, #8549, #716, #29339, #1057, #29669, #5986, #13994, #24218, #882, #11119, #554, #21495, #32216, #11446, #13329, #11278, #26438, #8881, #5817, #31719, #19277, #383, #10785, #6321, #8391, #21160, #18778, #24047, #31557, #5660, #3103, #21661, #3266, #8718, #16048, #13491, #23886, #26766, #17393, #12280, #4102, #19782, #9728, #6667, #14494, #32719, #24892, #25062, #1552, #30006, #9553, #14334, #27779, #30177, #7176, #19615, #27607, #30344, #22001, #32893, #17054, #14164, #6834, #25230, #32384, #24731, #4274, #17220, #9386, #27448, #24558, #11950, #4443, #1385, #11773, #33059, #1893, #14667, #22332, #12115, #1214, #22672, #14831, #22163, #20118, #32550, #9225, #1715, #11611, #30511, #22506, #19945, #27115, #7007, #3777, #9048, #19440, #27278, #29843, #6503, #16881, #3935, #12963, #20961, #2750, #7524, #10255, #15004, #23358, #15176, #17909, #28631, #20460, #10583, #26080, #31354, #30691, #18072, #27953, #22845, #15512, #28467, #25394, #13124, #17560, #7354, #23517, #185, #2066, #31191, #4622, #10083, #17734, #15679, #4957, #33237, #15344, #30860, #23012, #9903, #12453, #5124, #28302 ),
 ( #20285, #25735, #21, #28122, #4783, #2406, #20631, #25569, #10418, #2233, #12792, #5286, #23182, #12617, #33409, #33576, #31031, #25904, #7689, #2576, #20790, #7857, #18242, #16503, #1010, #31520, #3560, #26902, #5456, #21616, #21457, #11076, #31839, #13784, #3226, #29292, #8504, #10742, #18897, #8190, #19066, #15843, #26401, #16334, #3060, #21123, #5943, #16168, #28800, #8350, #340, #26728, #18575, #11229, #11405, #28960, #3389, #8023, #13449, #23843, #18739, #24180, #26232, #841, #29455, #5617, #32011, #13950, #29125, #674, #24341, #21286, #5772, #13614, #26557, #8674, #24010, #10909, #6106, #16009, #21783, #18408, #2903, #516, #13289, #23680, #31680, #4229, #24687, #19236, #24848, #30298, #3730, #19398, #32676, #22294, #14453, #1346, #29631, #14119, #14627, #27402, #25023, #9342, #6278, #17355, #1676, #12069, #19737, #11733, #32849, #19899, #32174, #1512, #27563, #12238, #22120, #6460, #24513, #22457, #16841, #4064, #29965, #6966, #1848, #32511, #32345, #27740, #19572, #1171, #6623, #9183, #3889, #11567, #8834, #30133, #17008, #11909, #4403, #6791, #17179, #9512, #29799, #14788, #25180, #16671, #9009, #27235, #27068, #21955, #14284, #28381, #25825, #26154, #28715, #5696, #7938, #28874, #15921, #26319, #23265, #23603, #15759, #26478, #8108, #22624, #31278, #2985, #10662, #18160, #5530, #23760, #31441, #13365, #15588, #268, #18320, #8263, #23434, #9683, #426, #18491, #5371, #21203, #16085, #2820, #10828, #21037, #31598, #20879, #20707, #13204, #18653, #29043, #33012, #3147, #12872, #20077, #25991, #28555, #30472, #7134, #17518, #5039, #7770, #15428, #5203, #98, #2489, #33660, #10336, #31108, #2661, #13044, #10501, #11489, #6369, #3306, #8757, #13868, #8593, #758, #19146, #26813, #26978, #24253, #5859, #921, #29207, #11320, #3475, #18989, #18813, #27320, #14037, #21704, #32095, #9092, #29544, #6198, #16586, #11157, #21867, #3642, #6543, #13690, #31922, #11659, #14206, #1098, #16257, #26643, #24434, #32261, #29889, #8928, #19319, #16761, #27159, #24091, #29708, #3815, #16925, #24603, #13534, #1266, #22043, #32426, #29379, #19489, #23928, #591, #10986, #6024, #21365, #31760, #8427, #21532, #16416, #20163, #33114, #9601, #2120, #30737, #19994, #28000, #4491, #25275, #1762, #1599, #12163, #22891, #4666, #14383, #12329, #27491, #9950, #6879, #32764, #15050, #17777, #24773, #12502, #22375, #3986, #9438, #14709, #33283, #14883, #7222, #25444, #9265, #11990, #17613, #1940, #30560, #4146, #32940, #4325, #19828, #24942, #30395, #17268, #17438, #25102, #30048, #19658, #20338, #7056, #7396, #22726, #1429, #11823, #22211, #32600, #9779, #27658, #6716, #17106, #14541, #27821, #30224, #22555, #20680, #2456, #33454, #18458, #12837, #67, #25950, #15889, #31564, #31078, #28350, #26283, #20840, #8232, #13172, #28176, #2626, #21005, #15727, #23229, #238, #28845, #2792, #8073, #7736, #5335, #13012, #13336, #28520, #15225, #10630, #23569, #10466, #2957, #21169, #31243, #5500, #28675, #26124, #23404, #25791, #7905, #23727, #390, #4835, #31403, #17960, #10794, #18121, #33625, #25614, #2280, #12664, #23062, #10304, #10126, #5169, #15555, #20506, #30909, #7574, #5004, #15392, #18286, #21832, #16554, #11453, #8399, #13836, #18952, #13661, #5825, #24225, #31889, #32065, #29346, #10954, #561, #1065, #888, #32223, #19115, #5668, #3785, #8888, #19284, #29505, #8557, #29676, #6330, #18620, #11285, #14001, #32391, #11127, #26610, #23894, #16721, #3273, #21672, #16381, #27124, #22008, #21502, #18786, #14172, #5993, #21330, #26773, #3438, #24054, #31726, #29007, #6159, #8725, #26949, #24565, #3608, #24400, #1222, #16220, #11620, #16057, #26446, #29175, #725, #3110, #13500, #30351, #14342, #11782, #12122, #14674, #25402, #27614, #14838, #1902, #12288, #9232, #9560, #19622, #27454, #7183, #9736, #7014, #24738, #22170, #22514, #25068, #2073, #4284, #25237, #22681, #33067, #30013, #19954, #1722, #12461, #27786, #9055, #17228, #20124, #17400, #4108, #30518, #17567, #4450, #27960, #1561, #4629, #32902, #15013, #9394, #29852, #22852, #19448, #6510, #16889, #27287, #3942, #1392, #32560, #6675, #6841, #17062, #14501, #24899, #11956, #22339, #32726, #19791, #30185, #2413, #28309, #10592, #13297, #20292, #31363, #17918, #33244, #4965, #10263, #18416, #30, #2756, #194, #4791, #30869 ) ),
 .UNSPECIFIED., .F., .F., .T. ) 
 B_SPLINE_SURFACE_WITH_KNOTS ( ( 2, 2 ),
 ( 3, 2, 2, 2, 2, 2, 2, 2, 2, 2, 2, 2, 2, 2, 2, 2, 2, 2, 2, 2, 2, 2, 2, 2, 2, 2, 2, 2, 2, 2, 2, 2, 2, 2, 2, 2, 2, 2, 2, 2, 2, 2, 2, 2, 2, 2, 2, 2, 2, 2, 2, 2, 2, 2, 2, 2, 2, 2, 2, 2, 2, 2, 2, 2, 2, 2, 2, 2, 2, 2, 2, 2, 2, 2, 2, 2, 2, 2, 2, 2, 2, 2, 2, 2, 2, 2, 2, 2, 2, 2, 2, 2, 2, 2, 2, 2, 2, 2, 2, 2, 2, 2, 2, 2, 2, 2, 2, 2, 2, 2, 2, 2, 2, 2, 2, 2, 2, 2, 2, 2, 2, 2, 2, 2, 2, 2, 2, 2, 2, 2, 2, 2, 2, 2, 2, 2, 2, 2, 2, 2, 2, 2, 2, 2, 2, 2, 2, 2, 2, 2, 2, 2, 2, 2, 2, 2, 2, 2, 2, 2, 2, 2, 2, 2, 2, 2, 2, 2, 2, 2, 2, 2, 2, 2, 2, 2, 2, 2, 2, 2, 2, 2, 2, 2, 2, 2, 2, 2, 2, 2, 2, 2, 2, 2, 2, 2, 2, 2, 2, 2, 2, 2, 2, 2, 2, 2, 2, 2, 2, 2, 2, 2, 2, 2, 2, 2, 2, 2, 2, 2, 2, 2, 2, 2, 2, 2, 2, 2, 2, 2, 2, 2, 2, 2, 2, 2, 2, 2, 2, 2, 2, 2, 2, 2, 2, 2, 2, 2, 2, 2, 2, 2, 2, 2, 2, 2, 2, 2, 2, 2, 2, 2, 2, 2, 2, 2, 2, 2, 2, 2, 2, 2, 2, 2, 2, 3 ),
 ( 0.000000000000000000, 1.000000000000000000 ),
 ( 0.000000000000000000, 0.003571428571428571317, 0.007142857142857142634, 0.01071428571428571438, 0.01428571428571428527, 0.01785714285714285615, 0.02142857142857142877, 0.02500000000000000139, 0.02857142857142857054, 0.03214285714285713969, 0.03571428571428571230, 0.03928571428571428492, 0.04285714285714285754, 0.04642857142857143016, 0.05000000000000000278, 0.05357142857142856845, 0.05714285714285714107, 0.06071428571428571369, 0.06428571428571427937, 0.06785714285714285199, 0.07142857142857142461, 0.07499999999999999722, 0.07857142857142856984, 0.08214285714285714246, 0.08571428571428571508, 0.08928571428571428770, 0.09285714285714286031, 0.09642857142857143293, 0.1000000000000000056, 0.1035714285714285782, 0.1071428571428571369, 0.1107142857142857095, 0.1142857142857142821, 0.1178571428571428548, 0.1214285714285714274, 0.1250000000000000000, 0.1285714285714285587, 0.1321428571428571452, 0.1357142857142857040, 0.1392857142857142905, 0.1428571428571428492, 0.1464285714285714357, 0.1499999999999999944, 0.1535714285714285809, 0.1571428571428571397, 0.1607142857142857262, 0.1642857142857142849, 0.1678571428571428437, 0.1714285714285714302, 0.1749999999999999889, 0.1785714285714285754, 0.1821428571428571341, 0.1857142857142857206, 0.1892857142857142794, 0.1928571428571428659, 0.1964285714285714246, 0.2000000000000000111, 0.2035714285714285698, 0.2071428571428571563, 0.2107142857142857151, 0.2142857142857142738, 0.2178571428571428603, 0.2214285714285714191, 0.2250000000000000056, 0.2285714285714285643, 0.2321428571428571508, 0.2357142857142857095, 0.2392857142857142960, 0.2428571428571428548, 0.2464285714285714413, 0.2500000000000000000, 0.2535714285714285587, 0.2571428571428571175, 0.2607142857142857317, 0.2642857142857142905, 0.2678571428571428492, 0.2714285714285714080, 0.2750000000000000222, 0.2785714285714285809, 0.2821428571428571397, 0.2857142857142856984, 0.2892857142857143127, 0.2928571428571428714, 0.2964285714285714302, 0.2999999999999999889, 0.3035714285714285476, 0.3071428571428571619, 0.3107142857142857206, 0.3142857142857142794, 0.3178571428571428381, 0.3214285714285714524, 0.3250000000000000111, 0.3285714285714285698, 0.3321428571428571286, 0.3357142857142856873, 0.3392857142857143016, 0.3428571428571428603, 0.3464285714285714191, 0.3499999999999999778, 0.3535714285714285920, 0.3571428571428571508, 0.3607142857142857095, 0.3642857142857142683, 0.3678571428571428825, 0.3714285714285714413, 0.3750000000000000000, 0.3785714285714285587, 0.3821428571428571175, 0.3857142857142857317, 0.3892857142857142905, 0.3928571428571428492, 0.3964285714285714080, 0.4000000000000000222, 0.4035714285714285809, 0.4071428571428571397, 0.4107142857142856984, 0.4142857142857143127, 0.4178571428571428714, 0.4214285714285714302, 0.4249999999999999889, 0.4285714285714285476, 0.4321428571428571619, 0.4357142857142857206, 0.4392857142857142794, 0.4428571428571428381, 0.4464285714285714524, 0.4500000000000000111, 0.4535714285714285698, 0.4571428571428571286, 0.4607142857142856873, 0.4642857142857143016, 0.4678571428571428603, 0.4714285714285714191, 0.4749999999999999778, 0.4785714285714285920, 0.4821428571428571508, 0.4857142857142857095, 0.4892857142857142683, 0.4928571428571428825, 0.4964285714285714413, 0.5000000000000000000, 0.5035714285714285587, 0.5071428571428571175, 0.5107142857142856762, 0.5142857142857142350, 0.5178571428571429047, 0.5214285714285714635, 0.5250000000000000222, 0.5285714285714285809, 0.5321428571428571397, 0.5357142857142856984, 0.5392857142857142572, 0.5428571428571428159, 0.5464285714285713746, 0.5500000000000000444, 0.5535714285714286031, 0.5571428571428571619, 0.5607142857142857206, 0.5642857142857142794, 0.5678571428571428381, 0.5714285714285713969, 0.5749999999999999556, 0.5785714285714286254, 0.5821428571428571841, 0.5857142857142857428, 0.5892857142857143016, 0.5928571428571428603, 0.5964285714285714191, 0.5999999999999999778, 0.6035714285714285365, 0.6071428571428570953, 0.6107142857142857650, 0.6142857142857143238, 0.6178571428571428825, 0.6214285714285714413, 0.6250000000000000000, 0.6285714285714285587, 0.6321428571428571175, 0.6357142857142856762, 0.6392857142857142350, 0.6428571428571429047, 0.6464285714285714635, 0.6500000000000000222, 0.6535714285714285809, 0.6571428571428571397, 0.6607142857142856984, 0.6642857142857142572, 0.6678571428571428159, 0.6714285714285713746, 0.6750000000000000444, 0.6785714285714286031, 0.6821428571428571619, 0.6857142857142857206, 0.6892857142857142794, 0.6928571428571428381, 0.6964285714285713969, 0.6999999999999999556, 0.7035714285714286254, 0.7071428571428571841, 0.7107142857142857428, 0.7142857142857143016, 0.7178571428571428603, 0.7214285714285714191, 0.7249999999999999778, 0.7285714285714285365, 0.7321428571428570953, 0.7357142857142857650, 0.7392857142857143238, 0.7428571428571428825, 0.7464285714285714413, 0.7500000000000000000, 0.7535714285714285587, 0.7571428571428571175, 0.7607142857142856762, 0.7642857142857142350, 0.7678571428571429047, 0.7714285714285714635, 0.7750000000000000222, 0.7785714285714285809, 0.7821428571428571397, 0.7857142857142856984, 0.7892857142857142572, 0.7928571428571428159, 0.7964285714285713746, 0.8000000000000000444, 0.8035714285714286031, 0.8071428571428571619, 0.8107142857142857206, 0.8142857142857142794, 0.8178571428571428381, 0.8214285714285713969, 0.8249999999999999556, 0.8285714285714286254, 0.8321428571428571841, 0.8357142857142857428, 0.8392857142857143016, 0.8428571428571428603, 0.8464285714285714191, 0.8499999999999999778, 0.8535714285714285365, 0.8571428571428570953, 0.8607142857142857650, 0.8642857142857143238, 0.8678571428571428825, 0.8714285714285714413, 0.8750000000000000000, 0.8785714285714285587, 0.8821428571428571175, 0.8857142857142856762, 0.8892857142857142350, 0.8928571428571429047, 0.8964285714285714635, 0.9000000000000000222, 0.9035714285714285809, 0.9071428571428571397, 0.9107142857142856984, 0.9142857142857142572, 0.9178571428571428159, 0.9214285714285713746, 0.9250000000000000444, 0.9285714285714286031, 0.9321428571428571619, 0.9357142857142857206, 0.9392857142857142794, 0.9428571428571428381, 0.9464285714285713969, 0.9499999999999999556, 0.9535714285714286254, 0.9571428571428571841, 0.9607142857142857428, 0.9642857142857143016, 0.9678571428571428603, 0.9714285714285714191, 0.9749999999999999778, 0.9785714285714285365, 0.9821428571428570953 ),
 .UNSPECIFIED. ) 
 GEOMETRIC_REPRESENTATION_ITEM ( )  RATIONAL_B_SPLINE_SURFACE ( (
 ( 1.000000000000000000, 0.9510565162951535312, 1.000000000000000000, 0.9510565162951535312, 1.000000000000000000, 0.9510565162951535312, 1.000000000000000000, 0.9510565162951535312, 1.000000000000000000, 0.9510565162951535312, 1.000000000000000000, 0.9510565162951535312, 1.000000000000000000, 0.9510565162951535312, 1.000000000000000000, 0.9510565162951535312, 1.000000000000000000, 0.9510565162951535312, 1.000000000000000000, 0.9510565162951535312, 1.000000000000000000, 0.9510565162951535312, 1.000000000000000000, 0.9510565162951535312, 1.000000000000000000, 0.9510565162951535312, 1.000000000000000000, 0.9510565162951535312, 1.000000000000000000, 0.9510565162951535312, 1.000000000000000000, 0.9510565162951535312, 1.000000000000000000, 0.9510565162951535312, 1.000000000000000000, 0.9510565162951535312, 1.000000000000000000, 0.9510565162951535312, 1.000000000000000000, 0.9510565162951535312, 1.000000000000000000, 0.9510565162951535312, 1.000000000000000000, 0.9510565162951535312, 1.000000000000000000, 0.9510565162951535312, 1.000000000000000000, 0.9510565162951535312, 1.000000000000000000, 0.9510565162951535312, 1.000000000000000000, 0.9510565162951535312, 1.000000000000000000, 0.9510565162951535312, 1.000000000000000000, 0.9510565162951535312, 1.000000000000000000, 0.9510565162951535312, 1.000000000000000000, 0.9510565162951535312, 1.000000000000000000, 0.9510565162951535312, 1.000000000000000000, 0.9510565162951535312, 1.000000000000000000, 0.9510565162951535312, 1.000000000000000000, 0.9510565162951535312, 1.000000000000000000, 0.9510565162951535312, 1.000000000000000000, 0.9510565162951535312, 1.000000000000000000, 0.9510565162951535312, 1.000000000000000000, 0.9510565162951535312, 1.000000000000000000, 0.9510565162951535312, 1.000000000000000000, 0.9510565162951535312, 1.000000000000000000, 0.9510565162951535312, 1.000000000000000000, 0.9510565162951535312, 1.000000000000000000, 0.9510565162951535312, 1.000000000000000000, 0.9510565162951535312, 1.000000000000000000, 0.9510565162951535312, 1.000000000000000000, 0.9510565162951535312, 1.000000000000000000, 0.9510565162951535312, 1.000000000000000000, 0.9510565162951535312, 1.000000000000000000, 0.9510565162951535312, 1.000000000000000000, 0.9510565162951535312, 1.000000000000000000, 0.9510565162951535312, 1.000000000000000000, 0.9510565162951535312, 1.000000000000000000, 0.9510565162951535312, 1.000000000000000000, 0.9510565162951535312, 1.000000000000000000, 0.9510565162951535312, 1.000000000000000000, 0.9510565162951535312, 1.000000000000000000, 0.9510565162951535312, 1.000000000000000000, 0.9510565162951535312, 1.000000000000000000, 0.9510565162951535312, 1.000000000000000000, 0.9510565162951535312, 1.000000000000000000, 0.9510565162951535312, 1.000000000000000000, 0.9510565162951535312, 1.000000000000000000, 0.9510565162951535312, 1.000000000000000000, 0.9510565162951535312, 1.000000000000000000, 0.9510565162951535312, 1.000000000000000000, 0.9510565162951535312, 1.000000000000000000, 0.9510565162951535312, 1.000000000000000000, 0.9510565162951535312, 1.000000000000000000, 0.9510565162951535312, 1.000000000000000000, 0.9510565162951535312, 1.000000000000000000, 0.9510565162951535312, 1.000000000000000000, 0.9510565162951535312, 1.000000000000000000, 0.9510565162951535312, 1.000000000000000000, 0.9510565162951535312, 1.000000000000000000, 0.9510565162951535312, 1.000000000000000000, 0.9510565162951535312, 1.000000000000000000, 0.9510565162951535312, 1.000000000000000000, 0.9510565162951535312, 1.000000000000000000, 0.9510565162951535312, 1.000000000000000000, 0.9510565162951535312, 1.000000000000000000, 0.9510565162951535312, 1.000000000000000000, 0.9510565162951535312, 1.000000000000000000, 0.9510565162951535312, 1.000000000000000000, 0.9510565162951535312, 1.000000000000000000, 0.9510565162951535312, 1.000000000000000000, 0.9510565162951535312, 1.000000000000000000, 0.9510565162951535312, 1.000000000000000000, 0.9510565162951535312, 1.000000000000000000, 0.9510565162951535312, 1.000000000000000000, 0.9510565162951535312, 1.000000000000000000, 0.9510565162951535312, 1.000000000000000000, 0.9510565162951535312, 1.000000000000000000, 0.9510565162951535312, 1.000000000000000000, 0.9510565162951535312, 1.000000000000000000, 0.9510565162951535312, 1.000000000000000000, 0.9510565162951535312, 1.000000000000000000, 0.9510565162951535312, 1.000000000000000000, 0.9510565162951535312, 1.000000000000000000, 0.9510565162951535312, 1.000000000000000000, 0.9510565162951535312, 1.000000000000000000, 0.9510565162951535312, 1.000000000000000000, 0.9510565162951535312, 1.000000000000000000, 0.9510565162951535312, 1.000000000000000000, 0.9510565162951535312, 1.000000000000000000, 0.9510565162951535312, 1.000000000000000000, 0.9510565162951535312, 1.000000000000000000, 0.9510565162951535312, 1.000000000000000000, 0.9510565162951535312, 1.000000000000000000, 0.9510565162951535312, 1.000000000000000000, 0.9510565162951535312, 1.000000000000000000, 0.9510565162951535312, 1.000000000000000000, 0.9510565162951535312, 1.000000000000000000, 0.9510565162951535312, 1.000000000000000000, 0.9510565162951535312, 1.000000000000000000, 0.9510565162951535312, 1.000000000000000000, 0.9510565162951535312, 1.000000000000000000, 0.9510565162951535312, 1.000000000000000000, 0.9510565162951535312, 1.000000000000000000, 0.9510565162951535312, 1.000000000000000000, 0.9510565162951535312, 1.000000000000000000, 0.9510565162951535312, 1.000000000000000000, 0.9510565162951535312, 1.000000000000000000, 0.9510565162951535312, 1.000000000000000000, 0.9510565162951535312, 1.000000000000000000, 0.9510565162951535312, 1.000000000000000000, 0.9510565162951535312, 1.000000000000000000, 0.9510565162951535312, 1.000000000000000000, 0.9510565162951535312, 1.000000000000000000, 0.9510565162951535312, 1.000000000000000000, 0.9510565162951535312, 1.000000000000000000, 0.9510565162951535312, 1.000000000000000000, 0.9510565162951535312, 1.000000000000000000, 0.9510565162951535312, 1.000000000000000000, 0.9510565162951535312, 1.000000000000000000, 0.9510565162951535312, 1.000000000000000000, 0.9510565162951535312, 1.000000000000000000, 0.9510565162951535312, 1.000000000000000000, 0.9510565162951535312, 1.000000000000000000, 0.9510565162951535312, 1.000000000000000000, 0.9510565162951535312, 1.000000000000000000, 0.9510565162951535312, 1.000000000000000000, 0.9510565162951535312, 1.000000000000000000, 0.9510565162951535312, 1.000000000000000000, 0.9510565162951535312, 1.000000000000000000, 0.9510565162951535312, 1.000000000000000000, 0.9510565162951535312, 1.000000000000000000, 0.9510565162951535312, 1.000000000000000000, 0.9510565162951535312, 1.000000000000000000, 0.9510565162951535312, 1.000000000000000000, 0.9510565162951535312, 1.000000000000000000, 0.9510565162951535312, 1.000000000000000000, 0.9510565162951535312, 1.000000000000000000, 0.9510565162951535312, 1.000000000000000000, 0.9510565162951535312, 1.000000000000000000, 0.9510565162951535312, 1.000000000000000000, 0.9510565162951535312, 1.000000000000000000, 0.9510565162951535312, 1.000000000000000000, 0.9510565162951535312, 1.000000000000000000, 0.9510565162951535312, 1.000000000000000000, 0.9510565162951535312, 1.000000000000000000, 0.9510565162951535312, 1.000000000000000000, 0.9510565162951535312, 1.000000000000000000, 0.9510565162951535312, 1.000000000000000000, 0.9510565162951535312, 1.000000000000000000, 0.9510565162951535312, 1.000000000000000000, 0.9510565162951535312, 1.000000000000000000, 0.9510565162951535312, 1.000000000000000000, 0.9510565162951535312, 1.000000000000000000, 0.9510565162951535312, 1.000000000000000000, 0.9510565162951535312, 1.000000000000000000, 0.9510565162951535312, 1.000000000000000000, 0.9510565162951535312, 1.000000000000000000, 0.9510565162951535312, 1.000000000000000000, 0.9510565162951535312, 1.000000000000000000, 0.9510565162951535312, 1.000000000000000000, 0.9510565162951535312, 1.000000000000000000, 0.9510565162951535312, 1.000000000000000000, 0.9510565162951535312, 1.000000000000000000, 0.9510565162951535312, 1.000000000000000000, 0.9510565162951535312, 1.000000000000000000, 0.9510565162951535312, 1.000000000000000000, 0.9510565162951535312, 1.000000000000000000, 0.9510565162951535312, 1.000000000000000000, 0.9510565162951535312, 1.000000000000000000, 0.9510565162951535312, 1.000000000000000000, 0.9510565162951535312, 1.000000000000000000, 0.9510565162951535312, 1.000000000000000000, 0.9510565162951535312, 1.000000000000000000, 0.9510565162951535312, 1.000000000000000000, 0.9510565162951535312, 1.000000000000000000, 0.9510565162951535312, 1.000000000000000000, 0.9510565162951535312, 1.000000000000000000, 0.9510565162951535312, 1.000000000000000000, 0.9510565162951535312, 1.000000000000000000, 0.9510565162951535312, 1.000000000000000000, 0.9510565162951535312, 1.000000000000000000, 0.9510565162951535312, 1.000000000000000000, 0.9510565162951535312, 1.000000000000000000, 0.9510565162951535312, 1.000000000000000000, 0.9510565162951535312, 1.000000000000000000, 0.9510565162951535312, 1.000000000000000000, 0.9510565162951535312, 1.000000000000000000, 0.9510565162951535312, 1.000000000000000000, 0.9510565162951535312, 1.000000000000000000, 0.9510565162951535312, 1.000000000000000000, 0.9510565162951535312, 1.000000000000000000, 0.9510565162951535312, 1.000000000000000000, 0.9510565162951535312, 1.000000000000000000, 0.9510565162951535312, 1.000000000000000000, 0.9510565162951535312, 1.000000000000000000, 0.9510565162951535312, 1.000000000000000000, 0.9510565162951535312, 1.000000000000000000, 0.9510565162951535312, 1.000000000000000000, 0.9510565162951535312, 1.000000000000000000, 0.9510565162951535312, 1.000000000000000000, 0.9510565162951535312, 1.000000000000000000, 0.9510565162951535312, 1.000000000000000000, 0.9510565162951535312, 1.000000000000000000, 0.9510565162951535312, 1.000000000000000000, 0.9510565162951535312, 1.000000000000000000, 0.9510565162951535312, 1.000000000000000000, 0.9510565162951535312, 1.000000000000000000, 0.9510565162951535312, 1.000000000000000000, 0.9510565162951535312, 1.000000000000000000, 0.9510565162951535312, 1.000000000000000000, 0.9510565162951535312, 1.000000000000000000, 0.9510565162951535312, 1.000000000000000000, 0.9510565162951535312, 1.000000000000000000, 0.9510565162951535312, 1.000000000000000000, 0.9510565162951535312, 1.000000000000000000, 0.9510565162951535312, 1.000000000000000000, 0.9510565162951535312, 1.000000000000000000, 0.9510565162951535312, 1.000000000000000000, 0.9510565162951535312, 1.000000000000000000, 0.9510565162951535312, 1.000000000000000000, 0.9510565162951535312, 1.000000000000000000, 0.9510565162951535312, 1.000000000000000000, 0.9510565162951535312, 1.000000000000000000, 0.9510565162951535312, 1.000000000000000000, 0.9510565162951535312, 1.000000000000000000, 0.9510565162951535312, 1.000000000000000000, 0.9510565162951535312, 1.000000000000000000, 0.9510565162951535312, 1.000000000000000000, 0.9510565162951535312, 1.000000000000000000, 0.9510565162951535312, 1.000000000000000000, 0.9510565162951535312, 1.000000000000000000, 0.9510565162951535312, 1.000000000000000000, 0.9510565162951535312, 1.000000000000000000, 0.9510565162951535312, 1.000000000000000000, 0.9510565162951535312, 1.000000000000000000, 0.9510565162951535312, 1.000000000000000000, 0.9510565162951535312, 1.000000000000000000, 0.9510565162951535312, 1.000000000000000000, 0.9510565162951535312, 1.000000000000000000, 0.9510565162951535312, 1.000000000000000000, 0.9510565162951535312, 1.000000000000000000, 0.9510565162951535312, 1.000000000000000000, 0.9510565162951535312, 1.000000000000000000, 0.9510565162951535312, 1.000000000000000000, 0.9510565162951535312, 1.000000000000000000, 0.9510565162951535312, 1.000000000000000000, 0.9510565162951535312, 1.000000000000000000, 0.9510565162951535312, 1.000000000000000000, 0.9510565162951535312, 1.000000000000000000, 0.9510565162951535312, 1.000000000000000000, 0.9510565162951535312, 1.000000000000000000, 0.9510565162951535312, 1.000000000000000000, 0.9510565162951535312, 1.000000000000000000, 0.9510565162951535312, 1.000000000000000000, 0.9510565162951535312, 1.000000000000000000, 0.9510565162951535312, 1.000000000000000000, 0.9510565162951535312, 1.000000000000000000, 0.9510565162951535312, 1.000000000000000000, 0.9510565162951535312, 1.000000000000000000, 0.9510565162951535312, 1.000000000000000000),
 ( 1.000000000000000000, 0.9510565162951535312, 1.000000000000000000, 0.9510565162951535312, 1.000000000000000000, 0.9510565162951535312, 1.000000000000000000, 0.9510565162951535312, 1.000000000000000000, 0.9510565162951535312, 1.000000000000000000, 0.9510565162951535312, 1.000000000000000000, 0.9510565162951535312, 1.000000000000000000, 0.9510565162951535312, 1.000000000000000000, 0.9510565162951535312, 1.000000000000000000, 0.9510565162951535312, 1.000000000000000000, 0.9510565162951535312, 1.000000000000000000, 0.9510565162951535312, 1.000000000000000000, 0.9510565162951535312, 1.000000000000000000, 0.9510565162951535312, 1.000000000000000000, 0.9510565162951535312, 1.000000000000000000, 0.9510565162951535312, 1.000000000000000000, 0.9510565162951535312, 1.000000000000000000, 0.9510565162951535312, 1.000000000000000000, 0.9510565162951535312, 1.000000000000000000, 0.9510565162951535312, 1.000000000000000000, 0.9510565162951535312, 1.000000000000000000, 0.9510565162951535312, 1.000000000000000000, 0.9510565162951535312, 1.000000000000000000, 0.9510565162951535312, 1.000000000000000000, 0.9510565162951535312, 1.000000000000000000, 0.9510565162951535312, 1.000000000000000000, 0.9510565162951535312, 1.000000000000000000, 0.9510565162951535312, 1.000000000000000000, 0.9510565162951535312, 1.000000000000000000, 0.9510565162951535312, 1.000000000000000000, 0.9510565162951535312, 1.000000000000000000, 0.9510565162951535312, 1.000000000000000000, 0.9510565162951535312, 1.000000000000000000, 0.9510565162951535312, 1.000000000000000000, 0.9510565162951535312, 1.000000000000000000, 0.9510565162951535312, 1.000000000000000000, 0.9510565162951535312, 1.000000000000000000, 0.9510565162951535312, 1.000000000000000000, 0.9510565162951535312, 1.000000000000000000, 0.9510565162951535312, 1.000000000000000000, 0.9510565162951535312, 1.000000000000000000, 0.9510565162951535312, 1.000000000000000000, 0.9510565162951535312, 1.000000000000000000, 0.9510565162951535312, 1.000000000000000000, 0.9510565162951535312, 1.000000000000000000, 0.9510565162951535312, 1.000000000000000000, 0.9510565162951535312, 1.000000000000000000, 0.9510565162951535312, 1.000000000000000000, 0.9510565162951535312, 1.000000000000000000, 0.9510565162951535312, 1.000000000000000000, 0.9510565162951535312, 1.000000000000000000, 0.9510565162951535312, 1.000000000000000000, 0.9510565162951535312, 1.000000000000000000, 0.9510565162951535312, 1.000000000000000000, 0.9510565162951535312, 1.000000000000000000, 0.9510565162951535312, 1.000000000000000000, 0.9510565162951535312, 1.000000000000000000, 0.9510565162951535312, 1.000000000000000000, 0.9510565162951535312, 1.000000000000000000, 0.9510565162951535312, 1.000000000000000000, 0.9510565162951535312, 1.000000000000000000, 0.9510565162951535312, 1.000000000000000000, 0.9510565162951535312, 1.000000000000000000, 0.9510565162951535312, 1.000000000000000000, 0.9510565162951535312, 1.000000000000000000, 0.9510565162951535312, 1.000000000000000000, 0.9510565162951535312, 1.000000000000000000, 0.9510565162951535312, 1.000000000000000000, 0.9510565162951535312, 1.000000000000000000, 0.9510565162951535312, 1.000000000000000000, 0.9510565162951535312, 1.000000000000000000, 0.9510565162951535312, 1.000000000000000000, 0.9510565162951535312, 1.000000000000000000, 0.9510565162951535312, 1.000000000000000000, 0.9510565162951535312, 1.000000000000000000, 0.9510565162951535312, 1.000000000000000000, 0.9510565162951535312, 1.000000000000000000, 0.9510565162951535312, 1.000000000000000000, 0.9510565162951535312, 1.000000000000000000, 0.9510565162951535312, 1.000000000000000000, 0.9510565162951535312, 1.000000000000000000, 0.9510565162951535312, 1.000000000000000000, 0.9510565162951535312, 1.000000000000000000, 0.9510565162951535312, 1.000000000000000000, 0.9510565162951535312, 1.000000000000000000, 0.9510565162951535312, 1.000000000000000000, 0.9510565162951535312, 1.000000000000000000, 0.9510565162951535312, 1.000000000000000000, 0.9510565162951535312, 1.000000000000000000, 0.9510565162951535312, 1.000000000000000000, 0.9510565162951535312, 1.000000000000000000, 0.9510565162951535312, 1.000000000000000000, 0.9510565162951535312, 1.000000000000000000, 0.9510565162951535312, 1.000000000000000000, 0.9510565162951535312, 1.000000000000000000, 0.9510565162951535312, 1.000000000000000000, 0.9510565162951535312, 1.000000000000000000, 0.9510565162951535312, 1.000000000000000000, 0.9510565162951535312, 1.000000000000000000, 0.9510565162951535312, 1.000000000000000000, 0.9510565162951535312, 1.000000000000000000, 0.9510565162951535312, 1.000000000000000000, 0.9510565162951535312, 1.000000000000000000, 0.9510565162951535312, 1.000000000000000000, 0.9510565162951535312, 1.000000000000000000, 0.9510565162951535312, 1.000000000000000000, 0.9510565162951535312, 1.000000000000000000, 0.9510565162951535312, 1.000000000000000000, 0.9510565162951535312, 1.000000000000000000, 0.9510565162951535312, 1.000000000000000000, 0.9510565162951535312, 1.000000000000000000, 0.9510565162951535312, 1.000000000000000000, 0.9510565162951535312, 1.000000000000000000, 0.9510565162951535312, 1.000000000000000000, 0.9510565162951535312, 1.000000000000000000, 0.9510565162951535312, 1.000000000000000000, 0.9510565162951535312, 1.000000000000000000, 0.9510565162951535312, 1.000000000000000000, 0.9510565162951535312, 1.000000000000000000, 0.9510565162951535312, 1.000000000000000000, 0.9510565162951535312, 1.000000000000000000, 0.9510565162951535312, 1.000000000000000000, 0.9510565162951535312, 1.000000000000000000, 0.9510565162951535312, 1.000000000000000000, 0.9510565162951535312, 1.000000000000000000, 0.9510565162951535312, 1.000000000000000000, 0.9510565162951535312, 1.000000000000000000, 0.9510565162951535312, 1.000000000000000000, 0.9510565162951535312, 1.000000000000000000, 0.9510565162951535312, 1.000000000000000000, 0.9510565162951535312, 1.000000000000000000, 0.9510565162951535312, 1.000000000000000000, 0.9510565162951535312, 1.000000000000000000, 0.9510565162951535312, 1.000000000000000000, 0.9510565162951535312, 1.000000000000000000, 0.9510565162951535312, 1.000000000000000000, 0.9510565162951535312, 1.000000000000000000, 0.9510565162951535312, 1.000000000000000000, 0.9510565162951535312, 1.000000000000000000, 0.9510565162951535312, 1.000000000000000000, 0.9510565162951535312, 1.000000000000000000, 0.9510565162951535312, 1.000000000000000000, 0.9510565162951535312, 1.000000000000000000, 0.9510565162951535312, 1.000000000000000000, 0.9510565162951535312, 1.000000000000000000, 0.9510565162951535312, 1.000000000000000000, 0.9510565162951535312, 1.000000000000000000, 0.9510565162951535312, 1.000000000000000000, 0.9510565162951535312, 1.000000000000000000, 0.9510565162951535312, 1.000000000000000000, 0.9510565162951535312, 1.000000000000000000, 0.9510565162951535312, 1.000000000000000000, 0.9510565162951535312, 1.000000000000000000, 0.9510565162951535312, 1.000000000000000000, 0.9510565162951535312, 1.000000000000000000, 0.9510565162951535312, 1.000000000000000000, 0.9510565162951535312, 1.000000000000000000, 0.9510565162951535312, 1.000000000000000000, 0.9510565162951535312, 1.000000000000000000, 0.9510565162951535312, 1.000000000000000000, 0.9510565162951535312, 1.000000000000000000, 0.9510565162951535312, 1.000000000000000000, 0.9510565162951535312, 1.000000000000000000, 0.9510565162951535312, 1.000000000000000000, 0.9510565162951535312, 1.000000000000000000, 0.9510565162951535312, 1.000000000000000000, 0.9510565162951535312, 1.000000000000000000, 0.9510565162951535312, 1.000000000000000000, 0.9510565162951535312, 1.000000000000000000, 0.9510565162951535312, 1.000000000000000000, 0.9510565162951535312, 1.000000000000000000, 0.9510565162951535312, 1.000000000000000000, 0.9510565162951535312, 1.000000000000000000, 0.9510565162951535312, 1.000000000000000000, 0.9510565162951535312, 1.000000000000000000, 0.9510565162951535312, 1.000000000000000000, 0.9510565162951535312, 1.000000000000000000, 0.9510565162951535312, 1.000000000000000000, 0.9510565162951535312, 1.000000000000000000, 0.9510565162951535312, 1.000000000000000000, 0.9510565162951535312, 1.000000000000000000, 0.9510565162951535312, 1.000000000000000000, 0.9510565162951535312, 1.000000000000000000, 0.9510565162951535312, 1.000000000000000000, 0.9510565162951535312, 1.000000000000000000, 0.9510565162951535312, 1.000000000000000000, 0.9510565162951535312, 1.000000000000000000, 0.9510565162951535312, 1.000000000000000000, 0.9510565162951535312, 1.000000000000000000, 0.9510565162951535312, 1.000000000000000000, 0.9510565162951535312, 1.000000000000000000, 0.9510565162951535312, 1.000000000000000000, 0.9510565162951535312, 1.000000000000000000, 0.9510565162951535312, 1.000000000000000000, 0.9510565162951535312, 1.000000000000000000, 0.9510565162951535312, 1.000000000000000000, 0.9510565162951535312, 1.000000000000000000, 0.9510565162951535312, 1.000000000000000000, 0.9510565162951535312, 1.000000000000000000, 0.9510565162951535312, 1.000000000000000000, 0.9510565162951535312, 1.000000000000000000, 0.9510565162951535312, 1.000000000000000000, 0.9510565162951535312, 1.000000000000000000, 0.9510565162951535312, 1.000000000000000000, 0.9510565162951535312, 1.000000000000000000, 0.9510565162951535312, 1.000000000000000000, 0.9510565162951535312, 1.000000000000000000, 0.9510565162951535312, 1.000000000000000000, 0.9510565162951535312, 1.000000000000000000, 0.9510565162951535312, 1.000000000000000000, 0.9510565162951535312, 1.000000000000000000, 0.9510565162951535312, 1.000000000000000000, 0.9510565162951535312, 1.000000000000000000, 0.9510565162951535312, 1.000000000000000000, 0.9510565162951535312, 1.000000000000000000, 0.9510565162951535312, 1.000000000000000000, 0.9510565162951535312, 1.000000000000000000, 0.9510565162951535312, 1.000000000000000000, 0.9510565162951535312, 1.000000000000000000, 0.9510565162951535312, 1.000000000000000000, 0.9510565162951535312, 1.000000000000000000, 0.9510565162951535312, 1.000000000000000000, 0.9510565162951535312, 1.000000000000000000, 0.9510565162951535312, 1.000000000000000000, 0.9510565162951535312, 1.000000000000000000, 0.9510565162951535312, 1.000000000000000000, 0.9510565162951535312, 1.000000000000000000, 0.9510565162951535312, 1.000000000000000000, 0.9510565162951535312, 1.000000000000000000, 0.9510565162951535312, 1.000000000000000000, 0.9510565162951535312, 1.000000000000000000, 0.9510565162951535312, 1.000000000000000000, 0.9510565162951535312, 1.000000000000000000, 0.9510565162951535312, 1.000000000000000000, 0.9510565162951535312, 1.000000000000000000, 0.9510565162951535312, 1.000000000000000000, 0.9510565162951535312, 1.000000000000000000, 0.9510565162951535312, 1.000000000000000000, 0.9510565162951535312, 1.000000000000000000, 0.9510565162951535312, 1.000000000000000000, 0.9510565162951535312, 1.000000000000000000, 0.9510565162951535312, 1.000000000000000000, 0.9510565162951535312, 1.000000000000000000, 0.9510565162951535312, 1.000000000000000000, 0.9510565162951535312, 1.000000000000000000, 0.9510565162951535312, 1.000000000000000000, 0.9510565162951535312, 1.000000000000000000, 0.9510565162951535312, 1.000000000000000000, 0.9510565162951535312, 1.000000000000000000, 0.9510565162951535312, 1.000000000000000000, 0.9510565162951535312, 1.000000000000000000, 0.9510565162951535312, 1.000000000000000000, 0.9510565162951535312, 1.000000000000000000, 0.9510565162951535312, 1.000000000000000000, 0.9510565162951535312, 1.000000000000000000, 0.9510565162951535312, 1.000000000000000000, 0.9510565162951535312, 1.000000000000000000, 0.9510565162951535312, 1.000000000000000000, 0.9510565162951535312, 1.000000000000000000, 0.9510565162951535312, 1.000000000000000000, 0.9510565162951535312, 1.000000000000000000, 0.9510565162951535312, 1.000000000000000000, 0.9510565162951535312, 1.000000000000000000, 0.9510565162951535312, 1.000000000000000000, 0.9510565162951535312, 1.000000000000000000, 0.9510565162951535312, 1.000000000000000000, 0.9510565162951535312, 1.000000000000000000, 0.9510565162951535312, 1.000000000000000000, 0.9510565162951535312, 1.000000000000000000, 0.9510565162951535312, 1.000000000000000000, 0.9510565162951535312, 1.000000000000000000, 0.9510565162951535312, 1.000000000000000000, 0.9510565162951535312, 1.000000000000000000, 0.9510565162951535312, 1.000000000000000000, 0.9510565162951535312, 1.000000000000000000) ) ) 
 REPRESENTATION_ITEM ( '' )  SURFACE ( )  );
#23281=VECTOR ( 'NONE', #29786, 1000.000000000000000 ) ;
#23284=AXIS2_PLACEMENT_3D ( 'NONE', #9207, #19597, #7155 ) ;
#23289=CARTESIAN_POINT ( 'NONE',  ( 78.57499999726881867, 145.8408176439707802, 12.60653300113718345 ) ) ;
#23291=EDGE_LOOP ( 'NONE', ( #18632, #5191, #24761, #15667 ) ) ;
#23293=CARTESIAN_POINT ( 'NONE',  ( 73.22499999726881015, 160.0630714827496206, -15.58253175000000823 ) ) ;
#23297=CARTESIAN_POINT ( 'NONE',  ( 62.02499999726880020, 160.0630714827496206, 15.58253174999999402 ) ) ;
#23306=CARTESIAN_POINT ( 'NONE',  ( 127.5000000000000000, 155.0000000000000000, -6.938893903907228378E-15 ) ) ;
#23312=CARTESIAN_POINT ( 'NONE',  ( 125.5000000000000000, 229.9533188057749555, 74.95331880577313655 ) ) ;
#23314=CARTESIAN_POINT ( 'NONE',  ( 39.72499999726881015, 169.8198683612136222, 4.815267126137181997 ) ) ;
#23320=CARTESIAN_POINT ( 'NONE',  ( 75.78867513459483973, 155.0000000000000000, 15.00000000000001243 ) ) ;
#23323=CARTESIAN_POINT ( 'NONE',  ( 70.69999999453764872, 167.3344367211045096, 8.961492836873468093 ) ) ;
#23330=ORIENTED_EDGE ( 'NONE', *, *, #28229, .T. ) ;
#23332=EDGE_LOOP ( 'NONE', ( #23496, #10310, #30320, #786 ) ) ;
#23334=VERTEX_POINT ( 'NONE', #20765 ) ;
#23338=AXIS2_PLACEMENT_3D ( 'NONE', #9041, #16539, #32378 ) ;
#23339=FACE_OUTER_BOUND ( 'NONE', #6120, .T. ) ;
#23345=CARTESIAN_POINT ( 'NONE',  ( 61.17499999726882010, 145.8408176439707802, -12.60653300113719588 ) ) ;
#23353=CARTESIAN_POINT ( 'NONE',  ( 79.71132485994280614, 155.0000000000000000, -15.00000000000002487 ) ) ;
#23358=CARTESIAN_POINT ( 'NONE',  ( 84.10000000000000853, 141.2096805137202580, -4.480746418436742040 ) ) ;
#23363=CARTESIAN_POINT ( 'NONE',  ( 57.27499999726882152, 149.9369285172503510, -15.58253175000000823 ) ) ;
#23370=CARTESIAN_POINT ( 'NONE',  ( 56.79999999453762882, 163.5228861582408797, 11.73074641843673049 ) ) ;
#23379=VERTEX_POINT ( 'NONE', #23160 ) ;
#23386=CARTESIAN_POINT ( 'NONE',  ( 42.07499999726881157, 168.2552932293087906, 9.630534252274372875 ) ) ;
#23388=CARTESIAN_POINT ( 'NONE',  ( 51.92499999726880588, 164.1591823560292198, 12.60653300113718167 ) ) ;
#23392=CARTESIAN_POINT ( 'NONE',  ( 56.47499999726881015, 149.9369285172503510, 15.58253174999999580 ) ) ;
#23396=CARTESIAN_POINT ( 'NONE',  ( 65.90000000000000568, 141.2096805137202580, 4.480746418436733158 ) ) ;
#23397=( BOUNDED_CURVE ( )  B_SPLINE_CURVE ( 2, ( #28190, #15238, #30749, #24958, #6730, #2133, #12516, #25289, #19841, #22905, #12004 ),
 .UNSPECIFIED., .F., .T. ) 
 B_SPLINE_CURVE_WITH_KNOTS ( ( 3, 2, 2, 2, 2, 3 ),
 ( 0.3749999999999997780, 0.3785714285714283367, 0.3821428571428569509, 0.3857142857142855097, 0.3892857142857141239, 0.3928571428571426827 ),
 .UNSPECIFIED. ) 
 CURVE ( )  GEOMETRIC_REPRESENTATION_ITEM ( )  RATIONAL_B_SPLINE_CURVE ( ( 1.000000000000003109, 0.9510565162951504226, 1.000000000000000000, 0.9510565162951534202, 1.000000000000000000, 0.9510565162951534202, 1.000000000000000000, 0.9510565162951534202, 1.000000000000000000, 0.9510565162951549745, 0.9999999999999984457 ) ) 
 REPRESENTATION_ITEM ( '' )  );
#23402=FACE_OUTER_BOUND ( 'NONE', #8494, .T. ) ;
#23404=CARTESIAN_POINT ( 'NONE',  ( 71.32499999726881867, 164.1591823560292198, -12.60653300113719766 ) ) ;
#23407=CARTESIAN_POINT ( 'NONE',  ( 87.07499999726880446, 141.7447067706911810, -9.630534252274385310 ) ) ;
#23424=ORIENTED_EDGE ( 'NONE', *, *, #16665, .T. ) ;
#23427=CARTESIAN_POINT ( 'NONE',  ( 84.22499999726879594, 149.9369285172503510, 15.58253174999999580 ) ) ;
#23431=CARTESIAN_POINT ( 'NONE',  ( 50.10000000000000853, 141.2096805137202580, -4.480746418436742040 ) ) ;
#23434=CARTESIAN_POINT ( 'NONE',  ( 50.92499999726880588, 145.8408176439707802, -12.60653300113719588 ) ) ;
#23436=CARTESIAN_POINT ( 'NONE',  ( 87.50000000000001421, 155.0000000000000000, -70.00000000000002842 ) ) ;
#23437=CARTESIAN_POINT ( 'NONE',  ( 58.32499999726881157, 145.8408176439707802, 12.60653300113718345 ) ) ;
#23438=CARTESIAN_POINT ( 'NONE',  ( 73.17499999726881299, 145.8408176439707802, -12.60653300113719588 ) ) ;
#23443=CARTESIAN_POINT ( 'NONE',  ( 35.68867513459483121, 159.8737954434934920, 15.00000000000010836 ) ) ;
#23457=EDGE_CURVE ( 'NONE', #25621, #27498, #26318, .T. ) ;
#23458=CARTESIAN_POINT ( 'NONE',  ( 72.62499999726880162, 138.6155565068815747, -3.929120461958505118E-15 ) ) ;
#23462=CARTESIAN_POINT ( 'NONE',  ( 63.62499999726879452, 171.3844434931184253, -7.942151717890132712E-15 ) ) ;
#23477=CARTESIAN_POINT ( 'NONE',  ( 39.82499999726881157, 168.2552932293087906, 9.630534252274372875 ) ) ;
#23479=FACE_OUTER_BOUND ( 'NONE', #8518, .T. ) ;
#23486=CARTESIAN_POINT ( 'NONE',  ( 78.89999999453762314, 159.7113355953771077, 14.49999999999999289 ) ) ;
#23491=CARTESIAN_POINT ( 'NONE',  ( 49.58867513459482268, 163.8167787843871110, 12.13525491562421621 ) ) ;
#23496=ORIENTED_EDGE ( 'NONE', *, *, #28982, .F. ) ;
#23503=CARTESIAN_POINT ( 'NONE',  ( 63.87499999726880873, 171.3844434931184253, -7.942151717890134290E-15 ) ) ;
#23510=CARTESIAN_POINT ( 'NONE',  ( 79.91132485994282320, 163.8167787843871110, -12.13525491562423397 ) ) ;
#23517=CARTESIAN_POINT ( 'NONE',  ( 85.90000000000000568, 141.2096805137202580, 4.480746418436733158 ) ) ;
#23519=FACE_OUTER_BOUND ( 'NONE', #30917, .T. ) ;
#23522=CARTESIAN_POINT ( 'NONE',  ( 56.97499999726881015, 140.1801316387863778, -4.815267126137194431 ) ) ;
#23529=CARTESIAN_POINT ( 'NONE',  ( 63.09999999453763309, 150.2886644046228639, 14.49999999999999645 ) ) ;
#23533=DIRECTION ( 'NONE',  ( 1.000000000000000000, 0.000000000000000000, 0.000000000000000000 ) ) ;
#23536=ORIENTED_EDGE ( 'NONE', *, *, #8975, .T. ) ;
#23546=CARTESIAN_POINT ( 'NONE',  ( 43.17499999726881299, 145.8408176439707802, -12.60653300113719588 ) ) ;
#23548=CARTESIAN_POINT ( 'NONE',  ( 52.72499999726881015, 140.1801316387863778, -4.815267126137194431 ) ) ;
#23552=CARTESIAN_POINT ( 'NONE',  ( 55.97499999726881015, 169.8198683612136222, 4.815267126137181997 ) ) ;
#23555=CARTESIAN_POINT ( 'NONE',  ( 44.28867513459481842, 139.2280666364260071, -4.041636747397287284E-15 ) ) ;
#23556=EDGE_CURVE ( 'NONE', #5223, #31333, #25226, .T. ) ;
#23559=CARTESIAN_POINT ( 'NONE',  ( 67.19999999999998863, 167.3344367211045096, 8.961492836873468093 ) ) ;
#23561=CARTESIAN_POINT ( 'NONE',  ( 37.88867513459482694, 150.1262045565064227, 15.00000000000001599 ) ) ;
#23564=ADVANCED_FACE ( 'NONE', ( #31814 ), #10559, .T. ) ;
#23565=CARTESIAN_POINT ( 'NONE',  ( 35.37499999726881583, 155.0000000000000000, -15.58253175000000823 ) ) ;
#23569=CARTESIAN_POINT ( 'NONE',  ( 70.52499999726880731, 140.1801316387863778, 4.815267126137185549 ) ) ;
#23572=CARTESIAN_POINT ( 'NONE',  ( 38.39999999453763024, 168.7903194862797420, -4.480746418436745593 ) ) ;
#23574=AXIS2_PLACEMENT_3D ( 'NONE', #3122, #27133, #26958 ) ;
#23585=CARTESIAN_POINT ( 'NONE',  ( 74.71132485994280614, 155.0000000000000000, 15.00000000000001243 ) ) ;
#23594=( BOUNDED_CURVE ( )  B_SPLINE_CURVE ( 2, ( #19118, #24057, #29508, #8075, #21504, #6161, #10956, #29009, #16223, #13503, #5502 ),
 .UNSPECIFIED., .F., .T. ) 
 B_SPLINE_CURVE_WITH_KNOTS ( ( 3, 2, 2, 2, 2, 3 ),
 ( 0.2499999999999999445, 0.2535714285714285032, 0.2571428571428570620, 0.2607142857142857317, 0.2642857142857142905, 0.2678571428571428492 ),
 .UNSPECIFIED. ) 
 CURVE ( )  GEOMETRIC_REPRESENTATION_ITEM ( )  RATIONAL_B_SPLINE_CURVE ( ( 1.000000000000000666, 0.9510565162951526430, 1.000000000000000000, 0.9510565162951534202, 1.000000000000000000, 0.9510565162951534202, 1.000000000000000000, 0.9510565162951534202, 1.000000000000000000, 0.9510565162951534202, 1.000000000000000000 ) ) 
 REPRESENTATION_ITEM ( '' )  );
#23595=CARTESIAN_POINT ( 'NONE',  ( 36.27499999726880731, 160.0630714827496206, 15.58253174999999402 ) ) ;
#23600=CARTESIAN_POINT ( 'NONE',  ( 49.39999999999999147, 159.7113355953771077, 14.49999999999999289 ) ) ;
#23603=CARTESIAN_POINT ( 'NONE',  ( 49.22499999726881725, 160.0630714827496206, -15.58253175000000823 ) ) ;
#23606=CARTESIAN_POINT ( 'NONE',  ( 66.52499999726880731, 140.1801316387863778, 4.815267126137185549 ) ) ;
#23607=CARTESIAN_POINT ( 'NONE',  ( 67.07499999726880446, 141.7447067706911810, -9.630534252274385310 ) ) ;
#23617=CIRCLE ( 'NONE', #11650, 2.149999999999974598 ) ;
#23619=EDGE_LOOP ( 'NONE', ( #30244, #26889 ) ) ;
#23621=ORIENTED_EDGE ( 'NONE', *, *, #2242, .T. ) ;
#23622=DIRECTION ( 'NONE',  ( 1.000000000000000000, 0.000000000000000000, 0.000000000000000000 ) ) ;
#23624=ORIENTED_EDGE ( 'NONE', *, *, #29387, .T. ) ;
#23625=CARTESIAN_POINT ( 'NONE',  ( 78.92499999726881299, 145.8408176439707802, -12.60653300113719588 ) ) ;
#23626=DIRECTION ( 'NONE',  ( 1.000000000000000000, 0.000000000000000000, 0.000000000000000000 ) ) ;
#23627=COLOUR_RGB ( '', 0.31764706, 0.68627451, 0.89019608) ;
#23629=CARTESIAN_POINT ( 'NONE',  ( 67.12499999726881583, 155.0000000000000000, -15.58253175000000823 ) ) ;
#23639=FACE_OUTER_BOUND ( 'NONE', #30371, .T. ) ;
#23645=CARTESIAN_POINT ( 'NONE',  ( 43.12499999726881583, 155.0000000000000000, -15.58253175000000823 ) ) ;
#23647=DIRECTION ( 'NONE',  ( 1.000000000000000000, 0.000000000000000000, 0.000000000000000000 ) ) ;
#23653=CARTESIAN_POINT ( 'NONE',  ( 82.39999999453763735, 168.7903194862797420, -4.480746418436745593 ) ) ;
#23667=CARTESIAN_POINT ( 'NONE',  ( 63.17499999726880588, 145.8408176439707802, -12.60653300113719588 ) ) ;
#23678=CARTESIAN_POINT ( 'NONE',  ( 82.47499999726881015, 149.9369285172503510, 15.58253174999999580 ) ) ;
#23680=CARTESIAN_POINT ( 'NONE',  ( 41.62499999726880162, 171.3844434931184253, -7.942151717890132712E-15 ) ) ;
#23685=CARTESIAN_POINT ( 'NONE',  ( 56.77499999726881441, 140.1801316387863778, 4.815267126137185549 ) ) ;
#23692=CARTESIAN_POINT ( 'NONE',  ( 61.29999999453762882, 142.6655632788954620, 8.961492836873471646 ) ) ;
#23697=CARTESIAN_POINT ( 'NONE',  ( 44.91132485994280898, 146.1832212156128890, 12.13525491562421976 ) ) ;
#23709=CARTESIAN_POINT ( 'NONE',  ( 45.77499999726881441, 169.8198683612136222, -4.815267126137197984 ) ) ;
#23711=CARTESIAN_POINT ( 'NONE',  ( 48.92499999726881299, 145.8408176439707802, -12.60653300113719588 ) ) ;
#23716=CARTESIAN_POINT ( 'NONE',  ( 50.97499999726881725, 140.1801316387863778, -4.815267126137194431 ) ) ;
#23719=CARTESIAN_POINT ( 'NONE',  ( 43.98867513459482836, 146.1832212156128890, 12.13525491562421976 ) ) ;
#23720=CARTESIAN_POINT ( 'NONE',  ( 71.60000000000000853, 150.2886644046228639, 14.49999999999999645 ) ) ;
#23724=CARTESIAN_POINT ( 'NONE',  ( 56.98867513459482126, 163.8167787843871110, -12.13525491562423397 ) ) ;
#23725=CARTESIAN_POINT ( 'NONE',  ( 40.37499999726880873, 155.0000000000000000, 15.58253174999999402 ) ) ;
#23727=CARTESIAN_POINT ( 'NONE',  ( 71.62499999726881583, 171.3844434931184253, -7.942151717890132712E-15 ) ) ;
#23729=LINE ( 'NONE', #24227, #33153 ) ;
#23730=CARTESIAN_POINT ( 'NONE',  ( 39.49999999453761745, 139.7537977485451393, -4.138211985947621020E-15 ) ) ;
#23731=( BOUNDED_CURVE ( )  B_SPLINE_CURVE ( 2, ( #46, #23867, #3086, #31542, #364, #10768, #7711, #15701, #20813, #10607, #28323 ),
 .UNSPECIFIED., .F., .T. ) 
 B_SPLINE_CURVE_WITH_KNOTS ( ( 3, 2, 2, 2, 2, 3 ),
 ( 0.1785714285714286031, 0.1821428571428571619, 0.1857142857142857484, 0.1892857142857143071, 0.1928571428571428936, 0.1964285714285714524 ),
 .UNSPECIFIED. ) 
 CURVE ( )  GEOMETRIC_REPRESENTATION_ITEM ( )  RATIONAL_B_SPLINE_CURVE ( ( 0.9999999999999996669, 0.9510565162951537532, 1.000000000000000000, 0.9510565162951534202, 1.000000000000000000, 0.9510565162951534202, 1.000000000000000000, 0.9510565162951534202, 1.000000000000000000, 0.9510565162951530871, 1.000000000000000444 ) ) 
 REPRESENTATION_ITEM ( '' )  );
#23740=ADVANCED_FACE ( 'NONE', ( #32482 ), #14429, .T. ) ;
#23743=CARTESIAN_POINT ( 'NONE',  ( 74.01132485994280330, 167.7597621252805880, -9.270509831248443078 ) ) ;
#23751=CARTESIAN_POINT ( 'NONE',  ( 34.12499999726881583, 155.0000000000000000, 15.58253174999999402 ) ) ;
#23753=CARTESIAN_POINT ( 'NONE',  ( 87.02499999726879309, 149.9369285172503510, -15.58253175000000823 ) ) ;
#23757=CARTESIAN_POINT ( 'NONE',  ( 50.89999999999999858, 168.7903194862797420, -4.480746418436745593 ) ) ;
#23760=CARTESIAN_POINT ( 'NONE',  ( 50.22499999726880304, 149.9369285172503510, 15.58253174999999580 ) ) ;
#23763=VERTEX_POINT ( 'NONE', #27210 ) ;
#23764=DIRECTION ( 'NONE',  ( 0.000000000000000000, 0.000000000000000000, -1.000000000000000000 ) ) ;
#23765=CARTESIAN_POINT ( 'NONE',  ( 64.02499999726880731, 160.0630714827496206, 15.58253174999999224 ) ) ;
#23766=CARTESIAN_POINT ( 'NONE',  ( 75.37499999726881583, 155.0000000000000000, -15.58253175000000823 ) ) ;
#23770=CARTESIAN_POINT ( 'NONE',  ( 53.78867513459483263, 155.0000000000000000, 15.00000000000001243 ) ) ;
#23776=CARTESIAN_POINT ( 'NONE',  ( 34.18867513459482410, 140.7341522555726669, 4.635254915624211769 ) ) ;
#23787=CARTESIAN_POINT ( 'NONE',  ( 75.32499999726881867, 164.1591823560292198, -12.60653300113719766 ) ) ;
#23788=CARTESIAN_POINT ( 'NONE',  ( 125.5000000000000000, 80.04668119422552763, -74.95331880577366235 ) ) ;
#23791=CARTESIAN_POINT ( 'NONE',  ( 68.12499999726881583, 155.0000000000000000, 15.58253174999999402 ) ) ;
#23793=CIRCLE ( 'NONE', #2042, 2.149999999999985256 ) ;
#23795=CARTESIAN_POINT ( 'NONE',  ( 125.5000000000000000, 152.8500000000011028, 106.0000000000000426 ) ) ;
#23798=CARTESIAN_POINT ( 'NONE',  ( 48.71132485994280614, 155.0000000000000000, 15.00000000000001243 ) ) ;
#23804=CARTESIAN_POINT ( 'NONE',  ( 41.82499999726881157, 168.2552932293087906, 9.630534252274372875 ) ) ;
#23812=CARTESIAN_POINT ( 'NONE',  ( 82.79999999453762882, 163.5228861582408797, 11.73074641843673049 ) ) ;
#23817=CARTESIAN_POINT ( 'NONE',  ( 49.08867513459482979, 167.7597621252805880, -9.270509831248443078 ) ) ;
#23821=ORIENTED_EDGE ( 'NONE', *, *, #18949, .F. ) ;
#23822=EDGE_LOOP ( 'NONE', ( #2995, #26284 ) ) ;
#23823=CARTESIAN_POINT ( 'NONE',  ( 75.77499999726880731, 169.8198683612136222, -4.815267126137197984 ) ) ;
#23824=CARTESIAN_POINT ( 'NONE',  ( 52.71132485994279904, 155.0000000000000000, 15.00000000000001243 ) ) ;
#23831=CARTESIAN_POINT ( 'NONE',  ( 60.57499999726881157, 145.8408176439707802, 12.60653300113718345 ) ) ;
#23833=CARTESIAN_POINT ( 'NONE',  ( 62.58867513459481557, 146.1832212156128890, -12.13525491562423042 ) ) ;
#23837=CARTESIAN_POINT ( 'NONE',  ( 83.48867513459482836, 167.7597621252805880, 9.270509831248428867 ) ) ;
#23839=CARTESIAN_POINT ( 'NONE',  ( 82.37499999726881583, 155.0000000000000000, 15.58253174999999402 ) ) ;
#23843=CARTESIAN_POINT ( 'NONE',  ( 39.02499999726880731, 149.9369285172503510, -15.58253175000000823 ) ) ;
#23847=CARTESIAN_POINT ( 'NONE',  ( 55.47499999726881015, 160.0630714827496206, -15.58253175000000823 ) ) ;
#23853=CARTESIAN_POINT ( 'NONE',  ( 59.99999999453763166, 155.0000000000000000, -14.50000000000000711 ) ) ;
#23856=AXIS2_PLACEMENT_3D ( 'NONE', #9818, #4023, #4696 ) ;
#23860=CARTESIAN_POINT ( 'NONE',  ( 72.51132485994280330, 163.8167787843871110, 12.13525491562421621 ) ) ;
#23867=CARTESIAN_POINT ( 'NONE',  ( 43.81132485994280046, 159.8737954434936341, -15.00000000000000355 ) ) ;
#23873=CARTESIAN_POINT ( 'NONE',  ( 44.47499999726880304, 149.9369285172503510, 15.58253174999999580 ) ) ;
#23875=CARTESIAN_POINT ( 'NONE',  ( 48.52499999726880731, 140.1801316387863778, 4.815267126137185549 ) ) ;
#23878=ADVANCED_FACE ( 'NONE', ( #10012, #9656 ), #25326, .T. ) ;
#23880=CARTESIAN_POINT ( 'NONE',  ( 56.07499999726881157, 168.2552932293087906, 9.630534252274372875 ) ) ;
#23886=CARTESIAN_POINT ( 'NONE',  ( 76.89999999999999147, 168.7903194862797420, -4.480746418436745593 ) ) ;
#23890=CARTESIAN_POINT ( 'NONE',  ( 57.68867513459482410, 159.8737954434937478, 14.99999999999991651 ) ) ;
#23891=CARTESIAN_POINT ( 'NONE',  ( 41.17499999726881299, 145.8408176439707802, -12.60653300113719588 ) ) ;
#23894=CARTESIAN_POINT ( 'NONE',  ( 77.02499999726880731, 149.9369285172503510, -15.58253175000000823 ) ) ;
#23897=CARTESIAN_POINT ( 'NONE',  ( 40.79999999453762882, 163.5228861582408797, 11.73074641843673049 ) ) ;
#23917=CARTESIAN_POINT ( 'NONE',  ( 34.62499999726880873, 138.6155565068815463, -3.929120461958505118E-15 ) ) ;
#23918=CARTESIAN_POINT ( 'NONE',  ( 86.62499999726883004, 138.6155565068815463, -3.929120461958505118E-15 ) ) ;
#23922=CARTESIAN_POINT ( 'NONE',  ( 54.00000000000000000, 139.7537977485451393, -4.138211985947621020E-15 ) ) ;
#23926=( BOUNDED_CURVE ( )  B_SPLINE_CURVE ( 2, ( #21174, #565, #21678, #8730, #19121, #16559, #5672, #5999, #8565, #8894, #893 ),
 .UNSPECIFIED., .F., .T. ) 
 B_SPLINE_CURVE_WITH_KNOTS ( ( 3, 2, 2, 2, 2, 3 ),
 ( 0.1071428571428571092, 0.1107142857142856818, 0.1142857142857142544, 0.1178571428571428270, 0.1214285714285713996, 0.1249999999999999722 ),
 .UNSPECIFIED. ) 
 CURVE ( )  GEOMETRIC_REPRESENTATION_ITEM ( )  RATIONAL_B_SPLINE_CURVE ( ( 1.000000000000000444, 0.9510565162951530871, 1.000000000000000000, 0.9510565162951534202, 1.000000000000000000, 0.9510565162951534202, 1.000000000000000000, 0.9510565162951534202, 1.000000000000000000, 0.9510565162951537532, 0.9999999999999996669 ) ) 
 REPRESENTATION_ITEM ( '' )  );
#23928=CARTESIAN_POINT ( 'NONE',  ( 60.12499999726880873, 155.0000000000000000, 15.58253174999999402 ) ) ;
#23932=CARTESIAN_POINT ( 'NONE',  ( 62.32499999726881867, 145.8408176439707802, 12.60653300113718345 ) ) ;
#23933=CARTESIAN_POINT ( 'NONE',  ( 78.97499999726881015, 140.1801316387863778, -4.815267126137194431 ) ) ;
#23935=CYLINDRICAL_SURFACE ( 'NONE', #27684, 15.00000000000001776 ) ;
#23938=CARTESIAN_POINT ( 'NONE',  ( 53.68867513459483121, 159.8737954434933499, 15.00000000000019895 ) ) ;
#23953=CARTESIAN_POINT ( 'NONE',  ( 77.42499999726881299, 168.2552932293087906, -9.630534252274387086 ) ) ;
#23958=CARTESIAN_POINT ( 'NONE',  ( 70.62499999726881583, 138.6155565068815463, -3.929120461958505118E-15 ) ) ;
#23963=CARTESIAN_POINT ( 'NONE',  ( 33.20000000000000284, 167.3344367211045096, 8.961492836873468093 ) ) ;
#23972=CARTESIAN_POINT ( 'NONE',  ( 44.92499999726880588, 145.8408176439707802, -12.60653300113719588 ) ) ;
#23981=CARTESIAN_POINT ( 'NONE',  ( 78.59999999453762598, 168.7903194862797420, 4.480746418436729606 ) ) ;
#23991=CARTESIAN_POINT ( 'NONE',  ( 75.57499999726881867, 164.1591823560292198, -12.60653300113719766 ) ) ;
#23992=CARTESIAN_POINT ( 'NONE',  ( 53.01132485994281751, 142.2402378747194405, 9.270509831248432420 ) ) ;
#23998=CARTESIAN_POINT ( 'NONE',  ( 67.87499999726881583, 171.3844434931184253, -7.942151717890134290E-15 ) ) ;
#24000=CARTESIAN_POINT ( 'NONE',  ( 67.98867513459482836, 146.1832212156128890, 12.13525491562421976 ) ) ;
#24004=CARTESIAN_POINT ( 'NONE',  ( 80.21132485994280614, 170.7719333635740497, -7.904646289410545231E-15 ) ) ;
#24006=CARTESIAN_POINT ( 'NONE',  ( 85.77499999726880731, 169.8198683612136222, -4.815267126137197984 ) ) ;
#24010=CARTESIAN_POINT ( 'NONE',  ( 40.72499999726881725, 140.1801316387863778, -4.815267126137194431 ) ) ;
#24015=CARTESIAN_POINT ( 'NONE',  ( 56.17499999726881299, 164.1591823560292198, 12.60653300113718167 ) ) ;
#24022=CARTESIAN_POINT ( 'NONE',  ( 61.59999999453763309, 141.2096805137202580, -4.480746418436742040 ) ) ;
#24023=EDGE_LOOP ( 'NONE', ( #18968, #6092, #30910, #11064 ) ) ;
#24029=EDGE_LOOP ( 'NONE', ( #18181, #18346, #22869, #2171 ) ) ;
#24030=CARTESIAN_POINT ( 'NONE',  ( 50.61132485994281893, 159.8737954434936057, 15.00000000000001421 ) ) ;
#24036=CARTESIAN_POINT ( 'NONE',  ( 41.57499999726881157, 164.1591823560292198, -12.60653300113719766 ) ) ;
#24038=CARTESIAN_POINT ( 'NONE',  ( 50.52499999726880731, 140.1801316387863778, 4.815267126137185549 ) ) ;
#24043=CARTESIAN_POINT ( 'NONE',  ( 51.87499999726880162, 171.3844434931184253, -7.942151717890132712E-15 ) ) ;
#24047=CARTESIAN_POINT ( 'NONE',  ( 76.00000000000002842, 139.7537977485451393, -4.138211985947621020E-15 ) ) ;
#24051=CARTESIAN_POINT ( 'NONE',  ( 33.78867513459482552, 155.0000000000000000, 15.00000000000001243 ) ) ;
#24052=CARTESIAN_POINT ( 'NONE',  ( 35.57499999726881157, 164.1591823560292198, -12.60653300113719766 ) ) ;
#24054=CARTESIAN_POINT ( 'NONE',  ( 78.42499999726882720, 141.7447067706911810, 9.630534252274376428 ) ) ;
#24057=CARTESIAN_POINT ( 'NONE',  ( 47.81132485994282177, 159.8737954434935489, -15.00000000000007638 ) ) ;
#24058=CARTESIAN_POINT ( 'NONE',  ( 41.19999999453762740, 146.4771138417591203, 11.73074641843673227 ) ) ;
#24070=AXIS2_PLACEMENT_3D ( 'NONE', #8691, #19083, #29472 ) ;
#24073=CARTESIAN_POINT ( 'NONE',  ( 79.18867513459481700, 169.2658477444273331, -4.635254915624224203 ) ) ;
#24074=ORIENTED_EDGE ( 'NONE', *, *, #16386, .F. ) ;
#24077=CARTESIAN_POINT ( 'NONE',  ( 56.51132485994280330, 163.8167787843871110, 12.13525491562421621 ) ) ;
#24081=CARTESIAN_POINT ( 'NONE',  ( 36.77499999726881441, 140.1801316387863778, 4.815267126137185549 ) ) ;
#24086=CARTESIAN_POINT ( 'NONE',  ( 52.29999999999999716, 146.4771138417591203, -11.73074641843674470 ) ) ;
#24091=CARTESIAN_POINT ( 'NONE',  ( 59.02499999726880731, 149.9369285172503510, -15.58253175000000823 ) ) ;
#24093=CARTESIAN_POINT ( 'NONE',  ( 37.11132485994280472, 140.7341522555726669, 4.635254915624211769 ) ) ;
#24094=CARTESIAN_POINT ( 'NONE',  ( 65.62499999726880162, 171.3844434931184253, -7.942151717890134290E-15 ) ) ;
#24095=CARTESIAN_POINT ( 'NONE',  ( 77.57499999726881867, 164.1591823560292198, -12.60653300113719766 ) ) ;
#24110=ADVANCED_FACE ( 'NONE', ( #26014 ), #121, .T. ) ;
#24112=AXIS2_PLACEMENT_3D ( 'NONE', #13489, #7896, #10294 ) ;
#24118=CARTESIAN_POINT ( 'NONE',  ( 75.82499999726881867, 168.2552932293087906, 9.630534252274372875 ) ) ;
#24120=FACE_OUTER_BOUND ( 'NONE', #23117, .T. ) ;
#24121=CARTESIAN_POINT ( 'NONE',  ( 70.52499999726880731, 140.1801316387863778, 4.815267126137185549 ) ) ;
#24122=EDGE_CURVE ( 'NONE', #22913, #23167, #17809, .T. ) ;
#24127=CARTESIAN_POINT ( 'NONE',  ( 33.50000000000000000, 155.0000000000000000, 14.49999999999999467 ) ) ;
#24137=CARTESIAN_POINT ( 'NONE',  ( 44.62499999726880873, 138.6155565068815747, -3.929120461958505118E-15 ) ) ;
#24145=CARTESIAN_POINT ( 'NONE',  ( 86.19999999453763451, 163.5228861582408797, -11.73074641843674470 ) ) ;
#24149=CARTESIAN_POINT ( 'NONE',  ( 48.88867513459482694, 159.8737954434937478, -14.99999999999993072 ) ) ;
#24150=ORIENTED_EDGE ( 'NONE', *, *, #29938, .F. ) ;
#24158=CARTESIAN_POINT ( 'NONE',  ( 77.07499999726881867, 141.7447067706911810, -9.630534252274387086 ) ) ;
#24167=CARTESIAN_POINT ( 'NONE',  ( 68.57499999726881867, 145.8408176439707802, 12.60653300113718345 ) ) ;
#24169=CARTESIAN_POINT ( 'NONE',  ( 62.48867513459482836, 142.2402378747194405, -9.270509831248439525 ) ) ;
#24170=CARTESIAN_POINT ( 'NONE',  ( 43.08867513459483689, 167.7597621252805880, -9.270509831248443078 ) ) ;
#24176=CARTESIAN_POINT ( 'NONE',  ( 84.07499999726877604, 168.2552932293087906, 9.630534252274372875 ) ) ;
#24180=CARTESIAN_POINT ( 'NONE',  ( 39.22499999726881015, 160.0630714827496206, -15.58253175000000823 ) ) ;
#24183=CARTESIAN_POINT ( 'NONE',  ( 117.5000000000000142, 155.0000000000000000, -98.00000000000002842 ) ) ;
#24184=CARTESIAN_POINT ( 'NONE',  ( 64.47499999726881015, 149.9369285172503510, 15.58253174999999580 ) ) ;
#24191=CARTESIAN_POINT ( 'NONE',  ( 61.89999999453763024, 150.2886644046228639, -14.50000000000000888 ) ) ;
#24196=CARTESIAN_POINT ( 'NONE',  ( 58.71132485994280614, 155.0000000000000000, 15.00000000000001243 ) ) ;
#24199=ORIENTED_EDGE ( 'NONE', *, *, #31340, .T. ) ;
#24202=CARTESIAN_POINT ( 'NONE',  ( 57.71132485994280614, 155.0000000000000000, -15.00000000000002487 ) ) ;
#24207=CARTESIAN_POINT ( 'NONE',  ( 49.27499999726880020, 149.9369285172503510, -15.58253175000000823 ) ) ;
#24209=CARTESIAN_POINT ( 'NONE',  ( 58.62499999726880162, 138.6155565068815463, -3.929120461958505118E-15 ) ) ;
#24214=CARTESIAN_POINT ( 'NONE',  ( 58.47499999726880304, 149.9369285172503510, 15.58253174999999580 ) ) ;
#24218=CARTESIAN_POINT ( 'NONE',  ( 74.00000000000000000, 139.7537977485451393, -4.138211985947621020E-15 ) ) ;
#24219=CARTESIAN_POINT ( 'NONE',  ( 64.78867513459482552, 155.0000000000000000, -15.00000000000002487 ) ) ;
#24222=DIRECTION ( 'NONE',  ( -1.000000000000000000, 0.000000000000000000, -0.000000000000000000 ) ) ;
#24223=CARTESIAN_POINT ( 'NONE',  ( 40.27499999726881441, 160.0630714827496206, 15.58253174999999402 ) ) ;
#24225=CARTESIAN_POINT ( 'NONE',  ( 74.62499999726883004, 138.6155565068815463, -3.929120461958505118E-15 ) ) ;
#24227=CARTESIAN_POINT ( 'NONE',  ( 32.50000000000000000, 155.0000000000000000, -15.00000000000002487 ) ) ;
#24228=CARTESIAN_POINT ( 'NONE',  ( 39.89999999453763735, 150.2886644046228639, -14.50000000000000888 ) ) ;
#24236=ORIENTED_EDGE ( 'NONE', *, *, #16236, .F. ) ;
#24238=CARTESIAN_POINT ( 'NONE',  ( 78.78867513459481131, 155.0000000000000000, -15.00000000000002487 ) ) ;
#24244=CARTESIAN_POINT ( 'NONE',  ( 35.72499999726881015, 169.8198683612136222, 4.815267126137181997 ) ) ;
#24246=CARTESIAN_POINT ( 'NONE',  ( 37.07499999726881157, 141.7447067706911810, -9.630534252274385310 ) ) ;
#24250=CARTESIAN_POINT ( 'NONE',  ( 54.80000000000000426, 167.3344367211045096, -8.961492836873482304 ) ) ;
#24252=CARTESIAN_POINT ( 'NONE',  ( 33.71132485994280614, 155.0000000000000000, -15.00000000000002487 ) ) ;
#24253=CARTESIAN_POINT ( 'NONE',  ( 55.62499999726881583, 171.3844434931184253, -7.942151717890132712E-15 ) ) ;
#24256=CARTESIAN_POINT ( 'NONE',  ( 64.72499999726881015, 140.1801316387863778, -4.815267126137194431 ) ) ;
#24257=CARTESIAN_POINT ( 'NONE',  ( 73.37499999726881583, 155.0000000000000000, -15.58253175000000823 ) ) ;
#24269=VERTEX_POINT ( 'NONE', #24455 ) ;
#24275=CARTESIAN_POINT ( 'NONE',  ( 79.62499999726881583, 171.3844434931184253, -7.942151717890134290E-15 ) ) ;
#24277=DIRECTION ( 'NONE',  ( -1.000000000000000000, 0.000000000000000000, 0.000000000000000000 ) ) ;
#24279=CARTESIAN_POINT ( 'NONE',  ( 68.72499999726881015, 140.1801316387863778, -4.815267126137194431 ) ) ;
#24287=CARTESIAN_POINT ( 'NONE',  ( 34.89999999999999858, 168.7903194862797420, -4.480746418436745593 ) ) ;
#24297=CARTESIAN_POINT ( 'NONE',  ( 44.02499999726881441, 160.0630714827496206, 15.58253174999999224 ) ) ;
#24304=CARTESIAN_POINT ( 'NONE',  ( 84.29999999453761461, 167.3344367211045096, -8.961492836873482304 ) ) ;
#24308=EDGE_CURVE ( 'NONE', #27342, #9113, #22064, .T. ) ;
#24315=CARTESIAN_POINT ( 'NONE',  ( 70.17499999726881299, 164.1591823560292198, 12.60653300113718167 ) ) ;
#24320=CARTESIAN_POINT ( 'NONE',  ( 79.77499999726880731, 169.8198683612136222, -4.815267126137197984 ) ) ;
#24321=CARTESIAN_POINT ( 'NONE',  ( 76.71132485994280614, 155.0000000000000000, 15.00000000000001243 ) ) ;
#24324=SURFACE_STYLE_FILL_AREA ( #28945 ) ;
#24326=CARTESIAN_POINT ( 'NONE',  ( 67.37499999726881583, 155.0000000000000000, -15.58253175000000823 ) ) ;
#24327=ORIENTED_EDGE ( 'NONE', *, *, #20169, .T. ) ;
#24336=CARTESIAN_POINT ( 'NONE',  ( 82.77499999726880731, 140.1801316387863778, 4.815267126137185549 ) ) ;
#24339=VECTOR ( 'NONE', #6714, 1000.000000000000000 ) ;
#24341=CARTESIAN_POINT ( 'NONE',  ( 40.12499999726880873, 155.0000000000000000, 15.58253174999999402 ) ) ;
#24342=CARTESIAN_POINT ( 'NONE',  ( 36.48867513459482836, 142.2402378747194405, -9.270509831248439525 ) ) ;
#24346=CARTESIAN_POINT ( 'NONE',  ( 65.07499999726881867, 141.7447067706911810, -9.630534252274385310 ) ) ;
#24353=CARTESIAN_POINT ( 'NONE',  ( 85.78867513459481131, 155.0000000000000000, 15.00000000000001243 ) ) ;
#24356=CARTESIAN_POINT ( 'NONE',  ( 66.69999999453763451, 167.3344367211045096, 8.961492836873468093 ) ) ;
#24357=ORIENTED_EDGE ( 'NONE', *, *, #11401, .T. ) ;
#24363=CYLINDRICAL_SURFACE ( 'NONE', #8512, 15.00000000000001776 ) ;
#24377=CARTESIAN_POINT ( 'NONE',  ( 50.97499999726881725, 140.1801316387863778, -4.815267126137194431 ) ) ;
#24380=CARTESIAN_POINT ( 'NONE',  ( 57.42499999726880588, 168.2552932293087906, -9.630534252274385310 ) ) ;
#24382=CARTESIAN_POINT ( 'NONE',  ( 58.78867513459481842, 155.0000000000000000, -15.00000000000002487 ) ) ;
#24385=CARTESIAN_POINT ( 'NONE',  ( 58.97499999726881015, 140.1801316387863778, -4.815267126137194431 ) ) ;
#24387=CARTESIAN_POINT ( 'NONE',  ( 47.08867513459482979, 167.7597621252805880, -9.270509831248443078 ) ) ;
#24390=CARTESIAN_POINT ( 'NONE',  ( 72.29999999999999716, 146.4771138417591203, -11.73074641843674470 ) ) ;
#24395=LINE ( 'NONE', #1061, #16737 ) ;
#24396=CARTESIAN_POINT ( 'NONE',  ( 47.17499999726881299, 145.8408176439707802, -12.60653300113719588 ) ) ;
#24400=CARTESIAN_POINT ( 'NONE',  ( 79.22499999726879594, 160.0630714827496206, -15.58253175000000823 ) ) ;
#24401=VERTEX_POINT ( 'NONE', #16608 ) ;
#24403=CARTESIAN_POINT ( 'NONE',  ( 46.59999999453762598, 168.7903194862797420, 4.480746418436729606 ) ) ;
#24414=PRODUCT_DEFINITION_CONTEXT ( 'detailed design', #22452, 'design' ) ;
#24422=CARTESIAN_POINT ( 'NONE',  ( 40.62499999726880873, 138.6155565068815463, -3.929120461958505118E-15 ) ) ;
#24425=CARTESIAN_POINT ( 'NONE',  ( 42.47499999726880304, 149.9369285172503510, 15.58253174999999580 ) ) ;
#24429=CARTESIAN_POINT ( 'NONE',  ( 56.50000000000000000, 155.0000000000000000, -14.50000000000000711 ) ) ;
#24434=CARTESIAN_POINT ( 'NONE',  ( 58.32499999726881157, 145.8408176439707802, 12.60653300113718345 ) ) ;
#24437=CARTESIAN_POINT ( 'NONE',  ( 67.52499999726880731, 169.8198683612136222, -4.815267126137197984 ) ) ;
#24438=CARTESIAN_POINT ( 'NONE',  ( 79.27499999726880731, 149.9369285172503510, -15.58253175000000823 ) ) ;
#24455=CARTESIAN_POINT ( 'NONE',  ( 43.71132485994280614, 155.0000000000000000, -15.00000000000002487 ) ) ;
#24458=CARTESIAN_POINT ( 'NONE',  ( 86.32499999726880446, 145.8408176439707802, 12.60653300113718345 ) ) ;
#24462=CARTESIAN_POINT ( 'NONE',  ( 76.12499999726881583, 155.0000000000000000, 15.58253174999999402 ) ) ;
#24464=CARTESIAN_POINT ( 'NONE',  ( 75.18867513459481700, 169.2658477444273331, -4.635254915624224203 ) ) ;
#24466=CARTESIAN_POINT ( 'NONE',  ( 36.60000000000000853, 159.7113355953771077, -14.50000000000000888 ) ) ;
#24474=CARTESIAN_POINT ( 'NONE',  ( 51.72499999726881725, 169.8198683612136222, 4.815267126137181997 ) ) ;
#24476=CARTESIAN_POINT ( 'NONE',  ( 32.50000000000000000, 155.0000000000000000, 15.00000000000001243 ) ) ;
#24481=CARTESIAN_POINT ( 'NONE',  ( 84.09999999453761177, 159.7113355953771077, -14.50000000000000888 ) ) ;
#24490=CARTESIAN_POINT ( 'NONE',  ( 70.67499999726881299, 141.7447067706911810, 9.630534252274376428 ) ) ;
#24493=ORIENTED_EDGE ( 'NONE', *, *, #19093, .T. ) ;
#24494=CARTESIAN_POINT ( 'NONE',  ( 84.27499999726879309, 160.0630714827496206, 15.58253174999999224 ) ) ;
#24501=CARTESIAN_POINT ( 'NONE',  ( 68.77499999726880731, 140.1801316387863778, 4.815267126137185549 ) ) ;
#24503=CARTESIAN_POINT ( 'NONE',  ( 36.31132485994280046, 169.2658477444273331, 4.635254915624208216 ) ) ;
#24511=CARTESIAN_POINT ( 'NONE',  ( 66.78867513459482552, 155.0000000000000000, -15.00000000000002487 ) ) ;
#24513=CARTESIAN_POINT ( 'NONE',  ( 44.92499999726880588, 145.8408176439707802, -12.60653300113719588 ) ) ;
#24527=CARTESIAN_POINT ( 'NONE',  ( 68.59999999453762598, 168.7903194862797420, 4.480746418436729606 ) ) ;
#24533=EDGE_CURVE ( 'NONE', #5476, #6338, #33472, .T. ) ;
#24534=CYLINDRICAL_SURFACE ( 'NONE', #10156, 15.00000000000001776 ) ;
#24545=CARTESIAN_POINT ( 'NONE',  ( 48.67499999726881299, 141.7447067706911810, 9.630534252274376428 ) ) ;
#24547=CARTESIAN_POINT ( 'NONE',  ( 55.52499999726881441, 169.8198683612136222, -4.815267126137197984 ) ) ;
#24550=AXIS2_PLACEMENT_3D ( 'NONE', #25437, #9431, #12324 ) ;
#24553=CARTESIAN_POINT ( 'NONE',  ( 61.97499999726881015, 169.8198683612136222, 4.815267126137181997 ) ) ;
#24555=CARTESIAN_POINT ( 'NONE',  ( 87.50000000000001421, 155.0000000000000000, 15.00000000000001243 ) ) ;
#24558=CARTESIAN_POINT ( 'NONE',  ( 80.30000000000001137, 146.4771138417591203, -11.73074641843674470 ) ) ;
#24559=CARTESIAN_POINT ( 'NONE',  ( 40.58867513459482268, 146.1832212156128890, -12.13525491562423042 ) ) ;
#24562=CARTESIAN_POINT ( 'NONE',  ( 47.37499999726880873, 155.0000000000000000, -15.58253175000000823 ) ) ;
#24565=CARTESIAN_POINT ( 'NONE',  ( 79.02499999726879309, 149.9369285172503510, -15.58253175000000823 ) ) ;
#24569=CARTESIAN_POINT ( 'NONE',  ( 46.29999999453762882, 167.3344367211045096, -8.961492836873482304 ) ) ;
#24574=ORIENTED_EDGE ( 'NONE', *, *, #11903, .F. ) ;
#24580=CARTESIAN_POINT ( 'NONE',  ( 125.5000000000000000, 155.0000000000000000, -100.0000000000000284 ) ) ;
#24584=EDGE_CURVE ( 'NONE', #5650, #23379, #30914, .T. ) ;
#24590=CARTESIAN_POINT ( 'NONE',  ( 37.52499999726881441, 169.8198683612136222, -4.815267126137197984 ) ) ;
#24593=CARTESIAN_POINT ( 'NONE',  ( 38.57499999726881157, 145.8408176439707802, 12.60653300113718345 ) ) ;
#24598=CARTESIAN_POINT ( 'NONE',  ( 55.19999999999998863, 167.3344367211045096, 8.961492836873468093 ) ) ;
#24599=CARTESIAN_POINT ( 'NONE',  ( 59.71132485994280614, 155.0000000000000000, -15.00000000000002487 ) ) ;
#24603=CARTESIAN_POINT ( 'NONE',  ( 59.42499999726882010, 168.2552932293087906, -9.630534252274385310 ) ) ;
#24608=CARTESIAN_POINT ( 'NONE',  ( 83.47499999726881015, 160.0630714827496206, -15.58253175000000823 ) ) ;
#24611=CARTESIAN_POINT ( 'NONE',  ( 71.78867513459482552, 155.0000000000000000, 15.00000000000001243 ) ) ;
#24613=ORIENTED_EDGE ( 'NONE', *, *, #8927, .F. ) ;
#24623=CARTESIAN_POINT ( 'NONE',  ( 63.41132485994281609, 142.2402378747194405, -9.270509831248439525 ) ) ;
#24628=CARTESIAN_POINT ( 'NONE',  ( 83.52499999726880731, 169.8198683612136222, -4.815267126137197984 ) ) ;
#24633=CARTESIAN_POINT ( 'NONE',  ( 73.92499999726881299, 164.1591823560292198, 12.60653300113718167 ) ) ;
#24635=CARTESIAN_POINT ( 'NONE',  ( 75.28867513459483973, 170.7719333635740497, -7.904646289410545231E-15 ) ) ;
#24636=CARTESIAN_POINT ( 'NONE',  ( 32.50000000000000000, 155.0000000000000000, -14.50000000000000711 ) ) ;
#24644=CARTESIAN_POINT ( 'NONE',  ( 52.32499999726881157, 145.8408176439707802, 12.60653300113718345 ) ) ;
#24652=CARTESIAN_POINT ( 'NONE',  ( 85.79999999453762882, 146.4771138417591203, -11.73074641843674470 ) ) ;
#24663=CARTESIAN_POINT ( 'NONE',  ( 68.87499999726881583, 138.6155565068815463, -3.929120461958505118E-15 ) ) ;
#24666=CARTESIAN_POINT ( 'NONE',  ( 81.97499999726881015, 169.8198683612136222, 4.815267126137181997 ) ) ;
#24672=CARTESIAN_POINT ( 'NONE',  ( 71.57499999726881867, 164.1591823560292198, -12.60653300113719766 ) ) ;
#24675=( BOUNDED_CURVE ( )  B_SPLINE_CURVE ( 2, ( #12271, #19936, #9720, #33228, #9379, #29999, #30169, #23004, #22498, #7001, #12446 ),
 .UNSPECIFIED., .F., .T. ) 
 B_SPLINE_CURVE_WITH_KNOTS ( ( 3, 2, 2, 2, 2, 3 ),
 ( 0.4107142857142856984, 0.4142857142857143127, 0.4178571428571428714, 0.4214285714285714302, 0.4249999999999999889, 0.4285714285714285476 ),
 .UNSPECIFIED. ) 
 CURVE ( )  GEOMETRIC_REPRESENTATION_ITEM ( )  RATIONAL_B_SPLINE_CURVE ( ( 1.000000000000000000, 0.9510565162951534202, 1.000000000000000000, 0.9510565162951534202, 1.000000000000000000, 0.9510565162951534202, 1.000000000000000000, 0.9510565162951534202, 1.000000000000000000, 0.9510565162951534202, 1.000000000000000000 ) ) 
 REPRESENTATION_ITEM ( '' )  );
#24677=CARTESIAN_POINT ( 'NONE',  ( 55.71132485994280614, 155.0000000000000000, -15.00000000000002487 ) ) ;
#24684=AXIS2_PLACEMENT_3D ( 'NONE', #11091, #21471, #26573 ) ;
#24687=CARTESIAN_POINT ( 'NONE',  ( 41.92499999726881299, 164.1591823560292198, 12.60653300113718167 ) ) ;
#24689=CARTESIAN_POINT ( 'NONE',  ( 87.50000000000000000, 157.6678010926102047, -15.23241260079973536 ) ) ;
#24694=CARTESIAN_POINT ( 'NONE',  ( 127.5000000000000000, 80.04668119422662187, 74.95331880577468553 ) ) ;
#24699=CARTESIAN_POINT ( 'NONE',  ( 66.39999999453763735, 168.7903194862797420, -4.480746418436745593 ) ) ;
#24710=CARTESIAN_POINT ( 'NONE',  ( 58.18867513459483121, 140.7341522555726669, 4.635254915624211769 ) ) ;
#24714=EDGE_CURVE ( 'NONE', #18876, #6936, #20246, .T. ) ;
#24717=CARTESIAN_POINT ( 'NONE',  ( 53.07499999726880446, 141.7447067706911810, -9.630534252274387086 ) ) ;
#24720=CARTESIAN_POINT ( 'NONE',  ( 67.61132485994281183, 150.1262045565062806, -14.99999999999993072 ) ) ;
#24723=CARTESIAN_POINT ( 'NONE',  ( 61.87499999726881583, 171.3844434931184253, -7.942151717890132712E-15 ) ) ;
#24725=DIRECTION ( 'NONE',  ( 0.000000000000000000, 0.000000000000000000, -1.000000000000000000 ) ) ;
#24731=CARTESIAN_POINT ( 'NONE',  ( 79.80000000000002558, 142.6655632788954620, 8.961492836873471646 ) ) ;
#24736=CARTESIAN_POINT ( 'NONE',  ( 41.37499999726880873, 155.0000000000000000, -15.58253175000000823 ) ) ;
#24738=CARTESIAN_POINT ( 'NONE',  ( 81.92499999726882720, 164.1591823560292198, 12.60653300113718167 ) ) ;
#24739=ADVANCED_FACE ( 'NONE', ( #5966 ), #16526, .T. ) ;
#24742=CARTESIAN_POINT ( 'NONE',  ( 46.09999999453762598, 159.7113355953771077, -14.50000000000000888 ) ) ;
#24743=ORIENTED_EDGE ( 'NONE', *, *, #21846, .T. ) ;
#24751=EDGE_CURVE ( 'NONE', #20089, #31949, #31459, .T. ) ;
#24761=ORIENTED_EDGE ( 'NONE', *, *, #27431, .T. ) ;
#24762=CARTESIAN_POINT ( 'NONE',  ( 37.22499999726881015, 160.0630714827496206, -15.58253175000000823 ) ) ;
#24763=CARTESIAN_POINT ( 'NONE',  ( 39.28867513459483263, 170.7719333635740497, -7.904646289410545231E-15 ) ) ;
#24765=CARTESIAN_POINT ( 'NONE',  ( 40.37499999726880873, 155.0000000000000000, 15.58253174999999402 ) ) ;
#24768=CARTESIAN_POINT ( 'NONE',  ( 63.60000000000000142, 150.2886644046228639, 14.49999999999999645 ) ) ;
#24773=CARTESIAN_POINT ( 'NONE',  ( 63.22499999726881725, 160.0630714827496206, -15.58253175000000823 ) ) ;
#24775=EDGE_LOOP ( 'NONE', ( #11661, #30156, #14014, #6044 ) ) ;
#24777=CARTESIAN_POINT ( 'NONE',  ( 85.57499999726880446, 164.1591823560292198, -12.60653300113719766 ) ) ;
#24780=ADVANCED_FACE ( 'NONE', ( #18763 ), #19089, .F. ) ;
#24782=CARTESIAN_POINT ( 'NONE',  ( 52.88867513459483405, 159.8737954434939752, -14.99999999999974420 ) ) ;
#24793=VERTEX_POINT ( 'NONE', #695 ) ;
#24797=VERTEX_POINT ( 'NONE', #26749 ) ;
#24798=CARTESIAN_POINT ( 'NONE',  ( 86.22499999726882436, 149.9369285172503510, 15.58253174999999580 ) ) ;
#24800=CARTESIAN_POINT ( 'NONE',  ( 69.01132485994283172, 142.2402378747194405, 9.270509831248432420 ) ) ;
#24801=CARTESIAN_POINT ( 'NONE',  ( 73.72499999726881015, 169.8198683612136222, 4.815267126137181997 ) ) ;
#24802=CYLINDRICAL_SURFACE ( 'NONE', #16484, 15.00000000000001776 ) ;
#24805=CARTESIAN_POINT ( 'NONE',  ( 41.30000000000000426, 163.5228861582408797, 11.73074641843673049 ) ) ;
#24807=DIRECTION ( 'NONE',  ( 1.000000000000000000, 0.000000000000000000, 0.000000000000000000 ) ) ;
#24809=CARTESIAN_POINT ( 'NONE',  ( 32.50000000000000000, 155.0000000000000000, 15.00000000000001243 ) ) ;
#24810=CARTESIAN_POINT ( 'NONE',  ( 53.92499999726881299, 164.1591823560292198, 12.60653300113718167 ) ) ;
#24817=CARTESIAN_POINT ( 'NONE',  ( 84.59999999453762598, 168.7903194862797420, 4.480746418436729606 ) ) ;
#24820=( BOUNDED_CURVE ( )  B_SPLINE_CURVE ( 2, ( #11962, #19962, #22526, #32569, #25075, #12130, #11788, #16897, #22181, #14683, #1570 ),
 .UNSPECIFIED., .F., .F. ) 
 B_SPLINE_CURVE_WITH_KNOTS ( ( 3, 2, 2, 2, 2, 3 ),
 ( 0.5714285714285712858, 0.5749999999999998446, 0.5785714285714285143, 0.5821428571428569620, 0.5857142857142855208, 0.5892857142857140795 ),
 .UNSPECIFIED. ) 
 CURVE ( )  GEOMETRIC_REPRESENTATION_ITEM ( )  RATIONAL_B_SPLINE_CURVE ( ( 1.000000000000001554, 0.9510565162951518658, 1.000000000000000000, 0.9510565162951534202, 1.000000000000000000, 0.9510565162951534202, 1.000000000000000000, 0.9510565162951534202, 1.000000000000000000, 0.9510565162951564178, 0.9999999999999970024 ) ) 
 REPRESENTATION_ITEM ( '' )  );
#24826=CARTESIAN_POINT ( 'NONE',  ( 69.77499999726880731, 169.8198683612136222, -4.815267126137197984 ) ) ;
#24830=CARTESIAN_POINT ( 'NONE',  ( 84.47499999726883857, 149.9369285172503510, 15.58253174999999580 ) ) ;
#24834=DIRECTION ( 'NONE',  ( -1.000000000000000000, 0.000000000000000000, 0.000000000000000000 ) ) ;
#24839=LINE ( 'NONE', #15879, #5265 ) ;
#24844=CARTESIAN_POINT ( 'NONE',  ( 71.31132485994280046, 140.7341522555726669, -4.635254915624220651 ) ) ;
#24848=CARTESIAN_POINT ( 'NONE',  ( 42.12499999726881583, 155.0000000000000000, 15.58253174999999402 ) ) ;
#24850=CARTESIAN_POINT ( 'NONE',  ( 87.50000000000000000, 158.3354728270139447, -15.12515773927365181 ) ) ;
#24860=CARTESIAN_POINT ( 'NONE',  ( 69.09999999453764019, 150.2886644046228639, 14.49999999999999645 ) ) ;
#24877=CARTESIAN_POINT ( 'NONE',  ( 49.77499999726880731, 169.8198683612136222, -4.815267126137197984 ) ) ;
#24884=DIRECTION ( 'NONE',  ( 1.000000000000000000, 0.000000000000000000, 0.000000000000000000 ) ) ;
#24886=CARTESIAN_POINT ( 'NONE',  ( 60.07499999726879736, 168.2552932293087906, 9.630534252274372875 ) ) ;
#24888=CYLINDRICAL_SURFACE ( 'NONE', #14346, 2.149999999999984812 ) ;
#24892=CARTESIAN_POINT ( 'NONE',  ( 77.89999999999999147, 141.2096805137202580, 4.480746418436733158 ) ) ;
#24894=CARTESIAN_POINT ( 'NONE',  ( 125.5000000000000000, 81.56696077377769427, 76.47359838532574372 ) ) ;
#24897=CARTESIAN_POINT ( 'NONE',  ( 47.47499999726881015, 160.0630714827496206, -15.58253175000000823 ) ) ;
#24899=CARTESIAN_POINT ( 'NONE',  ( 86.02499999726880731, 160.0630714827496206, 15.58253174999999402 ) ) ;
#24902=CARTESIAN_POINT ( 'NONE',  ( 44.79999999453762882, 163.5228861582408797, 11.73074641843673049 ) ) ;
#24909=ORIENTED_EDGE ( 'NONE', *, *, #31152, .T. ) ;
#24917=DIRECTION ( 'NONE',  ( 1.000000000000000000, 0.000000000000000000, 0.000000000000000000 ) ) ;
#24925=CARTESIAN_POINT ( 'NONE',  ( 35.22499999726881015, 160.0630714827496206, -15.58253175000000823 ) ) ;
#24926=CARTESIAN_POINT ( 'NONE',  ( 40.71132485994280614, 155.0000000000000000, 15.00000000000001243 ) ) ;
#24927=EDGE_CURVE ( 'NONE', #19762, #9319, #28440, .T. ) ;
#24930=CARTESIAN_POINT ( 'NONE',  ( 37.87499999726880873, 171.3844434931184253, -7.942151717890132712E-15 ) ) ;
#24931=CYLINDRICAL_SURFACE ( 'NONE', #503, 15.00000000000001776 ) ;
#24936=CARTESIAN_POINT ( 'NONE',  ( 60.50000000000000000, 155.0000000000000000, -14.50000000000000711 ) ) ;
#24941=EDGE_CURVE ( 'NONE', #8938, #16276, #2625, .T. ) ;
#24942=CARTESIAN_POINT ( 'NONE',  ( 65.12499999726881583, 155.0000000000000000, -15.58253175000000823 ) ) ;
#24946=CARTESIAN_POINT ( 'NONE',  ( 84.67499999726881299, 141.7447067706911810, 9.630534252274376428 ) ) ;
#24950=ORIENTED_EDGE ( 'NONE', *, *, #757, .T. ) ;
#24955=VECTOR ( 'NONE', #24982, 1000.000000000000000 ) ;
#24958=CARTESIAN_POINT ( 'NONE',  ( 66.48867513459482836, 142.2402378747194405, -9.270509831248439525 ) ) ;
#24968=CARTESIAN_POINT ( 'NONE',  ( 87.32499999726880446, 164.1591823560292198, -12.60653300113719766 ) ) ;
#24971=CARTESIAN_POINT ( 'NONE',  ( 74.02499999726879309, 160.0630714827496206, 15.58253174999999402 ) ) ;
#24974=ADVANCED_FACE ( 'NONE', ( #12093 ), #1874, .T. ) ;
#24975=CARTESIAN_POINT ( 'NONE',  ( 75.08867513459483689, 167.7597621252805880, -9.270509831248443078 ) ) ;
#24976=CARTESIAN_POINT ( 'NONE',  ( 40.70000000000000284, 163.5228861582408797, -11.73074641843674470 ) ) ;
#24979=EDGE_CURVE ( 'NONE', #9541, #31511, #4122, .T. ) ;
#24981=CARTESIAN_POINT ( 'NONE',  ( 32.50000000000000000, 155.0000000000000000, 15.00000000000001243 ) ) ;
#24982=DIRECTION ( 'NONE',  ( 1.000000000000000000, 0.000000000000000000, 0.000000000000000000 ) ) ;
#24984=CARTESIAN_POINT ( 'NONE',  ( 51.82499999726881157, 168.2552932293087906, 9.630534252274372875 ) ) ;
#24985=CARTESIAN_POINT ( 'NONE',  ( 62.27499999726880020, 160.0630714827496206, 15.58253174999999402 ) ) ;
#25000=CARTESIAN_POINT ( 'NONE',  ( 70.37499999726881583, 155.0000000000000000, 15.58253174999999402 ) ) ;
#25003=ORIENTED_EDGE ( 'NONE', *, *, #25333, .T. ) ;
#25004=CARTESIAN_POINT ( 'NONE',  ( 85.77499999726880731, 169.8198683612136222, -4.815267126137197984 ) ) ;
#25019=CARTESIAN_POINT ( 'NONE',  ( 67.18867513459483121, 169.2658477444273331, -4.635254915624224203 ) ) ;
#25023=CARTESIAN_POINT ( 'NONE',  ( 43.32499999726881157, 164.1591823560292198, -12.60653300113719766 ) ) ;
#25025=CARTESIAN_POINT ( 'NONE',  ( 87.50000000000008527, 146.2573930672651841, -12.23674163361536316 ) ) ;
#25027=LINE ( 'NONE', #30302, #6973 ) ;
#25035=CARTESIAN_POINT ( 'NONE',  ( 64.99999999453761745, 155.0000000000000000, 14.49999999999999467 ) ) ;
#25045=CARTESIAN_POINT ( 'NONE',  ( 87.50000000000000000, 166.7234620888311838, -10.31567525671095531 ) ) ;
#25049=CARTESIAN_POINT ( 'NONE',  ( 85.51132485994281751, 146.1832212156128890, -12.13525491562423042 ) ) ;
#25051=CARTESIAN_POINT ( 'NONE',  ( 55.47499999726881015, 160.0630714827496206, -15.58253175000000823 ) ) ;
#25056=CARTESIAN_POINT ( 'NONE',  ( 67.37499999726881583, 155.0000000000000000, -15.58253175000000823 ) ) ;
#25058=CARTESIAN_POINT ( 'NONE',  ( 70.48867513459484258, 142.2402378747194405, -9.270509831248439525 ) ) ;
#25062=CARTESIAN_POINT ( 'NONE',  ( 78.00000000000000000, 139.7537977485451393, -4.138211985947621020E-15 ) ) ;
#25066=CARTESIAN_POINT ( 'NONE',  ( 41.57499999726881157, 164.1591823560292198, -12.60653300113719766 ) ) ;
#25068=CARTESIAN_POINT ( 'NONE',  ( 82.22499999726882436, 149.9369285172503510, 15.58253174999999580 ) ) ;
#25071=CARTESIAN_POINT ( 'NONE',  ( 45.49999999453763166, 139.7537977485451393, -4.138211985947621020E-15 ) ) ;
#25075=CARTESIAN_POINT ( 'NONE',  ( 66.11132485994281183, 169.2658477444273331, -4.635254915624224203 ) ) ;
#25080=DIRECTION ( 'NONE',  ( 0.000000000000000000, 0.000000000000000000, 1.000000000000000000 ) ) ;
#25083=CARTESIAN_POINT ( 'NONE',  ( 32.50000000000000000, 155.0000000000000000, -6.938893903907228378E-15 ) ) ;
#25085=CARTESIAN_POINT ( 'NONE',  ( 36.67499999726879878, 141.7447067706911810, 9.630534252274376428 ) ) ;
#25087=CARTESIAN_POINT ( 'NONE',  ( 41.22499999726881015, 160.0630714827496206, -15.58253175000000823 ) ) ;
#25091=CARTESIAN_POINT ( 'NONE',  ( 39.57499999726881157, 164.1591823560292198, -12.60653300113719766 ) ) ;
#25095=CARTESIAN_POINT ( 'NONE',  ( 62.30000000000000426, 146.4771138417591203, -11.73074641843674470 ) ) ;
#25096=CARTESIAN_POINT ( 'NONE',  ( 64.01132485994281751, 167.7597621252805880, -9.270509831248443078 ) ) ;
#25098=CYLINDRICAL_SURFACE ( 'NONE', #32489, 15.00000000000001776 ) ;
#25101=EDGE_CURVE ( 'NONE', #15366, #15702, #19145, .T. ) ;
#25102=CARTESIAN_POINT ( 'NONE',  ( 65.52499999726880731, 169.8198683612136222, -4.815267126137197984 ) ) ;
#25104=VERTEX_POINT ( 'NONE', #4255 ) ;
#25106=CARTESIAN_POINT ( 'NONE',  ( 80.57499999726880446, 145.8408176439707802, 12.60653300113718345 ) ) ;
#25113=DIRECTION ( 'NONE',  ( 0.000000000000000000, 0.000000000000000000, 1.000000000000000000 ) ) ;
#25117=CARTESIAN_POINT ( 'NONE',  ( 127.5000000000000000, 229.9533188057739039, -74.95331880577418815 ) ) ;
#25121=ORIENTED_EDGE ( 'NONE', *, *, #19289, .F. ) ;
#25122=CARTESIAN_POINT ( 'NONE',  ( 84.92499999726882720, 145.8408176439707802, -12.60653300113719588 ) ) ;
#25124=CARTESIAN_POINT ( 'NONE',  ( 69.41132485994282320, 142.2402378747194405, -9.270509831248439525 ) ) ;
#25126=CARTESIAN_POINT ( 'NONE',  ( 74.52499999726880731, 140.1801316387863778, 4.815267126137185549 ) ) ;
#25131=VECTOR ( 'NONE', #19533, 1000.000000000000000 ) ;
#25132=CARTESIAN_POINT ( 'NONE',  ( 43.39999999999999147, 159.7113355953771077, 14.49999999999999289 ) ) ;
#25137=CARTESIAN_POINT ( 'NONE',  ( 77.98867513459482836, 146.1832212156128890, 12.13525491562421976 ) ) ;
#25138=CARTESIAN_POINT ( 'NONE',  ( 32.50000000000000000, 155.0000000000000000, 15.00000000000001243 ) ) ;
#25139=CARTESIAN_POINT ( 'NONE',  ( 53.32499999726881157, 164.1591823560292198, -12.60653300113719766 ) ) ;
#25140=CARTESIAN_POINT ( 'NONE',  ( 62.17499999726882010, 164.1591823560292198, 12.60653300113718167 ) ) ;
#25149=CARTESIAN_POINT ( 'NONE',  ( 82.81132485994282888, 150.1262045565062806, 14.99999999999992006 ) ) ;
#25157=CARTESIAN_POINT ( 'NONE',  ( 80.57499999726880446, 145.8408176439707802, 12.60653300113718345 ) ) ;
#25161=EDGE_CURVE ( 'NONE', #12632, #33078, #22992, .T. ) ;
#25162=CARTESIAN_POINT ( 'NONE',  ( 84.07499999726879025, 168.2552932293087906, 9.630534252274372875 ) ) ;
#25165=ADVANCED_FACE ( 'NONE', ( #18052 ), #28446, .T. ) ;
#25166=CARTESIAN_POINT ( 'NONE',  ( 54.02499999726880020, 160.0630714827496206, 15.58253174999999402 ) ) ;
#25170=CARTESIAN_POINT ( 'NONE',  ( 84.78867513459482552, 155.0000000000000000, -15.00000000000002487 ) ) ;
#25171=AXIS2_PLACEMENT_3D ( 'NONE', #14293, #14128, #30141 ) ;
#25173=CARTESIAN_POINT ( 'NONE',  ( 86.21132485994283456, 170.7719333635740497, -7.904646289410545231E-15 ) ) ;
#25180=CARTESIAN_POINT ( 'NONE',  ( 47.52499999726881441, 169.8198683612136222, -4.815267126137197984 ) ) ;
#25184=CARTESIAN_POINT ( 'NONE',  ( 82.08867513459485110, 142.2402378747194405, 9.270509831248432420 ) ) ;
#25188=VECTOR ( 'NONE', #1245, 1000.000000000000000 ) ;
#25190=CARTESIAN_POINT ( 'NONE',  ( 60.78867513459481842, 155.0000000000000000, -15.00000000000002487 ) ) ;
#25193=CARTESIAN_POINT ( 'NONE',  ( 74.39999999453763735, 168.7903194862797420, -4.480746418436745593 ) ) ;
#25194=ORIENTED_EDGE ( 'NONE', *, *, #1625, .F. ) ;
#25202=AXIS2_PLACEMENT_3D ( 'NONE', #91, #25472, #20530 ) ;
#25204=EDGE_LOOP ( 'NONE', ( #21226, #2036, #31013, #16435 ) ) ;
#25211=AXIS2_PLACEMENT_3D ( 'NONE', #17081, #4808, #14688 ) ;
#25213=DIRECTION ( 'NONE',  ( 0.000000000000000000, 0.000000000000000000, 1.000000000000000000 ) ) ;
#25216=CARTESIAN_POINT ( 'NONE',  ( 57.77499999726881441, 169.8198683612136222, -4.815267126137197984 ) ) ;
#25221=LINE ( 'NONE', #20276, #31504 ) ;
#25223=CARTESIAN_POINT ( 'NONE',  ( 63.17499999726880588, 145.8408176439707802, -12.60653300113719588 ) ) ;
#25225=DIRECTION ( 'NONE',  ( 1.000000000000000000, 0.000000000000000000, 0.000000000000000000 ) ) ;
#25226=( BOUNDED_CURVE ( )  B_SPLINE_CURVE ( 2, ( #3037, #31498, #23491, #29265, #8323, #19040, #13421, #23817, #2725, #24149, #158 ),
 .UNSPECIFIED., .F., .F. ) 
 B_SPLINE_CURVE_WITH_KNOTS ( ( 3, 2, 2, 2, 2, 3 ),
 ( 0.6785714285714283811, 0.6821428571428569398, 0.6857142857142854986, 0.6892857142857141683, 0.6928571428571427271, 0.6964285714285712858 ),
 .UNSPECIFIED. ) 
 CURVE ( )  GEOMETRIC_REPRESENTATION_ITEM ( )  RATIONAL_B_SPLINE_CURVE ( ( 1.000000000000003109, 0.9510565162951504226, 1.000000000000000000, 0.9510565162951534202, 1.000000000000000000, 0.9510565162951534202, 1.000000000000000000, 0.9510565162951534202, 1.000000000000000000, 0.9510565162951549745, 0.9999999999999984457 ) ) 
 REPRESENTATION_ITEM ( '' )  );
#25230=CARTESIAN_POINT ( 'NONE',  ( 79.60000000000000853, 150.2886644046228639, 14.49999999999999645 ) ) ;
#25235=CARTESIAN_POINT ( 'NONE',  ( 51.97499999726881725, 169.8198683612136222, 4.815267126137181997 ) ) ;
#25237=CARTESIAN_POINT ( 'NONE',  ( 82.52499999726880731, 140.1801316387863778, 4.815267126137185549 ) ) ;
#25240=CARTESIAN_POINT ( 'NONE',  ( 53.39999999453763024, 141.2096805137202580, 4.480746418436733158 ) ) ;
#25252=LINE ( 'NONE', #14856, #8371 ) ;
#25255=CARTESIAN_POINT ( 'NONE',  ( 32.50000000000000000, 155.0000000000000000, 15.00000000000001243 ) ) ;
#25257=CARTESIAN_POINT ( 'NONE',  ( 34.97499999726881015, 140.1801316387863778, -4.815267126137194431 ) ) ;
#25259=CARTESIAN_POINT ( 'NONE',  ( 44.72499999726881015, 140.1801316387863778, -4.815267126137194431 ) ) ;
#25264=CARTESIAN_POINT ( 'NONE',  ( 49.47499999726881725, 160.0630714827496206, -15.58253175000000823 ) ) ;
#25268=CARTESIAN_POINT ( 'NONE',  ( 63.39999999999999858, 159.7113355953771077, 14.49999999999999289 ) ) ;
#25270=CARTESIAN_POINT ( 'NONE',  ( 64.41132485994282320, 167.7597621252805880, 9.270509831248428867 ) ) ;
#25273=CARTESIAN_POINT ( 'NONE',  ( 33.87499999726881583, 171.3844434931184253, -7.942151717890132712E-15 ) ) ;
#25275=CARTESIAN_POINT ( 'NONE',  ( 61.82499999726881157, 168.2552932293087906, 9.630534252274372875 ) ) ;
#25280=CARTESIAN_POINT ( 'NONE',  ( 85.07499999726880446, 141.7447067706911810, -9.630534252274385310 ) ) ;
#25282=CARTESIAN_POINT ( 'NONE',  ( 72.68867513459484542, 150.1262045565066785, -15.00000000000021316 ) ) ;
#25289=CARTESIAN_POINT ( 'NONE',  ( 66.08867513459483689, 142.2402378747194405, 9.270509831248432420 ) ) ;
#25291=DIRECTION ( 'NONE',  ( 0.000000000000000000, -0.7071067811865475727, -0.7071067811865475727 ) ) ;
#25295=ORIENTED_EDGE ( 'NONE', *, *, #19354, .F. ) ;
#25301=CARTESIAN_POINT ( 'NONE',  ( 72.87499999726881583, 138.6155565068815747, -3.929120461958505118E-15 ) ) ;
#25302=CARTESIAN_POINT ( 'NONE',  ( 80.62499999726880162, 138.6155565068815463, -3.929120461958505118E-15 ) ) ;
#25307=CARTESIAN_POINT ( 'NONE',  ( 42.40000000000000568, 150.2886644046228639, -14.50000000000000888 ) ) ;
#25313=CARTESIAN_POINT ( 'NONE',  ( 57.32499999726881157, 164.1591823560292198, -12.60653300113719766 ) ) ;
#25314=CARTESIAN_POINT ( 'NONE',  ( 64.27499999726880731, 160.0630714827496206, 15.58253174999999402 ) ) ;
#25321=DIRECTION ( 'NONE',  ( 1.000000000000000000, 0.000000000000000000, 0.000000000000000000 ) ) ;
#25323=CARTESIAN_POINT ( 'NONE',  ( 83.01132485994280330, 142.2402378747194405, 9.270509831248432420 ) ) ;
#25326=PLANE ( 'NONE',  #12382 ) ;
#25327=VERTEX_POINT ( 'NONE', #18223 ) ;
#25330=CARTESIAN_POINT ( 'NONE',  ( 75.87499999726881583, 171.3844434931184253, -7.942151717890132712E-15 ) ) ;
#25333=EDGE_CURVE ( 'NONE', #7786, #30423, #8703, .T. ) ;
#25334=CARTESIAN_POINT ( 'NONE',  ( 68.92499999726881299, 145.8408176439707802, -12.60653300113719588 ) ) ;
#25337=CARTESIAN_POINT ( 'NONE',  ( 59.42499999726882010, 168.2552932293087906, -9.630534252274385310 ) ) ;
#25340=ORIENTED_EDGE ( 'NONE', *, *, #31069, .F. ) ;
#25347=CARTESIAN_POINT ( 'NONE',  ( 45.28867513459482552, 170.7719333635740497, -7.904646289410545231E-15 ) ) ;
#25355=DIRECTION ( 'NONE',  ( -1.000000000000000000, -0.000000000000000000, -0.000000000000000000 ) ) ;
#25360=CARTESIAN_POINT ( 'NONE',  ( 85.48867513459482836, 167.7597621252805880, 9.270509831248428867 ) ) ;
#25363=CARTESIAN_POINT ( 'NONE',  ( 75.29999999453762882, 142.6655632788954620, 8.961492836873471646 ) ) ;
#25364=EDGE_LOOP ( 'NONE', ( #10808, #1248, #5344, #287 ) ) ;
#25367=ADVANCED_FACE ( 'NONE', ( #17713 ), #7336, .T. ) ;
#25369=AXIS2_PLACEMENT_3D ( 'NONE', #7394, #28347, #20161 ) ;
#25380=CARTESIAN_POINT ( 'NONE',  ( 54.81132485994282177, 150.1262045565065364, 15.00000000000011191 ) ) ;
#25382=CARTESIAN_POINT ( 'NONE',  ( 56.77499999726881441, 140.1801316387863778, 4.815267126137185549 ) ) ;
#25387=CARTESIAN_POINT ( 'NONE',  ( 68.37499999726881583, 155.0000000000000000, 15.58253174999999402 ) ) ;
#25394=CARTESIAN_POINT ( 'NONE',  ( 85.50000000000000000, 155.0000000000000000, 14.49999999999999467 ) ) ;
#25398=CARTESIAN_POINT ( 'NONE',  ( 52.47499999726881015, 149.9369285172503510, 15.58253174999999580 ) ) ;
#25402=CARTESIAN_POINT ( 'NONE',  ( 80.72499999726881015, 140.1801316387863778, -4.815267126137194431 ) ) ;
#25403=CARTESIAN_POINT ( 'NONE',  ( 52.71132485994279904, 155.0000000000000000, 15.00000000000001243 ) ) ;
#25405=CARTESIAN_POINT ( 'NONE',  ( 54.69999999453763451, 167.3344367211045096, 8.961492836873468093 ) ) ;
#25424=CARTESIAN_POINT ( 'NONE',  ( 35.17499999726881299, 145.8408176439707802, -12.60653300113719588 ) ) ;
#25426=CARTESIAN_POINT ( 'NONE',  ( 46.72499999726881015, 140.1801316387863778, -4.815267126137194431 ) ) ;
#25430=CARTESIAN_POINT ( 'NONE',  ( 45.67499999726881299, 168.2552932293087906, -9.630534252274385310 ) ) ;
#25435=CARTESIAN_POINT ( 'NONE',  ( 60.80000000000001137, 167.3344367211045096, -8.961492836873482304 ) ) ;
#25437=CARTESIAN_POINT ( 'NONE',  ( 125.5000000000000000, 155.0000000000000000, -6.938893903907228378E-15 ) ) ;
#25443=AXIS2_PLACEMENT_3D ( 'NONE', #21388, #26341, #21224 ) ;
#25444=CARTESIAN_POINT ( 'NONE',  ( 64.12499999726881583, 155.0000000000000000, 15.58253174999999402 ) ) ;
#25449=CARTESIAN_POINT ( 'NONE',  ( 34.49999999453763166, 170.2462022514548323, -7.872454543227099337E-15 ) ) ;
#25464=( BOUNDED_CURVE ( )  B_SPLINE_CURVE ( 2, ( #32258, #29540, #16758, #19144, #29887, #16921, #29205, #18988, #11820, #11156, #26975 ),
 .UNSPECIFIED., .F., .F. ) 
 B_SPLINE_CURVE_WITH_KNOTS ( ( 3, 2, 2, 2, 2, 3 ),
 ( 0.1785714285714282146, 0.1821428571428567733, 0.1857142857142854431, 0.1892857142857139741, 0.1928571428571425328, 0.1964285714285710915 ),
 .UNSPECIFIED. ) 
 CURVE ( )  GEOMETRIC_REPRESENTATION_ITEM ( )  RATIONAL_B_SPLINE_CURVE ( ( 1.000000000000003775, 0.9510565162951496454, 1.000000000000000000, 0.9510565162951534202, 1.000000000000000000, 0.9510565162951534202, 1.000000000000000000, 0.9510565162951534202, 1.000000000000000000, 0.9510565162951576390, 0.9999999999999957812 ) ) 
 REPRESENTATION_ITEM ( '' )  );
#25471=CARTESIAN_POINT ( 'NONE',  ( 82.12499999726881583, 155.0000000000000000, 15.58253174999999402 ) ) ;
#25472=DIRECTION ( 'NONE',  ( 1.000000000000000000, 0.000000000000000000, 0.000000000000000000 ) ) ;
#25477=CARTESIAN_POINT ( 'NONE',  ( 40.90000000000000568, 168.7903194862797420, -4.480746418436745593 ) ) ;
#25481=CARTESIAN_POINT ( 'NONE',  ( 54.52499999726881441, 140.1801316387863778, 4.815267126137185549 ) ) ;
#25482=CARTESIAN_POINT ( 'NONE',  ( 71.27499999726880731, 149.9369285172503510, -15.58253175000000823 ) ) ;
#25484=FACE_BOUND ( 'NONE', #13387, .T. ) ;
#25494=CARTESIAN_POINT ( 'NONE',  ( 32.50000000000000000, 155.0000000000000000, -15.00000000000002487 ) ) ;
#25502=CARTESIAN_POINT ( 'NONE',  ( 78.37499999726883004, 155.0000000000000000, 15.58253174999999402 ) ) ;
#25506=CARTESIAN_POINT ( 'NONE',  ( 70.02499999726879309, 160.0630714827496206, 15.58253174999999224 ) ) ;
#25510=CARTESIAN_POINT ( 'NONE',  ( 65.62499999726880162, 171.3844434931184253, -7.942151717890132712E-15 ) ) ;
#25527=CARTESIAN_POINT ( 'NONE',  ( 36.22499999726881015, 149.9369285172503510, 15.58253174999999580 ) ) ;
#25531=EDGE_CURVE ( 'NONE', #562, #7373, #11300, .T. ) ;
#25536=CARTESIAN_POINT ( 'NONE',  ( 72.59999999453762598, 168.7903194862797420, 4.480746418436729606 ) ) ;
#25537=VERTEX_POINT ( 'NONE', #24321 ) ;
#25556=CARTESIAN_POINT ( 'NONE',  ( 55.77499999726881441, 169.8198683612136222, -4.815267126137197984 ) ) ;
#25563=CARTESIAN_POINT ( 'NONE',  ( 67.47499999726879594, 160.0630714827496206, -15.58253175000000823 ) ) ;
#25567=DIRECTION ( 'NONE',  ( 0.000000000000000000, 0.000000000000000000, -1.000000000000000000 ) ) ;
#25569=CARTESIAN_POINT ( 'NONE',  ( 33.82499999726880446, 168.2552932293087906, 9.630534252274372875 ) ) ;
#25571=DIRECTION ( 'NONE',  ( 0.000000000000000000, 0.000000000000000000, -1.000000000000000000 ) ) ;
#25573=CARTESIAN_POINT ( 'NONE',  ( 86.71132485994282035, 155.0000000000000000, 15.00000000000001243 ) ) ;
#25574=CARTESIAN_POINT ( 'NONE',  ( 51.07499999726879736, 141.7447067706911810, -9.630534252274385310 ) ) ;
#25577=DIRECTION ( 'NONE',  ( 0.000000000000000000, 0.000000000000000000, -1.000000000000000000 ) ) ;
#25578=CARTESIAN_POINT ( 'NONE',  ( 52.31132485994280046, 169.2658477444273331, 4.635254915624208216 ) ) ;
#25580=CARTESIAN_POINT ( 'NONE',  ( 50.89999999453763735, 159.7113355953771077, 14.49999999999999289 ) ) ;
#25585=DIRECTION ( 'NONE',  ( -1.000000000000000000, 0.000000000000000000, -0.000000000000000000 ) ) ;
#25593=ORIENTED_EDGE ( 'NONE', *, *, #32425, .T. ) ;
#25595=EDGE_CURVE ( 'NONE', #12632, #11089, #28712, .T. ) ;
#25597=CARTESIAN_POINT ( 'NONE',  ( 36.47499999726881015, 149.9369285172503510, 15.58253174999999580 ) ) ;
#25599=CARTESIAN_POINT ( 'NONE',  ( 46.82499999726880446, 141.7447067706911810, -9.630534252274385310 ) ) ;
#25600=LINE ( 'NONE', #28501, #6636 ) ;
#25604=CARTESIAN_POINT ( 'NONE',  ( 44.57499999726881157, 145.8408176439707802, 12.60653300113718345 ) ) ;
#25608=CARTESIAN_POINT ( 'NONE',  ( 70.00000000000000000, 139.7537977485451393, -4.138211985947621020E-15 ) ) ;
#25614=CARTESIAN_POINT ( 'NONE',  ( 72.42499999726881299, 141.7447067706911810, 9.630534252274376428 ) ) ;
#25618=CARTESIAN_POINT ( 'NONE',  ( 88.37499999726880162, 155.0000000000000000, 15.58253174999999402 ) ) ;
#25621=VERTEX_POINT ( 'NONE', #17335 ) ;
#25638=CARTESIAN_POINT ( 'NONE',  ( 34.61132485994281183, 159.8737954434934636, 15.00000000000012967 ) ) ;
#25640=CARTESIAN_POINT ( 'NONE',  ( 80.91132485994280898, 146.1832212156128890, 12.13525491562421976 ) ) ;
#25642=CARTESIAN_POINT ( 'NONE',  ( 83.92499999726882720, 164.1591823560292198, 12.60653300113718167 ) ) ;
#25647=CARTESIAN_POINT ( 'NONE',  ( 47.39999999999999147, 159.7113355953771077, 14.49999999999999289 ) ) ;
#25649=CARTESIAN_POINT ( 'NONE',  ( 37.71132485994279904, 155.0000000000000000, -15.00000000000002487 ) ) ;
#25653=CARTESIAN_POINT ( 'NONE',  ( 54.62499999726880873, 138.6155565068815747, -3.929120461958505118E-15 ) ) ;
#25654=CARTESIAN_POINT ( 'NONE',  ( 71.77499999726882152, 169.8198683612136222, -4.815267126137197984 ) ) ;
#25656=DIRECTION ( 'NONE',  ( 1.000000000000000000, 0.000000000000000000, 0.000000000000000000 ) ) ;
#25667=DIRECTION ( 'NONE',  ( 1.000000000000000000, 0.000000000000000000, 0.000000000000000000 ) ) ;
#25668=EDGE_LOOP ( 'NONE', ( #6863, #22182, #6224, #8238 ) ) ;
#25670=AXIS2_PLACEMENT_3D ( 'NONE', #6505, #8393, #1059 ) ;
#25673=CARTESIAN_POINT ( 'NONE',  ( 77.57499999726881867, 164.1591823560292198, -12.60653300113719766 ) ) ;
#25676=CARTESIAN_POINT ( 'NONE',  ( 72.42499999726881299, 141.7447067706911810, 9.630534252274376428 ) ) ;
#25680=CARTESIAN_POINT ( 'NONE',  ( 66.42499999726879878, 141.7447067706911810, 9.630534252274376428 ) ) ;
#25681=DIRECTION ( 'NONE',  ( 1.000000000000000000, 0.000000000000000000, 0.000000000000000000 ) ) ;
#25688=DIRECTION ( 'NONE',  ( 0.000000000000000000, 0.000000000000000000, 1.000000000000000000 ) ) ;
#25694=CARTESIAN_POINT ( 'NONE',  ( 40.92499999726881299, 145.8408176439707802, -12.60653300113719588 ) ) ;
#25702=CARTESIAN_POINT ( 'NONE',  ( 74.89999999453760893, 159.7113355953771077, 14.49999999999999289 ) ) ;
#25716=CARTESIAN_POINT ( 'NONE',  ( 55.78867513459481842, 155.0000000000000000, 15.00000000000001243 ) ) ;
#25722=CARTESIAN_POINT ( 'NONE',  ( 54.37499999726881583, 155.0000000000000000, 15.58253174999999402 ) ) ;
#25726=PRESENTATION_STYLE_ASSIGNMENT (( #28292 ) ) ;
#25735=CARTESIAN_POINT ( 'NONE',  ( 33.22499999726881725, 160.0630714827496206, -15.58253175000000823 ) ) ;
#25739=CARTESIAN_POINT ( 'NONE',  ( 64.78867513459482552, 155.0000000000000000, -15.00000000000002487 ) ) ;
#25740=CARTESIAN_POINT ( 'NONE',  ( 47.77499999726881441, 169.8198683612136222, -4.815267126137197984 ) ) ;
#25742=DIRECTION ( 'NONE',  ( -1.000000000000000000, 0.000000000000000000, -0.000000000000000000 ) ) ;
#25745=CARTESIAN_POINT ( 'NONE',  ( 51.49999999453763166, 139.7537977485451393, -4.138211985947621020E-15 ) ) ;
#25746=ORIENTED_EDGE ( 'NONE', *, *, #27409, .T. ) ;
#25761=CARTESIAN_POINT ( 'NONE',  ( 76.07499999726880446, 168.2552932293087906, 9.630534252274372875 ) ) ;
#25766=CARTESIAN_POINT ( 'NONE',  ( 36.87499999726881583, 138.6155565068815747, -3.929120461958505118E-15 ) ) ;
#25768=CARTESIAN_POINT ( 'NONE',  ( 46.62499999726880873, 138.6155565068815463, -3.929120461958505118E-15 ) ) ;
#25771=VECTOR ( 'NONE', #14459, 1000.000000000000000 ) ;
#25774=CARTESIAN_POINT ( 'NONE',  ( 44.17499999726881299, 164.1591823560292198, 12.60653300113718167 ) ) ;
#25779=ADVANCED_FACE ( 'NONE', ( #6776 ), #27547, .T. ) ;
#25781=CARTESIAN_POINT ( 'NONE',  ( 70.09999999999999432, 141.2096805137202580, -4.480746418436742040 ) ) ;
#25782=( BOUNDED_CURVE ( )  B_SPLINE_CURVE ( 2, ( #29495, #11607, #5813, #3775, #11276, #21657, #21823, #16210, #32213, #32053, #8716 ),
 .UNSPECIFIED., .F., .T. ) 
 B_SPLINE_CURVE_WITH_KNOTS ( ( 3, 2, 2, 2, 2, 3 ),
 ( 0.2499999999999996947, 0.2535714285714282812, 0.2571428571428568399, 0.2607142857142853987, 0.2642857142857140129, 0.2678571428571425717 ),
 .UNSPECIFIED. ) 
 CURVE ( )  GEOMETRIC_REPRESENTATION_ITEM ( )  RATIONAL_B_SPLINE_CURVE ( ( 1.000000000000004219, 0.9510565162951492013, 1.000000000000000000, 0.9510565162951534202, 1.000000000000000000, 0.9510565162951534202, 1.000000000000000000, 0.9510565162951534202, 1.000000000000000000, 0.9510565162951564178, 0.9999999999999970024 ) ) 
 REPRESENTATION_ITEM ( '' )  );
#25791=CARTESIAN_POINT ( 'NONE',  ( 71.42499999726879878, 168.2552932293087906, -9.630534252274385310 ) ) ;
#25792=VERTEX_POINT ( 'NONE', #14771 ) ;
#25794=CARTESIAN_POINT ( 'NONE',  ( 86.97499999726882436, 140.1801316387863778, -4.815267126137194431 ) ) ;
#25796=ADVANCED_FACE ( 'NONE', ( #3712 ), #19555, .F. ) ;
#25805=EDGE_LOOP ( 'NONE', ( #19517, #14401, #11546, #9849 ) ) ;
#25815=CARTESIAN_POINT ( 'NONE',  ( 81.21132485994280614, 139.2280666364260071, -4.041636747397287284E-15 ) ) ;
#25817=CARTESIAN_POINT ( 'NONE',  ( 85.72499999726882436, 169.8198683612136222, 4.815267126137181997 ) ) ;
#25818=CARTESIAN_POINT ( 'NONE',  ( 51.71132485994281325, 155.0000000000000000, -15.00000000000002487 ) ) ;
#25821=CARTESIAN_POINT ( 'NONE',  ( 47.50000000000000000, 155.0000000000000000, 14.49999999999999467 ) ) ;
#25825=CARTESIAN_POINT ( 'NONE',  ( 48.32499999726881157, 145.8408176439707802, 12.60653300113718345 ) ) ;
#25828=CARTESIAN_POINT ( 'NONE',  ( 59.52499999726881441, 169.8198683612136222, -4.815267126137197984 ) ) ;
#25829=CARTESIAN_POINT ( 'NONE',  ( 69.77499999726880731, 169.8198683612136222, -4.815267126137197984 ) ) ;
#25840=CARTESIAN_POINT ( 'NONE',  ( 68.21132485994280614, 170.7719333635740497, -7.904646289410545231E-15 ) ) ;
#25842=EDGE_CURVE ( 'NONE', #18876, #30423, #15113, .T. ) ;
#25848=CARTESIAN_POINT ( 'NONE',  ( 75.47499999726881015, 160.0630714827496206, -15.58253175000000823 ) ) ;
#25851=CARTESIAN_POINT ( 'NONE',  ( 74.42499999726881299, 141.7447067706911810, 9.630534252274376428 ) ) ;
#25854=CARTESIAN_POINT ( 'NONE',  ( 64.52499999726882152, 140.1801316387863778, 4.815267126137185549 ) ) ;
#25869=CARTESIAN_POINT ( 'NONE',  ( 35.22499999726881015, 160.0630714827496206, -15.58253175000000823 ) ) ;
#25878=CARTESIAN_POINT ( 'NONE',  ( 76.09999999453762598, 159.7113355953771077, -14.50000000000000888 ) ) ;
#25882=CARTESIAN_POINT ( 'NONE',  ( 125.5000000000000000, 157.1500000000010573, 105.9999999999999858 ) ) ;
#25893=CARTESIAN_POINT ( 'NONE',  ( 60.67499999726881299, 141.7447067706911810, 9.630534252274376428 ) ) ;
#25894=ORIENTED_EDGE ( 'NONE', *, *, #26852, .T. ) ;
#25899=LINE ( 'NONE', #15837, #7840 ) ;
#25904=CARTESIAN_POINT ( 'NONE',  ( 34.82499999726881157, 141.7447067706911810, -9.630534252274385310 ) ) ;
#25908=CARTESIAN_POINT ( 'NONE',  ( 48.17499999726881299, 164.1591823560292198, 12.60653300113718167 ) ) ;
#25911=CARTESIAN_POINT ( 'NONE',  ( 35.61132485994281183, 150.1262045565064511, -15.00000000000005329 ) ) ;
#25913=CARTESIAN_POINT ( 'NONE',  ( 65.51132485994280330, 146.1832212156128890, -12.13525491562423042 ) ) ;
#25914=CARTESIAN_POINT ( 'NONE',  ( 55.59999999453763309, 141.2096805137202580, -4.480746418436742040 ) ) ;
#25920=CARTESIAN_POINT ( 'NONE',  ( 59.71132485994280614, 155.0000000000000000, -15.00000000000002487 ) ) ;
#25926=CARTESIAN_POINT ( 'NONE',  ( 80.68867513459484542, 150.1262045565065648, -15.00000000000015632 ) ) ;
#25927=ORIENTED_EDGE ( 'NONE', *, *, #5641, .F. ) ;
#25931=CARTESIAN_POINT ( 'NONE',  ( 42.67499999726880588, 141.7447067706911810, 9.630534252274376428 ) ) ;
#25933=CARTESIAN_POINT ( 'NONE',  ( 52.22499999726881725, 149.9369285172503510, 15.58253174999999580 ) ) ;
#25934=DIRECTION ( 'NONE',  ( -1.000000000000000000, -0.000000000000000000, -0.000000000000000000 ) ) ;
#25937=CARTESIAN_POINT ( 'NONE',  ( 45.97499999726881015, 169.8198683612136222, 4.815267126137181997 ) ) ;
#25942=CARTESIAN_POINT ( 'NONE',  ( 70.50000000000000000, 155.0000000000000000, -14.50000000000000711 ) ) ;
#25946=CARTESIAN_POINT ( 'NONE',  ( 85.98867513459482836, 146.1832212156128890, 12.13525491562421976 ) ) ;
#25950=CARTESIAN_POINT ( 'NONE',  ( 68.02499999726882152, 160.0630714827496206, 15.58253174999999402 ) ) ;
#25953=CARTESIAN_POINT ( 'NONE',  ( 37.79999999453762882, 146.4771138417591203, -11.73074641843674470 ) ) ;
#25975=CARTESIAN_POINT ( 'NONE',  ( 89.50000000000001421, 155.0000000000000000, -6.938893903907228378E-15 ) ) ;
#25976=( BOUNDED_CURVE ( )  B_SPLINE_CURVE ( 2, ( #18397, #11, #28111, #23002, #7847, #30849, #6269, #13772, #24000, #29114, #8664 ),
 .UNSPECIFIED., .F., .T. ) 
 B_SPLINE_CURVE_WITH_KNOTS ( ( 3, 2, 2, 2, 2, 3 ),
 ( 0.3392857142857140795, 0.3428571428571427493, 0.3464285714285713080, 0.3499999999999998113, 0.3535714285714283700, 0.3571428571428569287 ),
 .UNSPECIFIED. ) 
 CURVE ( )  GEOMETRIC_REPRESENTATION_ITEM ( )  RATIONAL_B_SPLINE_CURVE ( ( 1.000000000000001554, 0.9510565162951518658, 1.000000000000000000, 0.9510565162951534202, 1.000000000000000000, 0.9510565162951534202, 1.000000000000000000, 0.9510565162951534202, 1.000000000000000000, 0.9510565162951557516, 0.9999999999999976685 ) ) 
 REPRESENTATION_ITEM ( '' )  );
#25978=CARTESIAN_POINT ( 'NONE',  ( 84.32499999726880446, 145.8408176439707802, 12.60653300113718345 ) ) ;
#25982=CARTESIAN_POINT ( 'NONE',  ( 125.5000000000000000, 48.99999999999998579, -1.387778780781445676E-14 ) ) ;
#25986=CARTESIAN_POINT ( 'NONE',  ( 51.39999999999999858, 159.7113355953771077, 14.49999999999999289 ) ) ;
#25991=CARTESIAN_POINT ( 'NONE',  ( 52.92499999726881299, 145.8408176439707802, -12.60653300113719588 ) ) ;
#25994=CARTESIAN_POINT ( 'NONE',  ( 55.02499999726881441, 149.9369285172503510, -15.58253175000000823 ) ) ;
#25995=CARTESIAN_POINT ( 'NONE',  ( 68.47499999726878173, 149.9369285172503510, 15.58253174999999580 ) ) ;
#26013=ORIENTED_EDGE ( 'NONE', *, *, #27227, .T. ) ;
#26014=FACE_OUTER_BOUND ( 'NONE', #14809, .T. ) ;
#26019=CARTESIAN_POINT ( 'NONE',  ( 72.92499999726881299, 145.8408176439707802, -12.60653300113719588 ) ) ;
#26022=CARTESIAN_POINT ( 'NONE',  ( 61.62499999726881583, 171.3844434931184253, -7.942151717890132712E-15 ) ) ;
#26031=EDGE_CURVE ( 'NONE', #11207, #7326, #27676, .T. ) ;
#26038=CARTESIAN_POINT ( 'NONE',  ( 127.5000000000000000, 155.0000000000000000, 112.0000000000000711 ) ) ;
#26040=CARTESIAN_POINT ( 'NONE',  ( 36.42499999726879878, 141.7447067706911810, 9.630534252274376428 ) ) ;
#26048=CARTESIAN_POINT ( 'NONE',  ( 77.29999999453764303, 142.6655632788954620, 8.961492836873471646 ) ) ;
#26053=VERTEX_POINT ( 'NONE', #616 ) ;
#26068=CARTESIAN_POINT ( 'NONE',  ( 61.97499999726881015, 169.8198683612136222, 4.815267126137181997 ) ) ;
#26069=CIRCLE ( 'NONE', #29317, 15.00000000000001776 ) ;
#26070=ORIENTED_EDGE ( 'NONE', *, *, #24941, .T. ) ;
#26080=CARTESIAN_POINT ( 'NONE',  ( 84.70000000000000284, 163.5228861582408797, -11.73074641843674470 ) ) ;
#26086=CARTESIAN_POINT ( 'NONE',  ( 58.37499999726881583, 155.0000000000000000, 15.58253174999999402 ) ) ;
#26090=CARTESIAN_POINT ( 'NONE',  ( 32.50000000000000000, 155.0000000000000000, -6.938893903907228378E-15 ) ) ;
#26091=CARTESIAN_POINT ( 'NONE',  ( 59.69999999453762030, 142.6655632788954620, -8.961492836873480528 ) ) ;
#26098=ORIENTED_EDGE ( 'NONE', *, *, #11870, .T. ) ;
#26107=CARTESIAN_POINT ( 'NONE',  ( 43.77499999726881441, 169.8198683612136222, -4.815267126137197984 ) ) ;
#26109=CARTESIAN_POINT ( 'NONE',  ( 48.22499999726880304, 149.9369285172503510, 15.58253174999999580 ) ) ;
#26113=CARTESIAN_POINT ( 'NONE',  ( 53.67499999726879878, 168.2552932293087906, -9.630534252274385310 ) ) ;
#26114=CARTESIAN_POINT ( 'NONE',  ( 79.41132485994285162, 142.2402378747194405, -9.270509831248439525 ) ) ;
#26116=CARTESIAN_POINT ( 'NONE',  ( 44.08867513459483689, 142.2402378747194405, 9.270509831248432420 ) ) ;
#26117=CARTESIAN_POINT ( 'NONE',  ( 65.70000000000000284, 146.4771138417591203, 11.73074641843673227 ) ) ;
#26122=CARTESIAN_POINT ( 'NONE',  ( 38.97499999726881015, 140.1801316387863778, -4.815267126137194431 ) ) ;
#26124=CARTESIAN_POINT ( 'NONE',  ( 71.22499999726879594, 160.0630714827496206, -15.58253175000000823 ) ) ;
#26125=ORIENTED_EDGE ( 'NONE', *, *, #11256, .F. ) ;
#26126=CARTESIAN_POINT ( 'NONE',  ( 43.51132485994280330, 146.1832212156128890, -12.13525491562423042 ) ) ;
#26127=CARTESIAN_POINT ( 'NONE',  ( 36.09999999453761887, 159.7113355953771077, -14.50000000000000888 ) ) ;
#26129=( BOUNDED_CURVE ( )  B_SPLINE_CURVE ( 2, ( #8040, #19085, #533, #28817, #21302, #359, #21636, #15861, #8206, #11093, #31696 ),
 .UNSPECIFIED., .F., .F. ) 
 B_SPLINE_CURVE_WITH_KNOTS ( ( 3, 2, 2, 2, 2, 3 ),
 ( 0.2857142857142854209, 0.2892857142857139796, 0.2928571428571425939, 0.2964285714285711526, 0.2999999999999997669, 0.3035714285714283256 ),
 .UNSPECIFIED. ) 
 CURVE ( )  GEOMETRIC_REPRESENTATION_ITEM ( )  RATIONAL_B_SPLINE_CURVE ( ( 1.000000000000003775, 0.9510565162951496454, 1.000000000000000000, 0.9510565162951534202, 1.000000000000000000, 0.9510565162951534202, 1.000000000000000000, 0.9510565162951534202, 1.000000000000000000, 0.9510565162951557516, 0.9999999999999976685 ) ) 
 REPRESENTATION_ITEM ( '' )  );
#26138=CARTESIAN_POINT ( 'NONE',  ( 74.31132485994281467, 169.2658477444273331, 4.635254915624208216 ) ) ;
#26139=ORIENTED_EDGE ( 'NONE', *, *, #12320, .T. ) ;
#26145=CARTESIAN_POINT ( 'NONE',  ( 37.47499999726880304, 160.0630714827496206, -15.58253175000000823 ) ) ;
#26146=CARTESIAN_POINT ( 'NONE',  ( 125.5000000000000000, 48.99999999999998579, -1.387778780781445676E-14 ) ) ;
#26150=CARTESIAN_POINT ( 'NONE',  ( 47.60000000000000853, 150.2886644046228639, 14.49999999999999645 ) ) ;
#26154=CARTESIAN_POINT ( 'NONE',  ( 48.42499999726881299, 141.7447067706911810, 9.630534252274376428 ) ) ;
#26157=CARTESIAN_POINT ( 'NONE',  ( 65.02499999726882152, 149.9369285172503510, -15.58253175000000823 ) ) ;
#26158=CARTESIAN_POINT ( 'NONE',  ( 69.67499999726878457, 168.2552932293087906, -9.630534252274385310 ) ) ;
#26165=CARTESIAN_POINT ( 'NONE',  ( 68.61132485994279762, 159.8737954434937478, 14.99999999999991651 ) ) ;
#26171=EDGE_LOOP ( 'NONE', ( #31249, #20949, #17966, #4421 ) ) ;
#26175=CARTESIAN_POINT ( 'NONE',  ( 77.92499999726881299, 164.1591823560292198, 12.60653300113718167 ) ) ;
#26178=CIRCLE ( 'NONE', #11493, 2.149999999999974598 ) ;
#26179=CARTESIAN_POINT ( 'NONE',  ( 63.22499999726881725, 160.0630714827496206, -15.58253175000000823 ) ) ;
#26181=LINE ( 'NONE', #26352, #2057 ) ;
#26182=ADVANCED_FACE ( 'NONE', ( #24120 ), #21397, .T. ) ;
#26188=FACE_BOUND ( 'NONE', #17715, .T. ) ;
#26196=CARTESIAN_POINT ( 'NONE',  ( 35.12499999726881583, 155.0000000000000000, -15.58253175000000823 ) ) ;
#26204=CARTESIAN_POINT ( 'NONE',  ( 76.69999999453764872, 167.3344367211045096, 8.961492836873468093 ) ) ;
#26210=ORIENTED_EDGE ( 'NONE', *, *, #3735, .F. ) ;
#26213=ORIENTED_EDGE ( 'NONE', *, *, #11870, .F. ) ;
#26216=CARTESIAN_POINT ( 'NONE',  ( 56.58867513459482979, 146.1832212156128890, -12.13525491562423042 ) ) ;
#26220=CARTESIAN_POINT ( 'NONE',  ( 62.07499999726881157, 168.2552932293087906, 9.630534252274372875 ) ) ;
#26221=ORIENTED_EDGE ( 'NONE', *, *, #6663, .T. ) ;
#26232=CARTESIAN_POINT ( 'NONE',  ( 39.32499999726881157, 164.1591823560292198, -12.60653300113719766 ) ) ;
#26237=CARTESIAN_POINT ( 'NONE',  ( 54.17499999726881299, 164.1591823560292198, 12.60653300113718167 ) ) ;
#26242=CARTESIAN_POINT ( 'NONE',  ( 35.21132485994281325, 139.2280666364260071, -4.041636747397287284E-15 ) ) ;
#26243=CARTESIAN_POINT ( 'NONE',  ( 55.58867513459482268, 163.8167787843871110, 12.13525491562421621 ) ) ;
#26245=CARTESIAN_POINT ( 'NONE',  ( 60.79999999453762882, 163.5228861582408797, 11.73074641843673049 ) ) ;
#26249=ADVANCED_FACE ( 'NONE', ( #31624 ), #8291, .T. ) ;
#26250=CARTESIAN_POINT ( 'NONE',  ( 77.61132485994281183, 150.1262045565064227, -15.00000000000002665 ) ) ;
#26252=CARTESIAN_POINT ( 'NONE',  ( 59.41132485994281609, 142.2402378747194405, -9.270509831248439525 ) ) ;
#26262=VECTOR ( 'NONE', #33120, 1000.000000000000000 ) ;
#26266=CARTESIAN_POINT ( 'NONE',  ( 45.17499999726881299, 145.8408176439707802, -12.60653300113719588 ) ) ;
#26267=ORIENTED_EDGE ( 'NONE', *, *, #12476, .F. ) ;
#26268=CARTESIAN_POINT ( 'NONE',  ( 49.72499999726881725, 169.8198683612136222, 4.815267126137181997 ) ) ;
#26272=CARTESIAN_POINT ( 'NONE',  ( 50.57499999726881157, 145.8408176439707802, 12.60653300113718345 ) ) ;
#26273=CARTESIAN_POINT ( 'NONE',  ( 52.28867513459482552, 139.2280666364260071, -4.041636747397287284E-15 ) ) ;
#26275=CARTESIAN_POINT ( 'NONE',  ( 125.5000000000000000, 78.52640161467446944, -73.43303922622258995 ) ) ;
#26277=CARTESIAN_POINT ( 'NONE',  ( 68.50000000000000000, 155.0000000000000000, -14.50000000000000711 ) ) ;
#26281=CARTESIAN_POINT ( 'NONE',  ( 40.07499999726879736, 168.2552932293087906, 9.630534252274372875 ) ) ;
#26283=CARTESIAN_POINT ( 'NONE',  ( 68.52499999726880731, 140.1801316387863778, 4.815267126137185549 ) ) ;
#26284=ORIENTED_EDGE ( 'NONE', *, *, #3748, .F. ) ;
#26287=CARTESIAN_POINT ( 'NONE',  ( 43.69999999453763451, 142.6655632788954620, -8.961492836873480528 ) ) ;
#26307=CARTESIAN_POINT ( 'NONE',  ( 33.42499999726881299, 168.2552932293087906, -9.630534252274385310 ) ) ;
#26309=VECTOR ( 'NONE', #2432, 1000.000000000000000 ) ;
#26310=CARTESIAN_POINT ( 'NONE',  ( 86.02499999726880731, 160.0630714827496206, 15.58253174999999402 ) ) ;
#26315=CARTESIAN_POINT ( 'NONE',  ( 45.99999999999999289, 139.7537977485451393, -4.138211985947621020E-15 ) ) ;
#26318=( BOUNDED_CURVE ( )  B_SPLINE_CURVE ( 2, ( #20606, #17536, #12591, #10058, #5096, #27923, #4597, #17880, #5260, #14982, #7664 ),
 .UNSPECIFIED., .F., .T. ) 
 B_SPLINE_CURVE_WITH_KNOTS ( ( 3, 2, 2, 2, 2, 3 ),
 ( 0.7321428571428570953, 0.7357142857142857650, 0.7392857142857143238, 0.7428571428571428825, 0.7464285714285714413, 0.7500000000000000000 ),
 .UNSPECIFIED. ) 
 CURVE ( )  GEOMETRIC_REPRESENTATION_ITEM ( )  RATIONAL_B_SPLINE_CURVE ( ( 1.000000000000000000, 0.9510565162951534202, 1.000000000000000000, 0.9510565162951534202, 1.000000000000000000, 0.9510565162951534202, 1.000000000000000000, 0.9510565162951534202, 1.000000000000000000, 0.9510565162951534202, 1.000000000000000000 ) ) 
 REPRESENTATION_ITEM ( '' )  );
#26319=CARTESIAN_POINT ( 'NONE',  ( 49.02499999726880731, 149.9369285172503510, -15.58253175000000823 ) ) ;
#26323=CARTESIAN_POINT ( 'NONE',  ( 62.62499999726880873, 138.6155565068815747, -3.929120461958505118E-15 ) ) ;
#26324=CARTESIAN_POINT ( 'NONE',  ( 79.37499999726881583, 155.0000000000000000, -15.58253175000000823 ) ) ;
#26333=CARTESIAN_POINT ( 'NONE',  ( 34.78867513459482552, 155.0000000000000000, -15.00000000000002487 ) ) ;
#26337=EDGE_CURVE ( 'NONE', #28846, #27342, #26505, .T. ) ;
#26338=EDGE_LOOP ( 'NONE', ( #29192, #2505 ) ) ;
#26341=DIRECTION ( 'NONE',  ( 1.000000000000000000, 0.000000000000000000, 0.000000000000000000 ) ) ;
#26345=CARTESIAN_POINT ( 'NONE',  ( 78.52499999726880731, 140.1801316387863778, 4.815267126137185549 ) ) ;
#26347=STYLED_ITEM ( 'NONE', ( #25726 ), #32336 ) ;
#26350=CARTESIAN_POINT ( 'NONE',  ( 67.62499999726881583, 171.3844434931184253, -7.942151717890132712E-15 ) ) ;
#26352=CARTESIAN_POINT ( 'NONE',  ( 32.50000000000000000, 155.0000000000000000, 15.00000000000001243 ) ) ;
#26363=CARTESIAN_POINT ( 'NONE',  ( 87.50000000000001421, 160.9457742543943652, -14.40357817542362540 ) ) ;
#26364=CARTESIAN_POINT ( 'NONE',  ( 60.78867513459481842, 155.0000000000000000, -15.00000000000002487 ) ) ;
#26365=CARTESIAN_POINT ( 'NONE',  ( 46.82499999726881157, 141.7447067706911810, -9.630534252274387086 ) ) ;
#26367=DIRECTION ( 'NONE',  ( 1.000000000000000000, 0.000000000000000000, 0.000000000000000000 ) ) ;
#26372=CARTESIAN_POINT ( 'NONE',  ( 78.49999999453764588, 170.2462022514548323, -7.872454543227099337E-15 ) ) ;
#26380=EDGE_CURVE ( 'NONE', #26053, #29866, #1947, .T. ) ;
#26381=ORIENTED_EDGE ( 'NONE', *, *, #12703, .F. ) ;
#26382=CARTESIAN_POINT ( 'NONE',  ( 74.67499999726879878, 141.7447067706911810, 9.630534252274376428 ) ) ;
#26385=CARTESIAN_POINT ( 'NONE',  ( 58.98867513459482836, 163.8167787843871110, -12.13525491562423397 ) ) ;
#26389=CARTESIAN_POINT ( 'NONE',  ( 65.67499999726881299, 168.2552932293087906, -9.630534252274387086 ) ) ;
#26390=EDGE_LOOP ( 'NONE', ( #27977, #5432, #2044, #28658 ) ) ;
#26391=CARTESIAN_POINT ( 'NONE',  ( 36.51132485994280330, 163.8167787843871110, 12.13525491562421621 ) ) ;
#26399=CARTESIAN_POINT ( 'NONE',  ( 86.77499999726882152, 140.1801316387863778, 4.815267126137185549 ) ) ;
#26401=CARTESIAN_POINT ( 'NONE',  ( 37.32499999726881157, 164.1591823560292198, -12.60653300113719766 ) ) ;
#26405=CARTESIAN_POINT ( 'NONE',  ( 82.48867513459482836, 142.2402378747194405, -9.270509831248439525 ) ) ;
#26406=CARTESIAN_POINT ( 'NONE',  ( 54.27499999726880020, 160.0630714827496206, 15.58253174999999402 ) ) ;
#26411=CARTESIAN_POINT ( 'NONE',  ( 55.68867513459483831, 159.8737954434936057, 15.00000000000001421 ) ) ;
#26413=CARTESIAN_POINT ( 'NONE',  ( 58.19999999453763451, 163.5228861582408797, -11.73074641843674470 ) ) ;
#26421=ORIENTED_EDGE ( 'NONE', *, *, #23088, .T. ) ;
#26422=CARTESIAN_POINT ( 'NONE',  ( 87.50000000000004263, 168.9939550398769086, -6.930048056949515534 ) ) ;
#26423=LINE ( 'NONE', #18433, #26309 ) ;
#26428=CARTESIAN_POINT ( 'NONE',  ( 46.47499999726880304, 149.9369285172503510, 15.58253174999999580 ) ) ;
#26430=CARTESIAN_POINT ( 'NONE',  ( 50.22499999726880304, 149.9369285172503510, 15.58253174999999580 ) ) ;
#26431=DIRECTION ( 'NONE',  ( 1.000000000000000000, 0.000000000000000000, 0.000000000000000000 ) ) ;
#26434=CARTESIAN_POINT ( 'NONE',  ( 52.57499999726881157, 145.8408176439707802, 12.60653300113718345 ) ) ;
#26436=CARTESIAN_POINT ( 'NONE',  ( 32.50000000000000000, 155.0000000000000000, -6.938893903907228378E-15 ) ) ;
#26438=CARTESIAN_POINT ( 'NONE',  ( 74.89999999999999147, 168.7903194862797420, -4.480746418436745593 ) ) ;
#26442=CARTESIAN_POINT ( 'NONE',  ( 56.78867513459481842, 155.0000000000000000, -15.00000000000002487 ) ) ;
#26443=CARTESIAN_POINT ( 'NONE',  ( 37.57499999726881157, 164.1591823560292198, -12.60653300113719766 ) ) ;
#26446=CARTESIAN_POINT ( 'NONE',  ( 79.72499999726881015, 169.8198683612136222, 4.815267126137181997 ) ) ;
#26449=CARTESIAN_POINT ( 'NONE',  ( 42.39999999453762314, 168.7903194862797420, -4.480746418436745593 ) ) ;
#26462=EDGE_LOOP ( 'NONE', ( #12504, #27926, #14694, #33476 ) ) ;
#26464=EDGE_CURVE ( 'NONE', #14208, #5796, #22399, .T. ) ;
#26470=CARTESIAN_POINT ( 'NONE',  ( 35.27499999726881441, 149.9369285172503510, -15.58253175000000823 ) ) ;
#26474=CARTESIAN_POINT ( 'NONE',  ( 57.70000000000000284, 146.4771138417591203, 11.73074641843673227 ) ) ;
#26478=CARTESIAN_POINT ( 'NONE',  ( 49.42499999726879878, 168.2552932293087906, -9.630534252274385310 ) ) ;
#26480=ORIENTED_EDGE ( 'NONE', *, *, #7424, .T. ) ;
#26482=CARTESIAN_POINT ( 'NONE',  ( 64.22499999726881015, 149.9369285172503510, 15.58253174999999580 ) ) ;
#26483=CARTESIAN_POINT ( 'NONE',  ( 75.27499999726879309, 149.9369285172503510, -15.58253175000000823 ) ) ;
#26485=DIRECTION ( 'NONE',  ( 0.000000000000000000, 0.000000000000000000, -1.000000000000000000 ) ) ;
#26487=CARTESIAN_POINT ( 'NONE',  ( 84.18867513459483121, 140.7341522555726669, 4.635254915624211769 ) ) ;
#26501=AXIS2_PLACEMENT_3D ( 'NONE', #22497, #9543, #7000 ) ;
#26504=CARTESIAN_POINT ( 'NONE',  ( 77.72499999726881015, 169.8198683612136222, 4.815267126137181997 ) ) ;
#26505=LINE ( 'NONE', #3174, #13002 ) ;
#26507=CARTESIAN_POINT ( 'NONE',  ( 68.42499999726881299, 141.7447067706911810, 9.630534252274376428 ) ) ;
#26511=CARTESIAN_POINT ( 'NONE',  ( 38.50000000000000000, 155.0000000000000000, -14.50000000000000711 ) ) ;
#26514=DIRECTION ( 'NONE',  ( 0.000000000000000000, 0.000000000000000000, -1.000000000000000000 ) ) ;
#26515=EDGE_CURVE ( 'NONE', #3092, #5650, #29603, .T. ) ;
#26520=CARTESIAN_POINT ( 'NONE',  ( 42.72499999726881015, 140.1801316387863778, -4.815267126137194431 ) ) ;
#26529=CARTESIAN_POINT ( 'NONE',  ( 80.49999999453763166, 170.2462022514548323, -7.872454543227099337E-15 ) ) ;
#26538=ORIENTED_EDGE ( 'NONE', *, *, #11249, .F. ) ;
#26539=CARTESIAN_POINT ( 'NONE',  ( 74.57499999726881867, 145.8408176439707802, 12.60653300113718345 ) ) ;
#26541=CARTESIAN_POINT ( 'NONE',  ( 59.28867513459483263, 170.7719333635740497, -7.904646289410545231E-15 ) ) ;
#26543=AXIS2_PLACEMENT_3D ( 'NONE', #18803, #29195, #5847 ) ;
#26545=CARTESIAN_POINT ( 'NONE',  ( 59.87499999726881583, 171.3844434931184253, -7.942151717890134290E-15 ) ) ;
#26547=CARTESIAN_POINT ( 'NONE',  ( 36.61132485994281893, 159.8737954434935489, 15.00000000000005151 ) ) ;
#26554=CARTESIAN_POINT ( 'NONE',  ( 87.47499999726883857, 160.0630714827496206, -15.58253175000000823 ) ) ;
#26557=CARTESIAN_POINT ( 'NONE',  ( 40.52499999726881441, 140.1801316387863778, 4.815267126137185549 ) ) ;
#26562=CARTESIAN_POINT ( 'NONE',  ( 59.17499999726881299, 145.8408176439707802, -12.60653300113719588 ) ) ;
#26569=CARTESIAN_POINT ( 'NONE',  ( 59.49999999453761745, 139.7537977485451393, -4.138211985947621020E-15 ) ) ;
#26573=DIRECTION ( 'NONE',  ( 0.000000000000000000, 0.000000000000000000, -1.000000000000000000 ) ) ;
#26576=CARTESIAN_POINT ( 'NONE',  ( 71.91132485994280898, 163.8167787843871110, -12.13525491562423397 ) ) ;
#26583=CARTESIAN_POINT ( 'NONE',  ( 50.11132485994281183, 169.2658477444273331, -4.635254915624224203 ) ) ;
#26584=ORIENTED_EDGE ( 'NONE', *, *, #9825, .T. ) ;
#26589=CARTESIAN_POINT ( 'NONE',  ( 43.27499999726880731, 149.9369285172503510, -15.58253175000000823 ) ) ;
#26591=CARTESIAN_POINT ( 'NONE',  ( 50.92499999726880588, 145.8408176439707802, -12.60653300113719588 ) ) ;
#26597=CARTESIAN_POINT ( 'NONE',  ( 51.27499999726880731, 149.9369285172503510, -15.58253175000000823 ) ) ;
#26603=CARTESIAN_POINT ( 'NONE',  ( 72.09999999999999432, 141.2096805137202580, -4.480746418436742040 ) ) ;
#26605=DIRECTION ( 'NONE',  ( 1.000000000000000000, 0.000000000000000000, 0.000000000000000000 ) ) ;
#26608=CARTESIAN_POINT ( 'NONE',  ( 36.37499999726881583, 155.0000000000000000, 15.58253174999999402 ) ) ;
#26610=CARTESIAN_POINT ( 'NONE',  ( 76.92499999726881299, 145.8408176439707802, -12.60653300113719588 ) ) ;
#26612=ORIENTED_EDGE ( 'NONE', *, *, #10960, .F. ) ;
#26614=CARTESIAN_POINT ( 'NONE',  ( 38.09999999453761887, 159.7113355953771077, -14.50000000000000888 ) ) ;
#26624=ORIENTED_EDGE ( 'NONE', *, *, #19475, .F. ) ;
#26636=CARTESIAN_POINT ( 'NONE',  ( 36.17499999726880588, 164.1591823560292198, 12.60653300113718167 ) ) ;
#26640=CARTESIAN_POINT ( 'NONE',  ( 55.40000000000000568, 159.7113355953771077, 14.49999999999999289 ) ) ;
#26643=CARTESIAN_POINT ( 'NONE',  ( 58.22499999726881015, 149.9369285172503510, 15.58253174999999580 ) ) ;
#26646=CARTESIAN_POINT ( 'NONE',  ( 65.22499999726881015, 160.0630714827496206, -15.58253175000000823 ) ) ;
#26647=CARTESIAN_POINT ( 'NONE',  ( 76.57499999726881867, 145.8408176439707802, 12.60653300113718345 ) ) ;
#26661=EDGE_CURVE ( 'NONE', #16104, #11212, #7631, .T. ) ;
#26671=CARTESIAN_POINT ( 'NONE',  ( 79.22499999726879594, 160.0630714827496206, -15.58253175000000823 ) ) ;
#26675=CARTESIAN_POINT ( 'NONE',  ( 72.52499999726882152, 140.1801316387863778, 4.815267126137185549 ) ) ;
#26680=CARTESIAN_POINT ( 'NONE',  ( 37.00000000000000000, 170.2462022514548323, -7.872454543227099337E-15 ) ) ;
#26689=CARTESIAN_POINT ( 'NONE',  ( 42.82499999726880446, 141.7447067706911810, -9.630534252274387086 ) ) ;
#26696=CARTESIAN_POINT ( 'NONE',  ( 81.89999999453763735, 150.2886644046228639, -14.50000000000000888 ) ) ;
#26704=CIRCLE ( 'NONE', #12019, 2.149999999999994138 ) ;
#26708=CARTESIAN_POINT ( 'NONE',  ( 75.37499999726881583, 155.0000000000000000, -15.58253175000000823 ) ) ;
#26710=CARTESIAN_POINT ( 'NONE',  ( 59.48867513459483547, 167.7597621252805880, 9.270509831248428867 ) ) ;
#26714=CARTESIAN_POINT ( 'NONE',  ( 72.57499999726880446, 145.8408176439707802, 12.60653300113718345 ) ) ;
#26716=CARTESIAN_POINT ( 'NONE',  ( 62.78867513459482552, 155.0000000000000000, -15.00000000000002487 ) ) ;
#26723=CARTESIAN_POINT ( 'NONE',  ( 84.17499999726882720, 164.1591823560292198, 12.60653300113718167 ) ) ;
#26726=VECTOR ( 'NONE', #22886, 1000.000000000000000 ) ;
#26728=CARTESIAN_POINT ( 'NONE',  ( 38.22499999726881015, 149.9369285172503510, 15.58253174999999580 ) ) ;
#26729=CARTESIAN_POINT ( 'NONE',  ( 36.08867513459483689, 142.2402378747194405, 9.270509831248432420 ) ) ;
#26733=CARTESIAN_POINT ( 'NONE',  ( 56.07499999726881157, 168.2552932293087906, 9.630534252274372875 ) ) ;
#26739=CARTESIAN_POINT ( 'NONE',  ( 60.49999999453763166, 170.2462022514548323, -7.872454543227099337E-15 ) ) ;
#26740=ORIENTED_EDGE ( 'NONE', *, *, #11608, .T. ) ;
#26744=CARTESIAN_POINT ( 'NONE',  ( 72.41132485994282320, 167.7597621252805880, 9.270509831248428867 ) ) ;
#26749=CARTESIAN_POINT ( 'NONE',  ( 83.78867513459482552, 155.0000000000000000, 15.00000000000001243 ) ) ;
#26750=CARTESIAN_POINT ( 'NONE',  ( 66.71132485994280614, 155.0000000000000000, 15.00000000000001243 ) ) ;
#26751=ORIENTED_EDGE ( 'NONE', *, *, #29729, .T. ) ;
#26755=CARTESIAN_POINT ( 'NONE',  ( 51.07499999726880446, 141.7447067706911810, -9.630534252274387086 ) ) ;
#26757=CARTESIAN_POINT ( 'NONE',  ( 56.72499999726881015, 140.1801316387863778, -4.815267126137194431 ) ) ;
#26761=CARTESIAN_POINT ( 'NONE',  ( 32.50000000000000000, 155.0000000000000000, -6.938893903907228378E-15 ) ) ;
#26763=CARTESIAN_POINT ( 'NONE',  ( 56.17499999726881299, 164.1591823560292198, 12.60653300113718167 ) ) ;
#26766=CARTESIAN_POINT ( 'NONE',  ( 77.00000000000001421, 170.2462022514548323, -7.872454543227099337E-15 ) ) ;
#26768=CARTESIAN_POINT ( 'NONE',  ( 61.71132485994280614, 155.0000000000000000, -15.00000000000002487 ) ) ;
#26770=DIRECTION ( 'NONE',  ( 0.000000000000000000, 0.000000000000000000, -1.000000000000000000 ) ) ;
#26771=CARTESIAN_POINT ( 'NONE',  ( 39.47499999726881015, 160.0630714827496206, -15.58253175000000823 ) ) ;
#26773=CARTESIAN_POINT ( 'NONE',  ( 78.22499999726881015, 149.9369285172503510, 15.58253174999999580 ) ) ;
#26777=CARTESIAN_POINT ( 'NONE',  ( 43.09999999453763309, 150.2886644046228639, 14.49999999999999645 ) ) ;
#26792=CARTESIAN_POINT ( 'NONE',  ( 50.18867513459482410, 140.7341522555726669, 4.635254915624211769 ) ) ;
#26797=EDGE_LOOP ( 'NONE', ( #2634, #28738, #17924, #31901 ) ) ;
#26798=CARTESIAN_POINT ( 'NONE',  ( 39.32499999726881157, 164.1591823560292198, -12.60653300113719766 ) ) ;
#26802=CARTESIAN_POINT ( 'NONE',  ( 86.32499999726880446, 145.8408176439707802, 12.60653300113718345 ) ) ;
#26806=AXIS2_PLACEMENT_3D ( 'NONE', #28850, #7402, #9959 ) ;
#26807=CARTESIAN_POINT ( 'NONE',  ( 54.69999999999999574, 163.5228861582408797, -11.73074641843674470 ) ) ;
#26813=CARTESIAN_POINT ( 'NONE',  ( 55.42499999726879878, 168.2552932293087906, -9.630534252274385310 ) ) ;
#26816=CARTESIAN_POINT ( 'NONE',  ( 64.32499999726881867, 145.8408176439707802, 12.60653300113718345 ) ) ;
#26817=CARTESIAN_POINT ( 'NONE',  ( 76.47499999726881015, 149.9369285172503510, 15.58253174999999580 ) ) ;
#26821=CARTESIAN_POINT ( 'NONE',  ( 84.28867513459483973, 139.2280666364260071, -4.041636747397287284E-15 ) ) ;
#26832=CARTESIAN_POINT ( 'NONE',  ( 63.51132485994280330, 146.1832212156128890, -12.13525491562423042 ) ) ;
#26840=CARTESIAN_POINT ( 'NONE',  ( 79.52499999726880731, 169.8198683612136222, -4.815267126137197984 ) ) ;
#26843=CARTESIAN_POINT ( 'NONE',  ( 68.92499999726881299, 145.8408176439707802, -12.60653300113719588 ) ) ;
#26846=CARTESIAN_POINT ( 'NONE',  ( 67.71132485994280614, 155.0000000000000000, -15.00000000000002487 ) ) ;
#26848=CARTESIAN_POINT ( 'NONE',  ( 32.50000000000000000, 155.0000000000000000, -6.938893903907228378E-15 ) ) ;
#26849=CARTESIAN_POINT ( 'NONE',  ( 35.40000000000000568, 159.7113355953771077, 14.49999999999999289 ) ) ;
#26852=EDGE_CURVE ( 'NONE', #7110, #27265, #30868, .T. ) ;
#26859=CARTESIAN_POINT ( 'NONE',  ( 43.62499999726880873, 171.3844434931184253, -7.942151717890134290E-15 ) ) ;
#26860=( BOUNDED_CURVE ( )  B_SPLINE_CURVE ( 2, ( #30124, #19728, #14780, #22798, #22286, #25173, #15122, #33189, #17170, #22114, #11900 ),
 .UNSPECIFIED., .F., .T. ) 
 B_SPLINE_CURVE_WITH_KNOTS ( ( 3, 2, 2, 2, 2, 3 ),
 ( 0.9285714285714286031, 0.9321428571428571619, 0.9357142857142858317, 0.9392857142857143904, 0.9428571428571430602, 0.9464285714285716189 ),
 .UNSPECIFIED. ) 
 CURVE ( )  GEOMETRIC_REPRESENTATION_ITEM ( )  RATIONAL_B_SPLINE_CURVE ( ( 1.000000000000000000, 0.9510565162951534202, 1.000000000000000000, 0.9510565162951534202, 1.000000000000000000, 0.9510565162951534202, 1.000000000000000000, 0.9510565162951534202, 1.000000000000000000, 0.9510565162951504226, 1.000000000000003109 ) ) 
 REPRESENTATION_ITEM ( '' )  );
#26869=CARTESIAN_POINT ( 'NONE',  ( 83.39999999453762314, 141.2096805137202580, 4.480746418436733158 ) ) ;
#26876=VERTEX_POINT ( 'NONE', #8097 ) ;
#26880=CARTESIAN_POINT ( 'NONE',  ( 79.47499999726881015, 160.0630714827496206, -15.58253175000000823 ) ) ;
#26888=CARTESIAN_POINT ( 'NONE',  ( 68.37499999726881583, 155.0000000000000000, 15.58253174999999402 ) ) ;
#26889=ORIENTED_EDGE ( 'NONE', *, *, #24122, .F. ) ;
#26890=LINE ( 'NONE', #3050, #3138 ) ;
#26892=CARTESIAN_POINT ( 'NONE',  ( 52.78867513459482552, 155.0000000000000000, -15.00000000000002487 ) ) ;
#26896=CARTESIAN_POINT ( 'NONE',  ( 80.71132485994280614, 155.0000000000000000, 15.00000000000001243 ) ) ;
#26898=CARTESIAN_POINT ( 'NONE',  ( 83.87499999726878741, 171.3844434931184253, -7.942151717890132712E-15 ) ) ;
#26902=CARTESIAN_POINT ( 'NONE',  ( 35.82499999726880446, 168.2552932293087906, 9.630534252274372875 ) ) ;
#26903=CARTESIAN_POINT ( 'NONE',  ( 127.5000000000000000, 229.9533188057749555, 74.95331880577313655 ) ) ;
#26904=DIRECTION ( 'NONE',  ( 0.000000000000000000, 0.000000000000000000, -1.000000000000000000 ) ) ;
#26907=CARTESIAN_POINT ( 'NONE',  ( 64.97499999726881015, 140.1801316387863778, -4.815267126137194431 ) ) ;
#26914=CARTESIAN_POINT ( 'NONE',  ( 65.09999999453764019, 150.2886644046228639, 14.49999999999999645 ) ) ;
#26918=CARTESIAN_POINT ( 'NONE',  ( 37.08867513459482268, 167.7597621252805880, -9.270509831248443078 ) ) ;
#26920=CARTESIAN_POINT ( 'NONE',  ( 59.51132485994281041, 146.1832212156128890, -12.13525491562423042 ) ) ;
#26924=CARTESIAN_POINT ( 'NONE',  ( 33.24999999726880873, 155.0000000000000000, -15.58253175000000823 ) ) ;
#26930=CARTESIAN_POINT ( 'NONE',  ( 48.87499999726880873, 138.6155565068815747, -3.929120461958505118E-15 ) ) ;
#26932=CARTESIAN_POINT ( 'NONE',  ( 59.52499999726881441, 169.8198683612136222, -4.815267126137197984 ) ) ;
#26935=FACE_OUTER_BOUND ( 'NONE', #9490, .T. ) ;
#26937=CARTESIAN_POINT ( 'NONE',  ( 57.87499999726880873, 171.3844434931184253, -7.942151717890132712E-15 ) ) ;
#26941=CARTESIAN_POINT ( 'NONE',  ( 73.09999999999999432, 168.7903194862797420, 4.480746418436729606 ) ) ;
#26942=CARTESIAN_POINT ( 'NONE',  ( 61.91132485994280898, 163.8167787843871110, -12.13525491562423397 ) ) ;
#26943=CYLINDRICAL_SURFACE ( 'NONE', #22946, 15.00000000000001776 ) ;
#26946=CARTESIAN_POINT ( 'NONE',  ( 46.77499999726881441, 140.1801316387863778, 4.815267126137185549 ) ) ;
#26949=CARTESIAN_POINT ( 'NONE',  ( 78.92499999726881299, 145.8408176439707802, -12.60653300113719588 ) ) ;
#26952=CARTESIAN_POINT ( 'NONE',  ( 38.99999999453762456, 155.0000000000000000, 14.49999999999999467 ) ) ;
#26958=DIRECTION ( 'NONE',  ( 0.000000000000000000, 0.000000000000000000, -1.000000000000000000 ) ) ;
#26968=CARTESIAN_POINT ( 'NONE',  ( 39.92499999726881299, 164.1591823560292198, 12.60653300113718167 ) ) ;
#26970=CARTESIAN_POINT ( 'NONE',  ( 41.67499999726881299, 168.2552932293087906, -9.630534252274385310 ) ) ;
#26973=CARTESIAN_POINT ( 'NONE',  ( 52.10000000000000142, 141.2096805137202580, -4.480746418436742040 ) ) ;
#26975=CARTESIAN_POINT ( 'NONE',  ( 76.78867513459483973, 155.0000000000000000, -15.00000000000002487 ) ) ;
#26977=ADVANCED_FACE ( 'NONE', ( #581 ), #29804, .F. ) ;
#26978=CARTESIAN_POINT ( 'NONE',  ( 55.52499999726881441, 169.8198683612136222, -4.815267126137197984 ) ) ;
#26982=CARTESIAN_POINT ( 'NONE',  ( 67.72499999726881015, 169.8198683612136222, 4.815267126137181997 ) ) ;
#26983=CARTESIAN_POINT ( 'NONE',  ( 78.37499999726883004, 155.0000000000000000, 15.58253174999999402 ) ) ;
#26987=CARTESIAN_POINT ( 'NONE',  ( 84.78867513459482552, 155.0000000000000000, -15.00000000000002487 ) ) ;
#27000=ORIENTED_EDGE ( 'NONE', *, *, #5845, .T. ) ;
#27002=ORIENTED_EDGE ( 'NONE', *, *, #27020, .F. ) ;
#27007=CARTESIAN_POINT ( 'NONE',  ( 85.12499999726881583, 155.0000000000000000, -15.58253175000000823 ) ) ;
#27010=EDGE_CURVE ( 'NONE', #32735, #7971, #18066, .T. ) ;
#27011=CARTESIAN_POINT ( 'NONE',  ( 78.22499999726881015, 149.9369285172503510, 15.58253174999999580 ) ) ;
#27016=CARTESIAN_POINT ( 'NONE',  ( 32.80000000000000426, 167.3344367211045096, -8.961492836873482304 ) ) ;
#27020=EDGE_CURVE ( 'NONE', #12770, #14229, #21531, .T. ) ;
#27026=CARTESIAN_POINT ( 'NONE',  ( 46.52499999726881441, 140.1801316387863778, 4.815267126137185549 ) ) ;
#27033=CARTESIAN_POINT ( 'NONE',  ( 88.99999999453763166, 155.0000000000000000, 14.49999999999999467 ) ) ;
#27044=CARTESIAN_POINT ( 'NONE',  ( 73.37499999726881583, 155.0000000000000000, -15.58253175000000823 ) ) ;
#27049=CARTESIAN_POINT ( 'NONE',  ( 85.27499999726879309, 149.9369285172503510, -15.58253175000000823 ) ) ;
#27050=DIRECTION ( 'NONE',  ( 1.000000000000000000, 0.000000000000000000, 0.000000000000000000 ) ) ;
#27051=CARTESIAN_POINT ( 'NONE',  ( 59.68867513459483121, 159.8737954434935489, 15.00000000000006040 ) ) ;
#27055=CARTESIAN_POINT ( 'NONE',  ( 67.47499999726881015, 160.0630714827496206, -15.58253175000000823 ) ) ;
#27064=CARTESIAN_POINT ( 'NONE',  ( 81.87499999726880162, 171.3844434931184253, -7.942151717890132712E-15 ) ) ;
#27068=CARTESIAN_POINT ( 'NONE',  ( 47.92499999726881299, 164.1591823560292198, 12.60653300113718167 ) ) ;
#27070=DIRECTION ( 'NONE',  ( -1.000000000000000000, 0.000000000000000000, 0.000000000000000000 ) ) ;
#27080=CARTESIAN_POINT ( 'NONE',  ( 67.69999999453763451, 142.6655632788954620, -8.961492836873480528 ) ) ;
#27084=EDGE_CURVE ( 'NONE', #23379, #20617, #6304, .T. ) ;
#27094=ADVANCED_FACE ( 'NONE', ( #4224 ), #13364, .F. ) ;
#27100=DIRECTION ( 'NONE',  ( 1.000000000000000000, 0.000000000000000000, 0.000000000000000000 ) ) ;
#27102=CARTESIAN_POINT ( 'NONE',  ( 47.47499999726881015, 160.0630714827496206, -15.58253175000000823 ) ) ;
#27104=ORIENTED_EDGE ( 'NONE', *, *, #14090, .T. ) ;
#27105=CARTESIAN_POINT ( 'NONE',  ( 57.32499999726881157, 164.1591823560292198, -12.60653300113719766 ) ) ;
#27111=CARTESIAN_POINT ( 'NONE',  ( 59.77499999726881441, 169.8198683612136222, -4.815267126137197984 ) ) ;
#27115=CARTESIAN_POINT ( 'NONE',  ( 82.50000000000000000, 155.0000000000000000, -14.50000000000000711 ) ) ;
#27116=CARTESIAN_POINT ( 'NONE',  ( 62.21132485994281325, 170.7719333635740497, -7.904646289410545231E-15 ) ) ;
#27121=CARTESIAN_POINT ( 'NONE',  ( 46.47499999726880304, 149.9369285172503510, 15.58253174999999580 ) ) ;
#27124=CARTESIAN_POINT ( 'NONE',  ( 77.52499999726880731, 169.8198683612136222, -4.815267126137197984 ) ) ;
#27127=CARTESIAN_POINT ( 'NONE',  ( 47.69999999453762740, 142.6655632788954620, -8.961492836873480528 ) ) ;
#27129=DIRECTION ( 'NONE',  ( 1.000000000000000000, 0.000000000000000000, 0.000000000000000000 ) ) ;
#27133=DIRECTION ( 'NONE',  ( 1.000000000000000000, 0.000000000000000000, 0.000000000000000000 ) ) ;
#27138=CARTESIAN_POINT ( 'NONE',  ( 79.68867513459481700, 159.8737954434934920, 15.00000000000007994 ) ) ;
#27142=CYLINDRICAL_SURFACE ( 'NONE', #16475, 15.00000000000001776 ) ;
#27146=CARTESIAN_POINT ( 'NONE',  ( 40.82499999726880446, 141.7447067706911810, -9.630534252274385310 ) ) ;
#27150=CARTESIAN_POINT ( 'NONE',  ( 43.17499999726881299, 145.8408176439707802, -12.60653300113719588 ) ) ;
#27154=CARTESIAN_POINT ( 'NONE',  ( 54.50000000000000711, 155.0000000000000000, -14.50000000000000711 ) ) ;
#27155=FACE_BOUND ( 'NONE', #23822, .T. ) ;
#27159=CARTESIAN_POINT ( 'NONE',  ( 58.92499999726881299, 145.8408176439707802, -12.60653300113719588 ) ) ;
#27162=CARTESIAN_POINT ( 'NONE',  ( 43.11132485994280472, 140.7341522555726669, 4.635254915624211769 ) ) ;
#27163=CARTESIAN_POINT ( 'NONE',  ( 82.57499999726880446, 145.8408176439707802, 12.60653300113718345 ) ) ;
#27183=CARTESIAN_POINT ( 'NONE',  ( 84.12499999726881583, 155.0000000000000000, 15.58253174999999402 ) ) ;
#27187=CARTESIAN_POINT ( 'NONE',  ( 74.32499999726881867, 145.8408176439707802, 12.60653300113718345 ) ) ;
#27190=CARTESIAN_POINT ( 'NONE',  ( 34.39999999999999858, 150.2886644046228639, -14.50000000000000888 ) ) ;
#27196=DIRECTION ( 'NONE',  ( 1.000000000000000000, 0.000000000000000000, 0.000000000000000000 ) ) ;
#27197=CARTESIAN_POINT ( 'NONE',  ( 51.62499999726881583, 171.3844434931184253, -7.942151717890134290E-15 ) ) ;
#27199=CARTESIAN_POINT ( 'NONE',  ( 41.21132485994281325, 139.2280666364260071, -4.041636747397287284E-15 ) ) ;
#27204=CARTESIAN_POINT ( 'NONE',  ( 85.89999999453762314, 150.2886644046228639, -14.50000000000000888 ) ) ;
#27207=EDGE_CURVE ( 'NONE', #11089, #33178, #18317, .T. ) ;
#27208=( BOUNDED_CURVE ( )  B_SPLINE_CURVE ( 2, ( #6559, #16943, #27338, #27507, #3498, #29730, #21888, #4003, #30067, #6732, #29564 ),
 .UNSPECIFIED., .F., .T. ) 
 B_SPLINE_CURVE_WITH_KNOTS ( ( 3, 2, 2, 2, 2, 3 ),
 ( 0.08928571428571423219, 0.09285714285714280480, 0.09642857142857139130, 0.09999999999999996392, 0.1035714285714285365, 0.1071428571428571092 ),
 .UNSPECIFIED. ) 
 CURVE ( )  GEOMETRIC_REPRESENTATION_ITEM ( )  RATIONAL_B_SPLINE_CURVE ( ( 1.000000000000000666, 0.9510565162951526430, 1.000000000000000000, 0.9510565162951534202, 1.000000000000000000, 0.9510565162951534202, 1.000000000000000000, 0.9510565162951534202, 1.000000000000000000, 0.9510565162951537532, 0.9999999999999996669 ) ) 
 REPRESENTATION_ITEM ( '' )  );
#27210=CARTESIAN_POINT ( 'NONE',  ( 125.5000000000000000, 261.0000000000000000, 2.149999999999985256 ) ) ;
#27214=CARTESIAN_POINT ( 'NONE',  ( 74.47499999726881015, 149.9369285172503510, 15.58253174999999580 ) ) ;
#27218=CARTESIAN_POINT ( 'NONE',  ( 80.87499999726881583, 138.6155565068815747, -3.929120461958505118E-15 ) ) ;
#27224=CARTESIAN_POINT ( 'NONE',  ( 70.27499999726880731, 160.0630714827496206, 15.58253174999999224 ) ) ;
#27227=EDGE_CURVE ( 'NONE', #28697, #7596, #11529, .T. ) ;
#27228=DIRECTION ( 'NONE',  ( 1.000000000000000000, 0.000000000000000000, 0.000000000000000000 ) ) ;
#27229=CARTESIAN_POINT ( 'NONE',  ( 43.18867513459481700, 169.2658477444273331, -4.635254915624224203 ) ) ;
#27235=CARTESIAN_POINT ( 'NONE',  ( 47.82499999726881867, 168.2552932293087906, 9.630534252274372875 ) ) ;
#27237=CARTESIAN_POINT ( 'NONE',  ( 87.50000000000002842, 154.6566093261667163, -15.35392587765464079 ) ) ;
#27244=CARTESIAN_POINT ( 'NONE',  ( 32.50000000000000000, 155.0000000000000000, -13.00000000000002487 ) ) ;
#27247=CARTESIAN_POINT ( 'NONE',  ( 64.19999999453762030, 163.5228861582408797, -11.73074641843674470 ) ) ;
#27253=CARTESIAN_POINT ( 'NONE',  ( 76.71132485994280614, 155.0000000000000000, 15.00000000000001243 ) ) ;
#27257=CARTESIAN_POINT ( 'NONE',  ( 42.28867513459482552, 139.2280666364260071, -4.041636747397287284E-15 ) ) ;
#27260=( BOUNDED_CURVE ( )  B_SPLINE_CURVE ( 2, ( #3510, #11352, #21736, #20326, #27814, #9942, #11982, #12319, #30551, #30386, #33446 ),
 .UNSPECIFIED., .F., .T. ) 
 B_SPLINE_CURVE_WITH_KNOTS ( ( 3, 2, 2, 2, 2, 3 ),
 ( 0.4285714285714285476, 0.4321428571428571619, 0.4357142857142857206, 0.4392857142857142239, 0.4428571428571427826, 0.4464285714285713969 ),
 .UNSPECIFIED. ) 
 CURVE ( )  GEOMETRIC_REPRESENTATION_ITEM ( )  RATIONAL_B_SPLINE_CURVE ( ( 1.000000000000000000, 0.9510565162951534202, 1.000000000000000000, 0.9510565162951534202, 1.000000000000000000, 0.9510565162951534202, 1.000000000000000000, 0.9510565162951534202, 1.000000000000000000, 0.9510565162951541973, 0.9999999999999992228 ) ) 
 REPRESENTATION_ITEM ( '' )  );
#27264=CARTESIAN_POINT ( 'NONE',  ( 52.77499999726881441, 140.1801316387863778, 4.815267126137185549 ) ) ;
#27265=VERTEX_POINT ( 'NONE', #18651 ) ;
#27267=CARTESIAN_POINT ( 'NONE',  ( 67.01132485994281751, 142.2402378747194405, 9.270509831248432420 ) ) ;
#27272=CARTESIAN_POINT ( 'NONE',  ( 61.67499999726881299, 168.2552932293087906, -9.630534252274385310 ) ) ;
#27278=CARTESIAN_POINT ( 'NONE',  ( 82.99999999999998579, 170.2462022514548323, -7.872454543227099337E-15 ) ) ;
#27283=CARTESIAN_POINT ( 'NONE',  ( 42.17499999726881299, 164.1591823560292198, 12.60653300113718167 ) ) ;
#27287=CARTESIAN_POINT ( 'NONE',  ( 85.22499999726882436, 160.0630714827496206, -15.58253175000000823 ) ) ;
#27289=CARTESIAN_POINT ( 'NONE',  ( 125.5000000000000000, 155.0000000000000000, -6.938893903907228378E-15 ) ) ;
#27290=CARTESIAN_POINT ( 'NONE',  ( 44.89999999453763024, 159.7113355953771077, 14.49999999999999289 ) ) ;
#27301=CARTESIAN_POINT ( 'NONE',  ( 79.38867513459483405, 169.2658477444273331, 4.635254915624208216 ) ) ;
#27306=CARTESIAN_POINT ( 'NONE',  ( 33.77499999726880731, 169.8198683612136222, -4.815267126137197984 ) ) ;
#27308=CARTESIAN_POINT ( 'NONE',  ( 35.02499999726880020, 149.9369285172503510, -15.58253175000000823 ) ) ;
#27311=CARTESIAN_POINT ( 'NONE',  ( 38.17499999726881299, 164.1591823560292198, 12.60653300113718167 ) ) ;
#27315=CARTESIAN_POINT ( 'NONE',  ( 61.70000000000000284, 146.4771138417591203, 11.73074641843673227 ) ) ;
#27316=DIRECTION ( 'NONE',  ( 0.000000000000000000, 0.7071067811865475727, 0.7071067811865475727 ) ) ;
#27320=CARTESIAN_POINT ( 'NONE',  ( 56.42499999726881299, 141.7447067706911810, 9.630534252274376428 ) ) ;
#27323=CARTESIAN_POINT ( 'NONE',  ( 45.71132485994280614, 155.0000000000000000, -15.00000000000002487 ) ) ;
#27325=CARTESIAN_POINT ( 'NONE',  ( 83.97499999726882436, 169.8198683612136222, 4.815267126137181997 ) ) ;
#27328=CARTESIAN_POINT ( 'NONE',  ( 72.18867513459481700, 140.7341522555726669, 4.635254915624211769 ) ) ;
#27329=CARTESIAN_POINT ( 'NONE',  ( 53.28867513459483263, 170.7719333635740497, -7.904646289410545231E-15 ) ) ;
#27338=CARTESIAN_POINT ( 'NONE',  ( 38.91132485994280898, 146.1832212156128890, 12.13525491562421976 ) ) ;
#27342=VERTEX_POINT ( 'NONE', #24252 ) ;
#27343=CARTESIAN_POINT ( 'NONE',  ( 84.82499999726880446, 141.7447067706911810, -9.630534252274387086 ) ) ;
#27348=CARTESIAN_POINT ( 'NONE',  ( 78.82499999726881867, 141.7447067706911810, -9.630534252274385310 ) ) ;
#27351=CARTESIAN_POINT ( 'NONE',  ( 87.49999999999998579, 168.4103784519322176, 7.072258346144660202 ) ) ;
#27353=CARTESIAN_POINT ( 'NONE',  ( 43.60000000000000142, 150.2886644046228639, 14.49999999999999645 ) ) ;
#27357=CARTESIAN_POINT ( 'NONE',  ( 32.50000000000000000, 155.0000000000000000, -6.938893903907228378E-15 ) ) ;
#27358=CARTESIAN_POINT ( 'NONE',  ( 78.58867513459483689, 146.1832212156128890, -12.13525491562423042 ) ) ;
#27359=CARTESIAN_POINT ( 'NONE',  ( 32.50000000000000000, 155.0000000000000000, -15.00000000000002487 ) ) ;
#27360=CARTESIAN_POINT ( 'NONE',  ( 49.22499999726881725, 160.0630714827496206, -15.58253175000000823 ) ) ;
#27368=CARTESIAN_POINT ( 'NONE',  ( 85.59999999453762598, 141.2096805137202580, -4.480746418436742040 ) ) ;
#27377=CARTESIAN_POINT ( 'NONE',  ( 70.87499999726878741, 138.6155565068815463, -3.929120461958505118E-15 ) ) ;
#27380=CARTESIAN_POINT ( 'NONE',  ( 81.87499999726881583, 171.3844434931184253, -7.942151717890134290E-15 ) ) ;
#27383=CARTESIAN_POINT ( 'NONE',  ( 125.5000000000000000, 152.8499999999996533, -106.0000000000000000 ) ) ;
#27390=CARTESIAN_POINT ( 'NONE',  ( 52.68867513459483831, 150.1262045565068206, -15.00000000000030909 ) ) ;
#27397=CARTESIAN_POINT ( 'NONE',  ( 87.87499999726877320, 171.3844434931184253, -7.942151717890132712E-15 ) ) ;
#27398=CIRCLE ( 'NONE', #7821, 98.00000000000000000 ) ;
#27402=CARTESIAN_POINT ( 'NONE',  ( 43.22499999726881015, 160.0630714827496206, -15.58253175000000823 ) ) ;
#27404=CARTESIAN_POINT ( 'NONE',  ( 34.32499999726881157, 145.8408176439707802, 12.60653300113718345 ) ) ;
#27407=( BOUNDED_CURVE ( )  B_SPLINE_CURVE ( 2, ( #15359, #10271, #7703, #30704, #18086, #15691, #28483, #5138, #15192, #15525, #2590 ),
 .UNSPECIFIED., .F., .T. ) 
 B_SPLINE_CURVE_WITH_KNOTS ( ( 3, 2, 2, 2, 2, 3 ),
 ( 0.2321428571428572063, 0.2357142857142857373, 0.2392857142857142960, 0.2428571428571428548, 0.2464285714285714135, 0.2499999999999999445 ),
 .UNSPECIFIED. ) 
 CURVE ( )  GEOMETRIC_REPRESENTATION_ITEM ( )  RATIONAL_B_SPLINE_CURVE ( ( 0.9999999999999992228, 0.9510565162951541973, 1.000000000000000000, 0.9510565162951534202, 1.000000000000000000, 0.9510565162951534202, 1.000000000000000000, 0.9510565162951534202, 1.000000000000000000, 0.9510565162951541973, 0.9999999999999992228 ) ) 
 REPRESENTATION_ITEM ( '' )  );
#27409=EDGE_CURVE ( 'NONE', #3255, #26876, #23793, .T. ) ;
#27411=CARTESIAN_POINT ( 'NONE',  ( 76.38867513459481984, 140.7341522555726669, -4.635254915624220651 ) ) ;
#27415=CARTESIAN_POINT ( 'NONE',  ( 65.19999999453762030, 146.4771138417591203, 11.73074641843673227 ) ) ;
#27416=ORIENTED_EDGE ( 'NONE', *, *, #8272, .T. ) ;
#27427=CARTESIAN_POINT ( 'NONE',  ( 87.49999999999997158, 161.8888959785116413, -14.01425902168828408 ) ) ;
#27429=VERTEX_POINT ( 'NONE', #1096 ) ;
#27431=EDGE_CURVE ( 'NONE', #8808, #3666, #25464, .T. ) ;
#27432=CARTESIAN_POINT ( 'NONE',  ( 54.91132485994280898, 146.1832212156128890, 12.13525491562421976 ) ) ;
#27434=CARTESIAN_POINT ( 'NONE',  ( 50.17499999726881299, 164.1591823560292198, 12.60653300113718167 ) ) ;
#27437=CARTESIAN_POINT ( 'NONE',  ( 67.71132485994280614, 155.0000000000000000, -15.00000000000002487 ) ) ;
#27443=CARTESIAN_POINT ( 'NONE',  ( 60.27499999726880020, 160.0630714827496206, 15.58253174999999402 ) ) ;
#27445=FACE_OUTER_BOUND ( 'NONE', #363, .T. ) ;
#27448=CARTESIAN_POINT ( 'NONE',  ( 80.19999999999997442, 142.6655632788954620, -8.961492836873480528 ) ) ;
#27451=CARTESIAN_POINT ( 'NONE',  ( 32.50000000000000000, 155.0000000000000000, -6.938893903907228378E-15 ) ) ;
#27452=CARTESIAN_POINT ( 'NONE',  ( 46.87499999726880873, 138.6155565068815463, -3.929120461958505118E-15 ) ) ;
#27454=CARTESIAN_POINT ( 'NONE',  ( 81.52499999726880731, 169.8198683612136222, -4.815267126137197984 ) ) ;
#27456=CARTESIAN_POINT ( 'NONE',  ( 64.71132485994279193, 155.0000000000000000, 15.00000000000001243 ) ) ;
#27457=CARTESIAN_POINT ( 'NONE',  ( 48.39999999453763024, 168.7903194862797420, -4.480746418436745593 ) ) ;
#27460=CARTESIAN_POINT ( 'NONE',  ( 61.11132485994280472, 140.7341522555726669, 4.635254915624211769 ) ) ;
#27476=CARTESIAN_POINT ( 'NONE',  ( 38.82499999726881157, 141.7447067706911810, -9.630534252274385310 ) ) ;
#27480=EDGE_CURVE ( 'NONE', #5476, #28404, #29241, .T. ) ;
#27481=CARTESIAN_POINT ( 'NONE',  ( 39.27499999726880020, 149.9369285172503510, -15.58253175000000823 ) ) ;
#27486=CARTESIAN_POINT ( 'NONE',  ( 61.59999999999999432, 150.2886644046228639, 14.49999999999999645 ) ) ;
#27491=CARTESIAN_POINT ( 'NONE',  ( 62.62499999726881583, 138.6155565068815463, -3.929120461958505118E-15 ) ) ;
#27495=CARTESIAN_POINT ( 'NONE',  ( 81.17499999726882720, 145.8408176439707802, -12.60653300113719588 ) ) ;
#27498=VERTEX_POINT ( 'NONE', #32094 ) ;
#27507=CARTESIAN_POINT ( 'NONE',  ( 39.01132485994280330, 142.2402378747194405, 9.270509831248432420 ) ) ;
#27514=CARTESIAN_POINT ( 'NONE',  ( 81.72499999726881015, 169.8198683612136222, 4.815267126137181997 ) ) ;
#27516=CARTESIAN_POINT ( 'NONE',  ( 69.31132485994278625, 140.7341522555726669, -4.635254915624220651 ) ) ;
#27517=CARTESIAN_POINT ( 'NONE',  ( 73.22499999726881015, 160.0630714827496206, -15.58253175000000823 ) ) ;
#27520=CARTESIAN_POINT ( 'NONE',  ( 87.50000000000002842, 170.3903390413697707, -0.7067623181846339753 ) ) ;
#27521=CARTESIAN_POINT ( 'NONE',  ( 44.79999999999999005, 167.3344367211045096, -8.961492836873482304 ) ) ;
#27526=CARTESIAN_POINT ( 'NONE',  ( 51.92499999726880588, 164.1591823560292198, 12.60653300113718167 ) ) ;
#27527=CARTESIAN_POINT ( 'NONE',  ( 66.27499999726880731, 160.0630714827496206, 15.58253174999999402 ) ) ;
#27534=CARTESIAN_POINT ( 'NONE',  ( 85.99999999453764588, 155.0000000000000000, -14.50000000000000711 ) ) ;
#27542=CARTESIAN_POINT ( 'NONE',  ( 69.97499999726881015, 169.8198683612136222, 4.815267126137181997 ) ) ;
#27545=VECTOR ( 'NONE', #28646, 1000.000000000000000 ) ;
#27546=CARTESIAN_POINT ( 'NONE',  ( 85.67499999726881299, 168.2552932293087906, -9.630534252274387086 ) ) ;
#27547=CYLINDRICAL_SURFACE ( 'NONE', #20585, 15.00000000000001776 ) ;
#27556=DIRECTION ( 'NONE',  ( 1.000000000000000000, 0.000000000000000000, 0.000000000000000000 ) ) ;
#27563=CARTESIAN_POINT ( 'NONE',  ( 44.52499999726881441, 140.1801316387863778, 4.815267126137185549 ) ) ;
#27564=CARTESIAN_POINT ( 'NONE',  ( 33.32499999726881157, 164.1591823560292198, -12.60653300113719766 ) ) ;
#27570=CARTESIAN_POINT ( 'NONE',  ( 76.28867513459483973, 139.2280666364260071, -4.041636747397287284E-15 ) ) ;
#27575=CARTESIAN_POINT ( 'NONE',  ( 68.49999999453761745, 170.2462022514548323, -7.872454543227099337E-15 ) ) ;
#27576=VERTEX_POINT ( 'NONE', #11487 ) ;
#27580=CARTESIAN_POINT ( 'NONE',  ( 76.01132485994281751, 167.7597621252805880, -9.270509831248443078 ) ) ;
#27590=CARTESIAN_POINT ( 'NONE',  ( 85.11132485994279762, 140.7341522555726669, 4.635254915624211769 ) ) ;
#27594=CARTESIAN_POINT ( 'NONE',  ( 58.17499999726881299, 164.1591823560292198, 12.60653300113718167 ) ) ;
#27595=ORIENTED_EDGE ( 'NONE', *, *, #7298, .F. ) ;
#27601=CARTESIAN_POINT ( 'NONE',  ( 64.17499999726879878, 164.1591823560292198, 12.60653300113718167 ) ) ;
#27607=CARTESIAN_POINT ( 'NONE',  ( 78.89999999999999147, 168.7903194862797420, -4.480746418436745593 ) ) ;
#27611=FACE_OUTER_BOUND ( 'NONE', #19132, .T. ) ;
#27612=CARTESIAN_POINT ( 'NONE',  ( 41.67499999726881299, 168.2552932293087906, -9.630534252274385310 ) ) ;
#27614=CARTESIAN_POINT ( 'NONE',  ( 80.82499999726880446, 141.7447067706911810, -9.630534252274385310 ) ) ;
#27617=CARTESIAN_POINT ( 'NONE',  ( 50.39999999453763024, 168.7903194862797420, -4.480746418436745593 ) ) ;
#27623=DIRECTION ( 'NONE',  ( 1.000000000000000000, 0.000000000000000000, 0.000000000000000000 ) ) ;
#27638=CARTESIAN_POINT ( 'NONE',  ( 35.97499999726881015, 169.8198683612136222, 4.815267126137181997 ) ) ;
#27640=CARTESIAN_POINT ( 'NONE',  ( 46.12499999726880873, 155.0000000000000000, 15.58253174999999402 ) ) ;
#27645=CARTESIAN_POINT ( 'NONE',  ( 42.27499999726880731, 160.0630714827496206, 15.58253174999999402 ) ) ;
#27646=DIRECTION ( 'NONE',  ( 1.000000000000000000, 0.000000000000000000, 0.000000000000000000 ) ) ;
#27651=CARTESIAN_POINT ( 'NONE',  ( 58.89999999999999858, 168.7903194862797420, -4.480746418436745593 ) ) ;
#27658=CARTESIAN_POINT ( 'NONE',  ( 66.72499999726881015, 140.1801316387863778, -4.815267126137194431 ) ) ;
#27662=CARTESIAN_POINT ( 'NONE',  ( 79.97499999726881015, 169.8198683612136222, 4.815267126137181997 ) ) ;
#27670=CARTESIAN_POINT ( 'NONE',  ( 127.5000000000000000, 48.99999999999998579, -1.387778780781445676E-14 ) ) ;
#27676=CIRCLE ( 'NONE', #18972, 2.149999999999984812 ) ;
#27680=CARTESIAN_POINT ( 'NONE',  ( 70.21132485994283456, 170.7719333635740497, -7.904646289410545231E-15 ) ) ;
#27684=AXIS2_PLACEMENT_3D ( 'NONE', #597, #9234, #18497 ) ;
#27685=CARTESIAN_POINT ( 'NONE',  ( 84.22499999726881015, 149.9369285172503510, 15.58253174999999580 ) ) ;
#27688=CARTESIAN_POINT ( 'NONE',  ( 74.62499999726883004, 138.6155565068815463, -3.929120461958505118E-15 ) ) ;
#27692=CARTESIAN_POINT ( 'NONE',  ( 40.40000000000000568, 150.2886644046228639, -14.50000000000000888 ) ) ;
#27698=LINE ( 'NONE', #4360, #31177 ) ;
#27701=CARTESIAN_POINT ( 'NONE',  ( 50.62499999726880873, 138.6155565068815747, -3.929120461958505118E-15 ) ) ;
#27702=CARTESIAN_POINT ( 'NONE',  ( 65.37499999726881583, 155.0000000000000000, -15.58253175000000823 ) ) ;
#27704=CARTESIAN_POINT ( 'NONE',  ( 117.5000000000000142, 155.0000000000000000, -6.938893903907228378E-15 ) ) ;
#27707=EDGE_CURVE ( 'NONE', #25104, #27576, #11986, .T. ) ;
#27711=CARTESIAN_POINT ( 'NONE',  ( 125.5000000000000000, 228.4330392262228600, -76.47359838532524634 ) ) ;
#27715=ADVANCED_FACE ( 'NONE', ( #22888 ), #25098, .T. ) ;
#27718=ORIENTED_EDGE ( 'NONE', *, *, #12294, .T. ) ;
#27721=CARTESIAN_POINT ( 'NONE',  ( 70.97499999726881015, 140.1801316387863778, -4.815267126137194431 ) ) ;
#27725=CARTESIAN_POINT ( 'NONE',  ( 80.27499999726879309, 160.0630714827496206, 15.58253174999999224 ) ) ;
#27728=CARTESIAN_POINT ( 'NONE',  ( 54.72499999726881015, 140.1801316387863778, -4.815267126137194431 ) ) ;
#27740=CARTESIAN_POINT ( 'NONE',  ( 45.82499999726881157, 168.2552932293087906, 9.630534252274372875 ) ) ;
#27742=CARTESIAN_POINT ( 'NONE',  ( 34.92499999726881299, 145.8408176439707802, -12.60653300113719588 ) ) ;
#27748=CARTESIAN_POINT ( 'NONE',  ( 54.68867513459483121, 150.1262045565066785, -15.00000000000021316 ) ) ;
#27751=CARTESIAN_POINT ( 'NONE',  ( 70.59999999453762598, 168.7903194862797420, 4.480746418436729606 ) ) ;
#27758=ORIENTED_EDGE ( 'NONE', *, *, #23044, .F. ) ;
#27766=CARTESIAN_POINT ( 'NONE',  ( 54.87499999726880873, 138.6155565068815747, -3.929120461958505118E-15 ) ) ;
#27767=ORIENTED_EDGE ( 'NONE', *, *, #3882, .T. ) ;
#27769=DIRECTION ( 'NONE',  ( 1.000000000000000000, 0.000000000000000000, 0.000000000000000000 ) ) ;
#27772=CARTESIAN_POINT ( 'NONE',  ( 65.67499999726881299, 168.2552932293087906, -9.630534252274385310 ) ) ;
#27774=CARTESIAN_POINT ( 'NONE',  ( 69.88867513459481984, 150.1262045565062238, 14.99999999999987388 ) ) ;
#27779=CARTESIAN_POINT ( 'NONE',  ( 78.50000000000000000, 155.0000000000000000, -14.50000000000000711 ) ) ;
#27784=CARTESIAN_POINT ( 'NONE',  ( 51.27499999726880731, 149.9369285172503510, -15.58253175000000823 ) ) ;
#27786=CARTESIAN_POINT ( 'NONE',  ( 83.22499999726879594, 160.0630714827496206, -15.58253175000000823 ) ) ;
#27789=CARTESIAN_POINT ( 'NONE',  ( 45.39999999453763024, 141.2096805137202580, 4.480746418436733158 ) ) ;
#27795=CYLINDRICAL_SURFACE ( 'NONE', #29743, 15.00000000000001776 ) ;
#27796=ORIENTED_EDGE ( 'NONE', *, *, #6328, .F. ) ;
#27803=DIRECTION ( 'NONE',  ( 1.000000000000000000, 0.000000000000000000, 0.000000000000000000 ) ) ;
#27805=CARTESIAN_POINT ( 'NONE',  ( 36.07499999726880446, 168.2552932293087906, 9.630534252274372875 ) ) ;
#27807=CARTESIAN_POINT ( 'NONE',  ( 42.02499999726880731, 160.0630714827496206, 15.58253174999999402 ) ) ;
#27811=CARTESIAN_POINT ( 'NONE',  ( 49.97499999726881725, 169.8198683612136222, 4.815267126137181997 ) ) ;
#27814=CARTESIAN_POINT ( 'NONE',  ( 58.11132485994280472, 169.2658477444273331, -4.635254915624224203 ) ) ;
#27815=CARTESIAN_POINT ( 'NONE',  ( 62.70000000000000284, 163.5228861582408797, -11.73074641843674470 ) ) ;
#27817=CARTESIAN_POINT ( 'NONE',  ( 64.71132485994279193, 155.0000000000000000, 15.00000000000001243 ) ) ;
#27821=CARTESIAN_POINT ( 'NONE',  ( 67.12499999726881583, 155.0000000000000000, -15.58253175000000823 ) ) ;
#27824=CARTESIAN_POINT ( 'NONE',  ( 42.91132485994280188, 146.1832212156128890, 12.13525491562421976 ) ) ;
#27826=CARTESIAN_POINT ( 'NONE',  ( 84.97499999726882436, 140.1801316387863778, -4.815267126137194431 ) ) ;
#27828=LINE ( 'NONE', #22050, #26262 ) ;
#27843=ORIENTED_EDGE ( 'NONE', *, *, #27849, .F. ) ;
#27847=CARTESIAN_POINT ( 'NONE',  ( 72.67499999726881299, 141.7447067706911810, 9.630534252274376428 ) ) ;
#27848=CARTESIAN_POINT ( 'NONE',  ( 85.92499999726881299, 164.1591823560292198, 12.60653300113718167 ) ) ;
#27849=EDGE_CURVE ( 'NONE', #31511, #10102, #11727, .T. ) ;
#27852=CARTESIAN_POINT ( 'NONE',  ( 87.50000000000005684, 169.8231623009795328, -4.699990950160915837 ) ) ;
#27854=CARTESIAN_POINT ( 'NONE',  ( 39.90000000000000568, 141.2096805137202580, 4.480746418436733158 ) ) ;
#27858=CARTESIAN_POINT ( 'NONE',  ( 73.41132485994282320, 142.2402378747194405, -9.270509831248439525 ) ) ;
#27860=CARTESIAN_POINT ( 'NONE',  ( 55.82499999726881157, 168.2552932293087906, 9.630534252274372875 ) ) ;
#27861=CARTESIAN_POINT ( 'NONE',  ( 60.67499999726881299, 141.7447067706911810, 9.630534252274376428 ) ) ;
#27871=CARTESIAN_POINT ( 'NONE',  ( 67.81132485994280046, 159.8737954434934920, -15.00000000000012434 ) ) ;
#27879=CARTESIAN_POINT ( 'NONE',  ( 81.17499999726882720, 145.8408176439707802, -12.60653300113719588 ) ) ;
#27884=EDGE_CURVE ( 'NONE', #7373, #18104, #33524, .T. ) ;
#27885=CARTESIAN_POINT ( 'NONE',  ( 69.82499999726879025, 168.2552932293087906, 9.630534252274372875 ) ) ;
#27888=CARTESIAN_POINT ( 'NONE',  ( 59.92499999726881299, 164.1591823560292198, 12.60653300113718167 ) ) ;
#27892=ORIENTED_EDGE ( 'NONE', *, *, #9401, .F. ) ;
#27899=EDGE_CURVE ( 'NONE', #20973, #18094, #21164, .T. ) ;
#27901=CARTESIAN_POINT ( 'NONE',  ( 45.78867513459482552, 155.0000000000000000, 15.00000000000001243 ) ) ;
#27906=CIRCLE ( 'NONE', #20892, 2.149999999999984812 ) ;
#27914=DIRECTION ( 'NONE',  ( 0.000000000000000000, 0.7071067811865506814, 0.7071067811865442421 ) ) ;
#27918=CARTESIAN_POINT ( 'NONE',  ( 71.29999999453761461, 142.6655632788954620, 8.961492836873471646 ) ) ;
#27923=CARTESIAN_POINT ( 'NONE',  ( 75.21132485994282035, 139.2280666364260071, -4.041636747397287284E-15 ) ) ;
#27926=ORIENTED_EDGE ( 'NONE', *, *, #7539, .T. ) ;
#27931=CARTESIAN_POINT ( 'NONE',  ( 58.28867513459482552, 139.2280666364260071, -4.041636747397287284E-15 ) ) ;
#27940=CARTESIAN_POINT ( 'NONE',  ( 57.87499999726880873, 171.3844434931184253, -7.942151717890134290E-15 ) ) ;
#27944=( NAMED_UNIT ( * ) PLANE_ANGLE_UNIT ( ) SI_UNIT ( $, .RADIAN. ) );
#27947=CARTESIAN_POINT ( 'NONE',  ( 65.17499999726881299, 145.8408176439707802, -12.60653300113719588 ) ) ;
#27953=CARTESIAN_POINT ( 'NONE',  ( 85.10000000000000853, 168.7903194862797420, 4.480746418436729606 ) ) ;
#27955=CARTESIAN_POINT ( 'NONE',  ( 32.50000000000000000, 155.0000000000000000, -15.00000000000002487 ) ) ;
#27957=DIRECTION ( 'NONE',  ( -1.000000000000000000, -0.000000000000000000, -0.000000000000000000 ) ) ;
#27958=CARTESIAN_POINT ( 'NONE',  ( 52.77499999726881441, 140.1801316387863778, 4.815267126137185549 ) ) ;
#27960=CARTESIAN_POINT ( 'NONE',  ( 84.12499999726881583, 155.0000000000000000, 15.58253174999999402 ) ) ;
#27964=CARTESIAN_POINT ( 'NONE',  ( 53.59999999453762598, 141.2096805137202580, -4.480746418436742040 ) ) ;
#27967=AXIS2_PLACEMENT_3D ( 'NONE', #30494, #9208, #6815 ) ;
#27968=CARTESIAN_POINT ( 'NONE',  ( 61.71132485994280614, 155.0000000000000000, -15.00000000000002487 ) ) ;
#27970=CARTESIAN_POINT ( 'NONE',  ( 125.5000000000000000, 155.0000000000010800, 106.0000000000000142 ) ) ;
#27977=ORIENTED_EDGE ( 'NONE', *, *, #5564, .T. ) ;
#27981=CARTESIAN_POINT ( 'NONE',  ( 39.27499999726880731, 149.9369285172503510, -15.58253175000000823 ) ) ;
#27982=ORIENTED_EDGE ( 'NONE', *, *, #13893, .T. ) ;
#27983=CARTESIAN_POINT ( 'NONE',  ( 45.52499999726881441, 169.8198683612136222, -4.815267126137197984 ) ) ;
#27988=CARTESIAN_POINT ( 'NONE',  ( 49.77499999726880731, 169.8198683612136222, -4.815267126137197984 ) ) ;
#27993=CARTESIAN_POINT ( 'NONE',  ( 60.39999999999999147, 150.2886644046228639, -14.50000000000000888 ) ) ;
#28000=CARTESIAN_POINT ( 'NONE',  ( 61.62499999726881583, 171.3844434931184253, -7.942151717890132712E-15 ) ) ;
#28002=EDGE_LOOP ( 'NONE', ( #6141, #32150, #28818, #19372 ) ) ;
#28004=CARTESIAN_POINT ( 'NONE',  ( 86.47499999726879594, 149.9369285172503510, 15.58253174999999580 ) ) ;
#28010=DIRECTION ( 'NONE',  ( 1.000000000000000000, 0.000000000000000000, 0.000000000000000000 ) ) ;
#28015=DIRECTION ( 'NONE',  ( 1.000000000000000000, 0.000000000000000000, 0.000000000000000000 ) ) ;
#28021=CARTESIAN_POINT ( 'NONE',  ( 33.91132485994280188, 163.8167787843871110, -12.13525491562423397 ) ) ;
#28023=CARTESIAN_POINT ( 'NONE',  ( 81.71132485994280614, 155.0000000000000000, -15.00000000000002487 ) ) ;
#28024=CARTESIAN_POINT ( 'NONE',  ( 83.62499999726881583, 171.3844434931184253, -7.942151717890132712E-15 ) ) ;
#28027=FACE_OUTER_BOUND ( 'NONE', #7448, .T. ) ;
#28030=CARTESIAN_POINT ( 'NONE',  ( 40.50000000000000000, 155.0000000000000000, -14.50000000000000711 ) ) ;
#28032=ADVANCED_FACE ( 'NONE', ( #7902 ), #28672, .F. ) ;
#28035=CARTESIAN_POINT ( 'NONE',  ( 73.01132485994281751, 142.2402378747194405, 9.270509831248432420 ) ) ;
#28037=CARTESIAN_POINT ( 'NONE',  ( 57.42499999726880588, 168.2552932293087906, -9.630534252274387086 ) ) ;
#28038=CARTESIAN_POINT ( 'NONE',  ( 69.37499999726881583, 155.0000000000000000, -15.58253175000000823 ) ) ;
#28040=FACE_BOUND ( 'NONE', #26338, .T. ) ;
#28048=CARTESIAN_POINT ( 'NONE',  ( 74.58867513459482268, 146.1832212156128890, -12.13525491562423042 ) ) ;
#28052=ORIENTED_EDGE ( 'NONE', *, *, #19753, .T. ) ;
#28056=CARTESIAN_POINT ( 'NONE',  ( 76.17499999726881299, 164.1591823560292198, 12.60653300113718167 ) ) ;
#28060=CARTESIAN_POINT ( 'NONE',  ( 71.62499999726881583, 171.3844434931184253, -7.942151717890134290E-15 ) ) ;
#28063=CARTESIAN_POINT ( 'NONE',  ( 65.32499999726881867, 164.1591823560292198, -12.60653300113719766 ) ) ;
#28065=ADVANCED_FACE ( 'NONE', ( #29502 ), #32388, .T. ) ;
#28079=CARTESIAN_POINT ( 'NONE',  ( 37.92499999726881299, 164.1591823560292198, 12.60653300113718167 ) ) ;
#28086=CARTESIAN_POINT ( 'NONE',  ( 54.58867513459482268, 146.1832212156128890, -12.13525491562423042 ) ) ;
#28089=CARTESIAN_POINT ( 'NONE',  ( 72.09999999453764019, 159.7113355953771077, -14.50000000000000888 ) ) ;
#28093=ADVANCED_FACE ( 'NONE', ( #6325 ), #3939, .F. ) ;
#28108=CARTESIAN_POINT ( 'NONE',  ( 55.07499999726880446, 141.7447067706911810, -9.630534252274387086 ) ) ;
#28111=CARTESIAN_POINT ( 'NONE',  ( 68.58867513459482268, 146.1832212156128890, -12.13525491562423042 ) ) ;
#28114=CARTESIAN_POINT ( 'NONE',  ( 67.17499999726881299, 145.8408176439707802, -12.60653300113719588 ) ) ;
#28116=CARTESIAN_POINT ( 'NONE',  ( 70.78867513459482552, 155.0000000000000000, -15.00000000000002487 ) ) ;
#28118=CYLINDRICAL_SURFACE ( 'NONE', #28255, 15.00000000000001776 ) ;
#28122=CARTESIAN_POINT ( 'NONE',  ( 33.42499999726881299, 168.2552932293087906, -9.630534252274385310 ) ) ;
#28124=CYLINDRICAL_SURFACE ( 'NONE', #14163, 15.00000000000001776 ) ;
#28127=CARTESIAN_POINT ( 'NONE',  ( 51.67499999726879878, 168.2552932293087906, -9.630534252274385310 ) ) ;
#28131=CARTESIAN_POINT ( 'NONE',  ( 32.50000000000000000, 155.0000000000000000, -6.938893903907228378E-15 ) ) ;
#28133=CYLINDRICAL_SURFACE ( 'NONE', #12469, 15.00000000000001776 ) ;
#28134=CARTESIAN_POINT ( 'NONE',  ( 56.09999999453763309, 159.7113355953771077, -14.50000000000000888 ) ) ;
#28139=CARTESIAN_POINT ( 'NONE',  ( 32.50000000000000000, 155.0000000000000000, 15.00000000000001243 ) ) ;
#28155=CARTESIAN_POINT ( 'NONE',  ( 39.17499999726881299, 145.8408176439707802, -12.60653300113719588 ) ) ;
#28158=CARTESIAN_POINT ( 'NONE',  ( 45.62499999726880162, 171.3844434931184253, -7.942151717890132712E-15 ) ) ;
#28162=CARTESIAN_POINT ( 'NONE',  ( 49.07499999726880446, 141.7447067706911810, -9.630534252274385310 ) ) ;
#28166=CARTESIAN_POINT ( 'NONE',  ( 69.50000000000000000, 155.0000000000000000, 14.49999999999999467 ) ) ;
#28173=CARTESIAN_POINT ( 'NONE',  ( 33.47499999726881015, 160.0630714827496206, -15.58253175000000823 ) ) ;
#28176=CARTESIAN_POINT ( 'NONE',  ( 68.92499999726881299, 145.8408176439707802, -12.60653300113719588 ) ) ;
#28181=CARTESIAN_POINT ( 'NONE',  ( 35.99999999453763166, 155.0000000000000000, -14.50000000000000711 ) ) ;
#28190=CARTESIAN_POINT ( 'NONE',  ( 66.78867513459482552, 155.0000000000000000, -15.00000000000002487 ) ) ;
#28193=ORIENTED_EDGE ( 'NONE', *, *, #22701, .T. ) ;
#28202=CARTESIAN_POINT ( 'NONE',  ( 80.42499999726879878, 141.7447067706911810, 9.630534252274376428 ) ) ;
#28203=DIRECTION ( 'NONE',  ( 1.000000000000000000, 0.000000000000000000, 0.000000000000000000 ) ) ;
#28208=CARTESIAN_POINT ( 'NONE',  ( 48.10000000000000142, 141.2096805137202580, -4.480746418436742040 ) ) ;
#28212=LINE ( 'NONE', #4475, #22407 ) ;
#28213=CARTESIAN_POINT ( 'NONE',  ( 57.72499999726881015, 169.8198683612136222, 4.815267126137181997 ) ) ;
#28214=CARTESIAN_POINT ( 'NONE',  ( 68.67499999726879878, 141.7447067706911810, 9.630534252274376428 ) ) ;
#28216=DIRECTION ( 'NONE',  ( 0.000000000000000000, 0.000000000000000000, -1.000000000000000000 ) ) ;
#28221=AXIS2_PLACEMENT_3D ( 'NONE', #7669, #28281, #3371 ) ;
#28229=EDGE_CURVE ( 'NONE', #11543, #9113, #15017, .T. ) ;
#28230=CARTESIAN_POINT ( 'NONE',  ( 89.50000000000001421, 155.0000000000000000, -6.938893903907228378E-15 ) ) ;
#28235=EDGE_LOOP ( 'NONE', ( #10955, #32114 ) ) ;
#28236=CARTESIAN_POINT ( 'NONE',  ( 77.07499999726881867, 141.7447067706911810, -9.630534252274385310 ) ) ;
#28239=CARTESIAN_POINT ( 'NONE',  ( 72.12499999726881583, 155.0000000000000000, 15.58253174999999402 ) ) ;
#28243=CARTESIAN_POINT ( 'NONE',  ( 66.32499999726881867, 145.8408176439707802, 12.60653300113718345 ) ) ;
#28246=ORIENTED_EDGE ( 'NONE', *, *, #25595, .T. ) ;
#28255=AXIS2_PLACEMENT_3D ( 'NONE', #15175, #33407, #25567 ) ;
#28259=CARTESIAN_POINT ( 'NONE',  ( 87.27499999726880731, 149.9369285172503510, -15.58253175000000823 ) ) ;
#28261=CARTESIAN_POINT ( 'NONE',  ( 40.32499999726881157, 145.8408176439707802, 12.60653300113718345 ) ) ;
#28269=CARTESIAN_POINT ( 'NONE',  ( 73.59999999453762598, 141.2096805137202580, -4.480746418436742040 ) ) ;
#28275=EDGE_CURVE ( 'NONE', #3255, #29401, #24395, .T. ) ;
#28281=DIRECTION ( 'NONE',  ( 1.000000000000000000, 0.000000000000000000, 0.000000000000000000 ) ) ;
#28286=CARTESIAN_POINT ( 'NONE',  ( 82.11132485994279762, 169.2658477444273331, -4.635254915624224203 ) ) ;
#28288=CARTESIAN_POINT ( 'NONE',  ( 57.17499999726881299, 145.8408176439707802, -12.60653300113719588 ) ) ;
#28292=SURFACE_STYLE_USAGE ( .BOTH. , #2398 ) ;
#28295=CARTESIAN_POINT ( 'NONE',  ( 67.77499999726880731, 169.8198683612136222, -4.815267126137197984 ) ) ;
#28302=CARTESIAN_POINT ( 'NONE',  ( 87.50000000000000000, 155.0000000000000000, 14.49999999999999467 ) ) ;
#28303=CARTESIAN_POINT ( 'NONE',  ( 32.50000000000000000, 155.0000000000000000, -6.938893903907228378E-15 ) ) ;
#28306=CARTESIAN_POINT ( 'NONE',  ( 51.37499999726881583, 155.0000000000000000, -15.58253175000000823 ) ) ;
#28307=EDGE_CURVE ( 'NONE', #29401, #23763, #7521, .T. ) ;
#28309=CARTESIAN_POINT ( 'NONE',  ( 86.72499999726882436, 140.1801316387863778, -4.815267126137194431 ) ) ;
#28312=CARTESIAN_POINT ( 'NONE',  ( 53.79999999453763593, 146.4771138417591203, -11.73074641843674470 ) ) ;
#28323=CARTESIAN_POINT ( 'NONE',  ( 44.71132485994280614, 155.0000000000000000, 15.00000000000001243 ) ) ;
#28329=CARTESIAN_POINT ( 'NONE',  ( 40.17499999726881299, 164.1591823560292198, 12.60653300113718167 ) ) ;
#28330=ORIENTED_EDGE ( 'NONE', *, *, #9297, .F. ) ;
#28331=CARTESIAN_POINT ( 'NONE',  ( 43.82499999726881157, 168.2552932293087906, 9.630534252274372875 ) ) ;
#28334=CIRCLE ( 'NONE', #4933, 2.149999999999985256 ) ;
#28337=CARTESIAN_POINT ( 'NONE',  ( 45.27499999726880020, 149.9369285172503510, -15.58253175000000823 ) ) ;
#28342=CARTESIAN_POINT ( 'NONE',  ( 69.00000000000001421, 170.2462022514548323, -7.872454543227099337E-15 ) ) ;
#28346=CARTESIAN_POINT ( 'NONE',  ( 57.08867513459483689, 167.7597621252805880, -9.270509831248443078 ) ) ;
#28347=DIRECTION ( 'NONE',  ( -1.000000000000000000, -0.000000000000000000, -0.000000000000000000 ) ) ;
#28350=CARTESIAN_POINT ( 'NONE',  ( 68.42499999726881299, 141.7447067706911810, 9.630534252274376428 ) ) ;
#28353=CARTESIAN_POINT ( 'NONE',  ( 36.89999999453762314, 159.7113355953771077, 14.49999999999999289 ) ) ;
#28355=FACE_OUTER_BOUND ( 'NONE', #23619, .T. ) ;
#28356=ORIENTED_EDGE ( 'NONE', *, *, #19498, .T. ) ;
#28358=VECTOR ( 'NONE', #7126, 1000.000000000000000 ) ;
#28370=CARTESIAN_POINT ( 'NONE',  ( 81.11132485994279762, 140.7341522555726669, 4.635254915624211769 ) ) ;
#28373=CARTESIAN_POINT ( 'NONE',  ( 85.02499999726882152, 149.9369285172503510, -15.58253175000000823 ) ) ;
#28378=CARTESIAN_POINT ( 'NONE',  ( 49.10000000000000142, 168.7903194862797420, 4.480746418436729606 ) ) ;
#28380=CARTESIAN_POINT ( 'NONE',  ( 88.07499999726879025, 168.2552932293087906, 9.630534252274372875 ) ) ;
#28381=CARTESIAN_POINT ( 'NONE',  ( 48.22499999726880304, 149.9369285172503510, 15.58253174999999580 ) ) ;
#28385=CARTESIAN_POINT ( 'NONE',  ( 59.22499999726880304, 160.0630714827496206, -15.58253175000000823 ) ) ;
#28386=CARTESIAN_POINT ( 'NONE',  ( 68.87499999726881583, 138.6155565068815463, -3.929120461958505118E-15 ) ) ;
#28388=CARTESIAN_POINT ( 'NONE',  ( 46.41132485994281609, 167.7597621252805880, 9.270509831248428867 ) ) ;
#28402=CARTESIAN_POINT ( 'NONE',  ( 77.67499999726879878, 168.2552932293087906, -9.630534252274385310 ) ) ;
#28404=VERTEX_POINT ( 'NONE', #30695 ) ;
#28405=CARTESIAN_POINT ( 'NONE',  ( 69.12499999726881583, 155.0000000000000000, -15.58253175000000823 ) ) ;
#28406=DIRECTION ( 'NONE',  ( 1.000000000000000000, 0.000000000000000000, 0.000000000000000000 ) ) ;
#28409=CARTESIAN_POINT ( 'NONE',  ( 63.92499999726880588, 164.1591823560292198, 12.60653300113718167 ) ) ;
#28418=CARTESIAN_POINT ( 'NONE',  ( 34.71132485994281325, 155.0000000000000000, 15.00000000000001243 ) ) ;
#28426=DIRECTION ( 'NONE',  ( 1.000000000000000000, 0.000000000000000000, 0.000000000000000000 ) ) ;
#28427=CARTESIAN_POINT ( 'NONE',  ( 38.62499999726880873, 138.6155565068815747, -3.929120461958505118E-15 ) ) ;
#28435=CARTESIAN_POINT ( 'NONE',  ( 74.19999999453763451, 163.5228861582408797, -11.73074641843674470 ) ) ;
#28440=B_SPLINE_CURVE_WITH_KNOTS ( 'NONE', 3,
 ( #16032, #26422, #22141, #1698, #25045, #17201, #9030, #32531, #27427, #11931 ),
 .UNSPECIFIED., .F., .F.,
 ( 4, 2, 2, 2, 4 ),
 ( 0.000000000000000000, 0.003060558710793118489, 0.006121117421586236979, 0.009181676132379355468, 0.01224223484317247396 ),
 .UNSPECIFIED. ) ;
#28445=VERTEX_POINT ( 'NONE', #4447 ) ;
#28446=CYLINDRICAL_SURFACE ( 'NONE', #30361, 15.00000000000001776 ) ;
#28449=ORIENTED_EDGE ( 'NONE', *, *, #17414, .T. ) ;
#28453=CARTESIAN_POINT ( 'NONE',  ( 63.77499999726880731, 169.8198683612136222, -4.815267126137197984 ) ) ;
#28456=AXIS2_PLACEMENT_3D ( 'NONE', #27357, #24807, #9469 ) ;
#28459=AXIS2_PLACEMENT_3D ( 'NONE', #25117, #28015, #25291 ) ;
#28467=CARTESIAN_POINT ( 'NONE',  ( 85.39999999999999147, 159.7113355953771077, 14.49999999999999289 ) ) ;
#28471=ADVANCED_FACE ( 'NONE', ( #27611 ), #32897, .T. ) ;
#28472=CARTESIAN_POINT ( 'NONE',  ( 47.78867513459482552, 155.0000000000000000, 15.00000000000001243 ) ) ;
#28473=CARTESIAN_POINT ( 'NONE',  ( 50.27499999726880731, 160.0630714827496206, 15.58253174999999402 ) ) ;
#28480=CARTESIAN_POINT ( 'NONE',  ( 53.29999999453763593, 142.6655632788954620, 8.961492836873471646 ) ) ;
#28483=CARTESIAN_POINT ( 'NONE',  ( 47.31132485994280756, 140.7341522555726669, -4.635254915624220651 ) ) ;
#28498=CARTESIAN_POINT ( 'NONE',  ( 41.07499999726881157, 141.7447067706911810, -9.630534252274387086 ) ) ;
#28500=CARTESIAN_POINT ( 'NONE',  ( 51.12499999726881583, 155.0000000000000000, -15.58253175000000823 ) ) ;
#28501=CARTESIAN_POINT ( 'NONE',  ( 32.50000000000000000, 155.0000000000000000, -15.00000000000002487 ) ) ;
#28505=CARTESIAN_POINT ( 'NONE',  ( 47.17499999726881299, 145.8408176439707802, -12.60653300113719588 ) ) ;
#28512=CARTESIAN_POINT ( 'NONE',  ( 66.90000000000000568, 168.7903194862797420, -4.480746418436745593 ) ) ;
#28517=AXIS2_PLACEMENT_3D ( 'NONE', #28783, #13270, #12776 ) ;
#28520=CARTESIAN_POINT ( 'NONE',  ( 70.22499999726879594, 149.9369285172503510, 15.58253174999999580 ) ) ;
#28523=CARTESIAN_POINT ( 'NONE',  ( 37.29999999453762882, 142.6655632788954620, 8.961492836873471646 ) ) ;
#28526=EDGE_CURVE ( 'NONE', #31333, #20312, #7159, .T. ) ;
#28538=ORIENTED_EDGE ( 'NONE', *, *, #9725, .F. ) ;
#28545=EDGE_LOOP ( 'NONE', ( #941, #7665, #20768, #1066 ) ) ;
#28547=CARTESIAN_POINT ( 'NONE',  ( 81.32499999726880446, 164.1591823560292198, -12.60653300113719766 ) ) ;
#28552=CARTESIAN_POINT ( 'NONE',  ( 50.40000000000000568, 150.2886644046228639, -14.50000000000000888 ) ) ;
#28555=CARTESIAN_POINT ( 'NONE',  ( 53.02499999726881441, 149.9369285172503510, -15.58253175000000823 ) ) ;
#28558=CARTESIAN_POINT ( 'NONE',  ( 56.42499999726881299, 141.7447067706911810, 9.630534252274376428 ) ) ;
#28559=CARTESIAN_POINT ( 'NONE',  ( 68.27499999726879309, 160.0630714827496206, 15.58253174999999402 ) ) ;
#28561=CARTESIAN_POINT ( 'NONE',  ( 41.51132485994280330, 146.1832212156128890, -12.13525491562423042 ) ) ;
#28574=ORIENTED_EDGE ( 'NONE', *, *, #18949, .T. ) ;
#28575=CARTESIAN_POINT ( 'NONE',  ( 78.97499999726881015, 140.1801316387863778, -4.815267126137194431 ) ) ;
#28578=CARTESIAN_POINT ( 'NONE',  ( 70.72499999726881015, 140.1801316387863778, -4.815267126137194431 ) ) ;
#28581=CARTESIAN_POINT ( 'NONE',  ( 60.52499999726881441, 140.1801316387863778, 4.815267126137185549 ) ) ;
#28596=CARTESIAN_POINT ( 'NONE',  ( 36.32499999726881157, 145.8408176439707802, 12.60653300113718345 ) ) ;
#28604=CARTESIAN_POINT ( 'NONE',  ( 77.99999999453763166, 155.0000000000000000, -14.50000000000000711 ) ) ;
#28609=EDGE_CURVE ( 'NONE', #12292, #23334, #6754, .T. ) ;
#28618=CARTESIAN_POINT ( 'NONE',  ( 82.61132485994282604, 159.8737954434934920, 15.00000000000010836 ) ) ;
#28620=CARTESIAN_POINT ( 'NONE',  ( 63.47499999726881015, 160.0630714827496206, -15.58253175000000823 ) ) ;
#28626=CARTESIAN_POINT ( 'NONE',  ( 87.40513633176574615, 142.1470333418077132, -8.983655774715980868 ) ) ;
#28631=CARTESIAN_POINT ( 'NONE',  ( 84.39999999999999147, 150.2886644046228639, -14.50000000000000888 ) ) ;
#28635=CARTESIAN_POINT ( 'NONE',  ( 64.38867513459483405, 140.7341522555726669, -4.635254915624220651 ) ) ;
#28636=CARTESIAN_POINT ( 'NONE',  ( 60.27499999726880020, 160.0630714827496206, 15.58253174999999402 ) ) ;
#28641=CARTESIAN_POINT ( 'NONE',  ( 57.79999999453762882, 146.4771138417591203, -11.73074641843674470 ) ) ;
#28642=VERTEX_POINT ( 'NONE', #25573 ) ;
#28646=DIRECTION ( 'NONE',  ( 1.000000000000000000, 0.000000000000000000, 0.000000000000000000 ) ) ;
#28652=CARTESIAN_POINT ( 'NONE',  ( 79.98867513459481415, 146.1832212156128890, 12.13525491562421976 ) ) ;
#28655=VECTOR ( 'NONE', #6000, 1000.000000000000000 ) ;
#28657=CARTESIAN_POINT ( 'NONE',  ( 42.97499999726881015, 140.1801316387863778, -4.815267126137194431 ) ) ;
#28658=ORIENTED_EDGE ( 'NONE', *, *, #8864, .F. ) ;
#28659=CARTESIAN_POINT ( 'NONE',  ( 52.62499999726880162, 138.6155565068815463, -3.929120461958505118E-15 ) ) ;
#28663=CARTESIAN_POINT ( 'NONE',  ( 53.07499999726880446, 141.7447067706911810, -9.630534252274385310 ) ) ;
#28668=CARTESIAN_POINT ( 'NONE',  ( 66.40000000000000568, 150.2886644046228639, -14.50000000000000888 ) ) ;
#28670=CARTESIAN_POINT ( 'NONE',  ( 38.08867513459482268, 142.2402378747194405, 9.270509831248432420 ) ) ;
#28672=CYLINDRICAL_SURFACE ( 'NONE', #23264, 2.149999999999984812 ) ;
#28673=CARTESIAN_POINT ( 'NONE',  ( 39.07499999726881157, 141.7447067706911810, -9.630534252274385310 ) ) ;
#28675=CARTESIAN_POINT ( 'NONE',  ( 71.12499999726881583, 155.0000000000000000, -15.58253175000000823 ) ) ;
#28678=CARTESIAN_POINT ( 'NONE',  ( 86.17499999726881299, 164.1591823560292198, 12.60653300113718167 ) ) ;
#28685=CIRCLE ( 'NONE', #23237, 13.00000000000001776 ) ;
#28694=CARTESIAN_POINT ( 'NONE',  ( 73.81132485994281467, 159.8737954434934920, -15.00000000000012434 ) ) ;
#28697=VERTEX_POINT ( 'NONE', #8027 ) ;
#28702=CARTESIAN_POINT ( 'NONE',  ( 35.67499999726880588, 168.2552932293087906, -9.630534252274385310 ) ) ;
#28703=FACE_OUTER_BOUND ( 'NONE', #28002, .T. ) ;
#28707=MECHANICAL_DESIGN_GEOMETRIC_PRESENTATION_REPRESENTATION('',(#30884),#11294);
#28708=CARTESIAN_POINT ( 'NONE',  ( 46.79999999999999716, 167.3344367211045096, -8.961492836873482304 ) ) ;
#28712=( BOUNDED_CURVE ( )  B_SPLINE_CURVE ( 2, ( #23824, #3210, #13598, #23992, #655, #11056, #21437, #18879, #29273, #5924, #16318 ),
 .UNSPECIFIED., .F., .T. ) 
 B_SPLINE_CURVE_WITH_KNOTS ( ( 3, 2, 2, 2, 2, 3 ),
 ( 0.3392857142857141906, 0.3428571428571427493, 0.3464285714285713080, 0.3499999999999998668, 0.3535714285714284810, 0.3571428571428570398 ),
 .UNSPECIFIED. ) 
 CURVE ( )  GEOMETRIC_REPRESENTATION_ITEM ( )  RATIONAL_B_SPLINE_CURVE ( ( 1.000000000000001554, 0.9510565162951518658, 1.000000000000000000, 0.9510565162951534202, 1.000000000000000000, 0.9510565162951534202, 1.000000000000000000, 0.9510565162951534202, 1.000000000000000000, 0.9510565162951549745, 0.9999999999999984457 ) ) 
 REPRESENTATION_ITEM ( '' )  );
#28715=CARTESIAN_POINT ( 'NONE',  ( 48.52499999726880731, 140.1801316387863778, 4.815267126137185549 ) ) ;
#28718=CARTESIAN_POINT ( 'NONE',  ( 66.32499999726881867, 145.8408176439707802, 12.60653300113718345 ) ) ;
#28719=CARTESIAN_POINT ( 'NONE',  ( 69.17499999726881299, 145.8408176439707802, -12.60653300113719588 ) ) ;
#28721=FACE_BOUND ( 'NONE', #20261, .T. ) ;
#28738=ORIENTED_EDGE ( 'NONE', *, *, #13724, .T. ) ;
#28739=CARTESIAN_POINT ( 'NONE',  ( 75.72499999726881015, 169.8198683612136222, 4.815267126137181997 ) ) ;
#28741=CARTESIAN_POINT ( 'NONE',  ( 127.5000000000000000, 231.4735983853260279, 73.43303922622204993 ) ) ;
#28743=CARTESIAN_POINT ( 'NONE',  ( 64.12499999726881583, 155.0000000000000000, 15.58253174999999402 ) ) ;
#28748=VERTEX_POINT ( 'NONE', #24183 ) ;
#28753=FACE_BOUND ( 'NONE', #10636, .T. ) ;
#28759=CARTESIAN_POINT ( 'NONE',  ( 45.98867513459482126, 146.1832212156128890, 12.13525491562421976 ) ) ;
#28761=CARTESIAN_POINT ( 'NONE',  ( 37.22499999726881015, 160.0630714827496206, -15.58253175000000823 ) ) ;
#28767=AXIS2_PLACEMENT_3D ( 'NONE', #31284, #25656, #7270 ) ;
#28770=CARTESIAN_POINT ( 'NONE',  ( 81.99999999453763166, 155.0000000000000000, -14.50000000000000711 ) ) ;
#28783=CARTESIAN_POINT ( 'NONE',  ( 125.5000000000000000, 154.9999999999996305, -106.0000000000000142 ) ) ;
#28785=CARTESIAN_POINT ( 'NONE',  ( 82.51132485994280330, 163.8167787843871110, 12.13525491562421621 ) ) ;
#28788=CARTESIAN_POINT ( 'NONE',  ( 63.37499999726880873, 155.0000000000000000, -15.58253175000000823 ) ) ;
#28789=AXIS2_PLACEMENT_3D ( 'NONE', #27289, #3946, #26485 ) ;
#28800=CARTESIAN_POINT ( 'NONE',  ( 37.92499999726881299, 164.1591823560292198, 12.60653300113718167 ) ) ;
#28806=CARTESIAN_POINT ( 'NONE',  ( 55.07499999726879736, 141.7447067706911810, -9.630534252274385310 ) ) ;
#28811=CARTESIAN_POINT ( 'NONE',  ( 58.89999999453761603, 159.7113355953771077, 14.49999999999999289 ) ) ;
#28814=CARTESIAN_POINT ( 'NONE',  ( 37.18867513459482410, 169.2658477444273331, -4.635254915624224203 ) ) ;
#28817=CARTESIAN_POINT ( 'NONE',  ( 71.48867513459484258, 167.7597621252805880, 9.270509831248428867 ) ) ;
#28818=ORIENTED_EDGE ( 'NONE', *, *, #344, .T. ) ;
#28826=CARTESIAN_POINT ( 'NONE',  ( 44.97499999726881015, 140.1801316387863778, -4.815267126137194431 ) ) ;
#28828=CARTESIAN_POINT ( 'NONE',  ( 53.72499999726881015, 169.8198683612136222, 4.815267126137181997 ) ) ;
#28832=CARTESIAN_POINT ( 'NONE',  ( 54.67499999726881299, 141.7447067706911810, 9.630534252274376428 ) ) ;
#28835=DIRECTION ( 'NONE',  ( -1.000000000000000000, -0.000000000000000000, -0.000000000000000000 ) ) ;
#28837=CARTESIAN_POINT ( 'NONE',  ( 68.40000000000000568, 150.2886644046228639, -14.50000000000000888 ) ) ;
#28839=CARTESIAN_POINT ( 'NONE',  ( 38.38867513459481984, 140.7341522555726669, -4.635254915624220651 ) ) ;
#28842=CARTESIAN_POINT ( 'NONE',  ( 39.57499999726881157, 164.1591823560292198, -12.60653300113719766 ) ) ;
#28845=CARTESIAN_POINT ( 'NONE',  ( 69.52499999726880731, 169.8198683612136222, -4.815267126137197984 ) ) ;
#28846=VERTEX_POINT ( 'NONE', #845 ) ;
#28848=CARTESIAN_POINT ( 'NONE',  ( 42.09999999453762598, 159.7113355953771077, -14.50000000000000888 ) ) ;
#28850=CARTESIAN_POINT ( 'NONE',  ( 32.50000000000000000, 155.0000000000000000, -6.938893903907228378E-15 ) ) ;
#28854=DIRECTION ( 'NONE',  ( 0.000000000000000000, 1.000000000000000000, -1.224646799147353207E-16 ) ) ;
#28858=FACE_OUTER_BOUND ( 'NONE', #1577, .T. ) ;
#28865=CARTESIAN_POINT ( 'NONE',  ( 35.77499999726881441, 169.8198683612136222, -4.815267126137197984 ) ) ;
#28869=CARTESIAN_POINT ( 'NONE',  ( 47.89999999999999858, 141.2096805137202580, 4.480746418436733158 ) ) ;
#28871=CARTESIAN_POINT ( 'NONE',  ( 83.91132485994279477, 163.8167787843871110, -12.13525491562423397 ) ) ;
#28874=CARTESIAN_POINT ( 'NONE',  ( 48.82499999726880446, 141.7447067706911810, -9.630534252274385310 ) ) ;
#28879=CARTESIAN_POINT ( 'NONE',  ( 60.72499999726881015, 140.1801316387863778, -4.815267126137194431 ) ) ;
#28880=CARTESIAN_POINT ( 'NONE',  ( 76.17499999726881299, 164.1591823560292198, 12.60653300113718167 ) ) ;
#28884=CARTESIAN_POINT ( 'NONE',  ( 35.78867513459482552, 155.0000000000000000, 15.00000000000001243 ) ) ;
#28886=ORIENTED_EDGE ( 'NONE', *, *, #21018, .F. ) ;
#28899=EDGE_CURVE ( 'NONE', #28445, #13382, #10268, .T. ) ;
#28900=CARTESIAN_POINT ( 'NONE',  ( 76.52499999726880731, 140.1801316387863778, 4.815267126137185549 ) ) ;
#28905=CARTESIAN_POINT ( 'NONE',  ( 72.82499999726879025, 141.7447067706911810, -9.630534252274385310 ) ) ;
#28908=FACE_OUTER_BOUND ( 'NONE', #18800, .T. ) ;
#28916=CARTESIAN_POINT ( 'NONE',  ( 87.37499999726880162, 155.0000000000000000, -15.58253175000000823 ) ) ;
#28917=CARTESIAN_POINT ( 'NONE',  ( 60.08867513459482979, 142.2402378747194405, 9.270509831248432420 ) ) ;
#28918=CARTESIAN_POINT ( 'NONE',  ( 46.22499999726880304, 149.9369285172503510, 15.58253174999999580 ) ) ;
#28926=CARTESIAN_POINT ( 'NONE',  ( 82.59999999453762598, 168.7903194862797420, 4.480746418436729606 ) ) ;
#28939=CARTESIAN_POINT ( 'NONE',  ( 79.17499999726881299, 145.8408176439707802, -12.60653300113719588 ) ) ;
#28945=FILL_AREA_STYLE ('',( #500 ) ) ;
#28947=CARTESIAN_POINT ( 'NONE',  ( 60.87499999726880162, 138.6155565068815747, -3.929120461958505118E-15 ) ) ;
#28949=CARTESIAN_POINT ( 'NONE',  ( 62.08867513459483689, 142.2402378747194405, 9.270509831248432420 ) ) ;
#28954=DIRECTION ( 'NONE',  ( 0.000000000000000000, 0.000000000000000000, -1.000000000000000000 ) ) ;
#28956=CARTESIAN_POINT ( 'NONE',  ( 83.37499999726881583, 155.0000000000000000, -15.58253175000000823 ) ) ;
#28957=SHAPE_DEFINITION_REPRESENTATION ( #21913, #32415 ) ;
#28960=CARTESIAN_POINT ( 'NONE',  ( 38.62499999726880873, 138.6155565068815463, -3.929120461958505118E-15 ) ) ;
#28964=CARTESIAN_POINT ( 'NONE',  ( 57.97499999726881015, 169.8198683612136222, 4.815267126137181997 ) ) ;
#28971=CARTESIAN_POINT ( 'NONE',  ( 57.29999999453762882, 142.6655632788954620, 8.961492836873471646 ) ) ;
#28974=FACE_OUTER_BOUND ( 'NONE', #25805, .T. ) ;
#28977=CARTESIAN_POINT ( 'NONE',  ( 72.71132485994280614, 155.0000000000000000, 15.00000000000001243 ) ) ;
#28982=EDGE_CURVE ( 'NONE', #17237, #28748, #25027, .T. ) ;
#28986=CIRCLE ( 'NONE', #2872, 70.00000000000002842 ) ;
#28990=CARTESIAN_POINT ( 'NONE',  ( 42.87499999726881583, 138.6155565068815747, -3.929120461958505118E-15 ) ) ;
#28992=CARTESIAN_POINT ( 'NONE',  ( 49.52499999726880731, 169.8198683612136222, -4.815267126137197984 ) ) ;
#28996=CARTESIAN_POINT ( 'NONE',  ( 54.07499999726880446, 168.2552932293087906, 9.630534252274372875 ) ) ;
#29000=CARTESIAN_POINT ( 'NONE',  ( 71.00000000000000000, 170.2462022514548323, -7.872454543227099337E-15 ) ) ;
#29005=CARTESIAN_POINT ( 'NONE',  ( 36.87499999726881583, 138.6155565068815463, -3.929120461958505118E-15 ) ) ;
#29007=CARTESIAN_POINT ( 'NONE',  ( 78.62499999726881583, 138.6155565068815463, -3.929120461958505118E-15 ) ) ;
#29008=ORIENTED_EDGE ( 'NONE', *, *, #17060, .F. ) ;
#29009=CARTESIAN_POINT ( 'NONE',  ( 48.41132485994280898, 167.7597621252805880, 9.270509831248428867 ) ) ;
#29011=CARTESIAN_POINT ( 'NONE',  ( 41.59999999453763309, 141.2096805137202580, -4.480746418436742040 ) ) ;
#29033=CARTESIAN_POINT ( 'NONE',  ( 33.52499999726880731, 169.8198683612136222, -4.815267126137197984 ) ) ;
#29036=CARTESIAN_POINT ( 'NONE',  ( 33.97499999726881725, 169.8198683612136222, 4.815267126137181997 ) ) ;
#29040=CARTESIAN_POINT ( 'NONE',  ( 57.19999999999999574, 167.3344367211045096, 8.961492836873468093 ) ) ;
#29043=CARTESIAN_POINT ( 'NONE',  ( 52.42499999726880588, 141.7447067706911810, 9.630534252274376428 ) ) ;
#29045=CARTESIAN_POINT ( 'NONE',  ( 125.5000000000000000, 81.56696077377658582, -76.47359838532473475 ) ) ;
#29046=CARTESIAN_POINT ( 'NONE',  ( 63.02499999726882152, 149.9369285172503510, -15.58253175000000823 ) ) ;
#29047=CARTESIAN_POINT ( 'NONE',  ( 75.87499999726881583, 171.3844434931184253, -7.942151717890132712E-15 ) ) ;
#29058=CARTESIAN_POINT ( 'NONE',  ( 33.78867513459482552, 155.0000000000000000, 15.00000000000001243 ) ) ;
#29060=VECTOR ( 'NONE', #865, 1000.000000000000000 ) ;
#29064=ORIENTED_EDGE ( 'NONE', *, *, #31661, .F. ) ;
#29066=ORIENTED_EDGE ( 'NONE', *, *, #8695, .F. ) ;
#29068=CARTESIAN_POINT ( 'NONE',  ( 80.12499999726881583, 155.0000000000000000, 15.58253174999999402 ) ) ;
#29069=DIRECTION ( 'NONE',  ( 1.000000000000000000, 0.000000000000000000, 0.000000000000000000 ) ) ;
#29073=CARTESIAN_POINT ( 'NONE',  ( 67.52499999726880731, 169.8198683612136222, -4.815267126137197984 ) ) ;
#29083=CARTESIAN_POINT ( 'NONE',  ( 63.78867513459482552, 155.0000000000000000, 15.00000000000001243 ) ) ;
#29089=CARTESIAN_POINT ( 'NONE',  ( 41.62499999726880162, 171.3844434931184253, -7.942151717890134290E-15 ) ) ;
#29091=CARTESIAN_POINT ( 'NONE',  ( 72.71132485994280614, 155.0000000000000000, 15.00000000000001243 ) ) ;
#29096=CARTESIAN_POINT ( 'NONE',  ( 79.99999999453763166, 155.0000000000000000, -14.50000000000000711 ) ) ;
#29099=EDGE_CURVE ( 'NONE', #7343, #9970, #3893, .T. ) ;
#29107=CARTESIAN_POINT ( 'NONE',  ( 77.77499999726880731, 169.8198683612136222, -4.815267126137197984 ) ) ;
#29112=CARTESIAN_POINT ( 'NONE',  ( 65.07499999726881867, 141.7447067706911810, -9.630534252274387086 ) ) ;
#29114=CARTESIAN_POINT ( 'NONE',  ( 67.88867513459483405, 150.1262045565062238, 14.99999999999987388 ) ) ;
#29116=CARTESIAN_POINT ( 'NONE',  ( 43.68867513459482410, 159.8737954434936057, 15.00000000000001421 ) ) ;
#29119=CARTESIAN_POINT ( 'NONE',  ( 80.51132485994280330, 163.8167787843871110, 12.13525491562421621 ) ) ;
#29122=CARTESIAN_POINT ( 'NONE',  ( 83.47499999726881015, 160.0630714827496206, -15.58253175000000823 ) ) ;
#29125=CARTESIAN_POINT ( 'NONE',  ( 39.92499999726881299, 164.1591823560292198, 12.60653300113718167 ) ) ;
#29126=CYLINDRICAL_SURFACE ( 'NONE', #13075, 2.149999999999984812 ) ;
#29128=CARTESIAN_POINT ( 'NONE',  ( 82.18867513459483121, 140.7341522555726669, 4.635254915624211769 ) ) ;
#29129=CARTESIAN_POINT ( 'NONE',  ( 54.57499999726881157, 145.8408176439707802, 12.60653300113718345 ) ) ;
#29136=CARTESIAN_POINT ( 'NONE',  ( 62.69999999453762740, 167.3344367211045096, 8.961492836873468093 ) ) ;
#29142=CARTESIAN_POINT ( 'NONE',  ( 71.71132485994280614, 155.0000000000000000, -15.00000000000002487 ) ) ;
#29147=DIRECTION ( 'NONE',  ( 1.000000000000000000, 0.000000000000000000, 0.000000000000000000 ) ) ;
#29150=DIRECTION ( 'NONE',  ( 1.000000000000000000, 0.000000000000000000, 0.000000000000000000 ) ) ;
#29152=CARTESIAN_POINT ( 'NONE',  ( 46.77499999726881441, 140.1801316387863778, 4.815267126137185549 ) ) ;
#29154=CARTESIAN_POINT ( 'NONE',  ( 50.42499999726880588, 141.7447067706911810, 9.630534252274376428 ) ) ;
#29156=CARTESIAN_POINT ( 'NONE',  ( 61.08867513459484400, 167.7597621252805880, -9.270509831248443078 ) ) ;
#29158=CARTESIAN_POINT ( 'NONE',  ( 54.97499999726881015, 140.1801316387863778, -4.815267126137194431 ) ) ;
#29165=CARTESIAN_POINT ( 'NONE',  ( 72.80000000000001137, 167.3344367211045096, -8.961492836873482304 ) ) ;
#29170=ADVANCED_FACE ( 'NONE', ( #23479 ), #4917, .T. ) ;
#29171=CARTESIAN_POINT ( 'NONE',  ( 34.97499999726881015, 140.1801316387863778, -4.815267126137194431 ) ) ;
#29175=CARTESIAN_POINT ( 'NONE',  ( 79.82499999726881867, 168.2552932293087906, 9.630534252274372875 ) ) ;
#29178=CARTESIAN_POINT ( 'NONE',  ( 40.99999999453763166, 155.0000000000000000, 14.49999999999999467 ) ) ;
#29192=ORIENTED_EDGE ( 'NONE', *, *, #11675, .F. ) ;
#29195=DIRECTION ( 'NONE',  ( 1.000000000000000000, 0.000000000000000000, 0.000000000000000000 ) ) ;
#29198=CARTESIAN_POINT ( 'NONE',  ( 33.72499999726881725, 169.8198683612136222, 4.815267126137181997 ) ) ;
#29199=CARTESIAN_POINT ( 'NONE',  ( 34.07499999726879736, 168.2552932293087906, 9.630534252274372875 ) ) ;
#29203=CARTESIAN_POINT ( 'NONE',  ( 54.90000000000000568, 168.7903194862797420, -4.480746418436745593 ) ) ;
#29205=CARTESIAN_POINT ( 'NONE',  ( 77.18867513459481700, 169.2658477444273331, -4.635254915624224203 ) ) ;
#29207=CARTESIAN_POINT ( 'NONE',  ( 55.92499999726881299, 164.1591823560292198, 12.60653300113718167 ) ) ;
#29208=VECTOR ( 'NONE', #27100, 1000.000000000000000 ) ;
#29211=CARTESIAN_POINT ( 'NONE',  ( 60.62499999726880162, 138.6155565068815747, -3.929120461958505118E-15 ) ) ;
#29212=CARTESIAN_POINT ( 'NONE',  ( 75.67499999726881299, 168.2552932293087906, -9.630534252274385310 ) ) ;
#29233=CARTESIAN_POINT ( 'NONE',  ( 77.32499999726881867, 164.1591823560292198, -12.60653300113719766 ) ) ;
#29234=ORIENTED_EDGE ( 'NONE', *, *, #12713, .T. ) ;
#29238=CARTESIAN_POINT ( 'NONE',  ( 68.32499999726881867, 145.8408176439707802, 12.60653300113718345 ) ) ;
#29241=CIRCLE ( 'NONE', #10750, 112.0000000000000711 ) ;
#29244=CARTESIAN_POINT ( 'NONE',  ( 35.50000000000000711, 155.0000000000000000, 14.49999999999999467 ) ) ;
#29252=CARTESIAN_POINT ( 'NONE',  ( 46.72499999726881015, 140.1801316387863778, -4.815267126137194431 ) ) ;
#29261=CARTESIAN_POINT ( 'NONE',  ( 77.09999999453762598, 150.2886644046228639, 14.49999999999999645 ) ) ;
#29265=CARTESIAN_POINT ( 'NONE',  ( 49.48867513459482126, 167.7597621252805880, 9.270509831248428867 ) ) ;
#29272=CARTESIAN_POINT ( 'NONE',  ( 74.17499999726881299, 164.1591823560292198, 12.60653300113718167 ) ) ;
#29273=CARTESIAN_POINT ( 'NONE',  ( 53.51132485994281041, 146.1832212156128890, -12.13525491562423042 ) ) ;
#29280=CARTESIAN_POINT ( 'NONE',  ( 69.97499999726881015, 169.8198683612136222, 4.815267126137181997 ) ) ;
#29282=CARTESIAN_POINT ( 'NONE',  ( 40.88867513459481984, 159.8737954434936057, -15.00000000000002665 ) ) ;
#29286=CARTESIAN_POINT ( 'NONE',  ( 83.38867513459483405, 169.2658477444273331, 4.635254915624208216 ) ) ;
#29288=CARTESIAN_POINT ( 'NONE',  ( 86.17499999726881299, 164.1591823560292198, 12.60653300113718167 ) ) ;
#29292=CARTESIAN_POINT ( 'NONE',  ( 36.62499999726881583, 138.6155565068815463, -3.929120461958505118E-15 ) ) ;
#29293=CARTESIAN_POINT ( 'NONE',  ( 35.71132485994280614, 155.0000000000000000, -15.00000000000002487 ) ) ;
#29294=CARTESIAN_POINT ( 'NONE',  ( 49.78867513459482552, 155.0000000000000000, 15.00000000000001243 ) ) ;
#29297=CARTESIAN_POINT ( 'NONE',  ( 54.67499999726881299, 141.7447067706911810, 9.630534252274376428 ) ) ;
#29304=CARTESIAN_POINT ( 'NONE',  ( 57.59999999453763309, 141.2096805137202580, -4.480746418436742040 ) ) ;
#29310=AXIS2_PLACEMENT_3D ( 'NONE', #18681, #29069, #5721 ) ;
#29311=CARTESIAN_POINT ( 'NONE',  ( 36.78867513459482552, 155.0000000000000000, -15.00000000000002487 ) ) ;
#29317=AXIS2_PLACEMENT_3D ( 'NONE', #26090, #31040, #197 ) ;
#29323=DIRECTION ( 'NONE',  ( 1.000000000000000000, 0.000000000000000000, 0.000000000000000000 ) ) ;
#29325=CARTESIAN_POINT ( 'NONE',  ( 47.57499999726881867, 164.1591823560292198, -12.60653300113719766 ) ) ;
#29327=CARTESIAN_POINT ( 'NONE',  ( 54.62499999726880162, 138.6155565068815463, -3.929120461958505118E-15 ) ) ;
#29329=CARTESIAN_POINT ( 'NONE',  ( 61.38867513459481984, 169.2658477444273331, 4.635254915624208216 ) ) ;
#29333=EDGE_CURVE ( 'NONE', #8954, #15366, #10380, .T. ) ;
#29334=CARTESIAN_POINT ( 'NONE',  ( 51.47499999726881725, 160.0630714827496206, -15.58253175000000823 ) ) ;
#29339=CARTESIAN_POINT ( 'NONE',  ( 73.50000000000001421, 155.0000000000000000, 14.49999999999999467 ) ) ;
#29343=CARTESIAN_POINT ( 'NONE',  ( 32.50000000000000000, 155.0000000000000000, -6.938893903907228378E-15 ) ) ;
#29344=CARTESIAN_POINT ( 'NONE',  ( 38.77499999726881441, 140.1801316387863778, 4.815267126137185549 ) ) ;
#29346=CARTESIAN_POINT ( 'NONE',  ( 74.92499999726881299, 145.8408176439707802, -12.60653300113719588 ) ) ;
#29347=ORIENTED_EDGE ( 'NONE', *, *, #32690, .T. ) ;
#29348=CARTESIAN_POINT ( 'NONE',  ( 51.78867513459482552, 155.0000000000000000, 15.00000000000001243 ) ) ;
#29349=CARTESIAN_POINT ( 'NONE',  ( 40.59999999453763309, 168.7903194862797420, 4.480746418436729606 ) ) ;
#29363=CARTESIAN_POINT ( 'NONE',  ( 50.48867513459482836, 142.2402378747194405, -9.270509831248439525 ) ) ;
#29364=VERTEX_POINT ( 'NONE', #29091 ) ;
#29369=ORIENTED_EDGE ( 'NONE', *, *, #24714, .T. ) ;
#29373=CARTESIAN_POINT ( 'NONE',  ( 35.07499999726881157, 141.7447067706911810, -9.630534252274385310 ) ) ;
#29376=CARTESIAN_POINT ( 'NONE',  ( 52.90000000000000568, 168.7903194862797420, -4.480746418436745593 ) ) ;
#29379=CARTESIAN_POINT ( 'NONE',  ( 59.92499999726881299, 164.1591823560292198, 12.60653300113718167 ) ) ;
#29382=CARTESIAN_POINT ( 'NONE',  ( 63.72499999726881015, 169.8198683612136222, 4.815267126137181997 ) ) ;
#29383=CARTESIAN_POINT ( 'NONE',  ( 74.37499999726881583, 155.0000000000000000, 15.58253174999999402 ) ) ;
#29386=CARTESIAN_POINT ( 'NONE',  ( 84.68867513459485963, 150.1262045565065364, -15.00000000000013323 ) ) ;
#29387=EDGE_CURVE ( 'NONE', #7672, #31619, #3352, .T. ) ;
#29398=VERTEX_POINT ( 'NONE', #636 ) ;
#29401=VERTEX_POINT ( 'NONE', #29419 ) ;
#29402=CARTESIAN_POINT ( 'NONE',  ( 75.22499999726879594, 160.0630714827496206, -15.58253175000000823 ) ) ;
#29404=DIRECTION ( 'NONE',  ( 0.000000000000000000, 0.7071067811865442421, -0.7071067811865506814 ) ) ;
#29405=CARTESIAN_POINT ( 'NONE',  ( 73.12499999726881583, 155.0000000000000000, -15.58253175000000823 ) ) ;
#29409=CARTESIAN_POINT ( 'NONE',  ( 33.10000000000000142, 168.7903194862797420, 4.480746418436729606 ) ) ;
#29417=CARTESIAN_POINT ( 'NONE',  ( 47.72499999726881015, 169.8198683612136222, 4.815267126137181997 ) ) ;
#29419=CARTESIAN_POINT ( 'NONE',  ( 125.5000000000000000, 261.0000000000000000, -2.149999999999985256 ) ) ;
#29425=CARTESIAN_POINT ( 'NONE',  ( 84.79999999453762882, 163.5228861582408797, 11.73074641843673049 ) ) ;
#29429=DIRECTION ( 'NONE',  ( 0.000000000000000000, 0.000000000000000000, -1.000000000000000000 ) ) ;
#29433=ORIENTED_EDGE ( 'NONE', *, *, #31666, .T. ) ;
#29436=CARTESIAN_POINT ( 'NONE',  ( 78.37499999726883004, 155.0000000000000000, 15.58253174999999402 ) ) ;
#29441=EDGE_CURVE ( 'NONE', #17245, #24797, #3688, .T. ) ;
#29443=CARTESIAN_POINT ( 'NONE',  ( 71.77499999726882152, 169.8198683612136222, -4.815267126137197984 ) ) ;
#29444=VERTEX_POINT ( 'NONE', #5906 ) ;
#29445=CARTESIAN_POINT ( 'NONE',  ( 127.5000000000000000, 78.52640161467553526, 73.43303922622362734 ) ) ;
#29450=CARTESIAN_POINT ( 'NONE',  ( 82.78867513459482552, 155.0000000000000000, -15.00000000000002487 ) ) ;
#29452=CARTESIAN_POINT ( 'NONE',  ( 83.67499999726884141, 168.2552932293087906, -9.630534252274385310 ) ) ;
#29455=CARTESIAN_POINT ( 'NONE',  ( 39.52499999726881441, 169.8198683612136222, -4.815267126137197984 ) ) ;
#29457=FACE_OUTER_BOUND ( 'NONE', #10851, .T. ) ;
#29460=CARTESIAN_POINT ( 'NONE',  ( 63.37499999726880873, 155.0000000000000000, -15.58253175000000823 ) ) ;
#29467=CARTESIAN_POINT ( 'NONE',  ( 65.69999999453763451, 142.6655632788954620, -8.961492836873480528 ) ) ;
#29472=DIRECTION ( 'NONE',  ( 0.000000000000000000, 0.000000000000000000, -1.000000000000000000 ) ) ;
#29476=EDGE_LOOP ( 'NONE', ( #20267, #4611, #11585, #12599 ) ) ;
#29484=CARTESIAN_POINT ( 'NONE',  ( 49.97499999726881725, 169.8198683612136222, 4.815267126137181997 ) ) ;
#29486=CARTESIAN_POINT ( 'NONE',  ( 56.62499999726880162, 138.6155565068815463, -3.929120461958505118E-15 ) ) ;
#29488=CARTESIAN_POINT ( 'NONE',  ( 61.28867513459483263, 170.7719333635740497, -7.904646289410545231E-15 ) ) ;
#29493=CARTESIAN_POINT ( 'NONE',  ( 57.27499999726882152, 149.9369285172503510, -15.58253175000000823 ) ) ;
#29495=CARTESIAN_POINT ( 'NONE',  ( 73.78867513459483973, 155.0000000000000000, 15.00000000000001243 ) ) ;
#29498=CARTESIAN_POINT ( 'NONE',  ( 71.39999999999999147, 159.7113355953771077, 14.49999999999999289 ) ) ;
#29502=FACE_OUTER_BOUND ( 'NONE', #12731, .T. ) ;
#29503=CARTESIAN_POINT ( 'NONE',  ( 46.37499999726880873, 155.0000000000000000, 15.58253174999999402 ) ) ;
#29505=CARTESIAN_POINT ( 'NONE',  ( 76.02499999726880731, 160.0630714827496206, 15.58253174999999402 ) ) ;
#29508=CARTESIAN_POINT ( 'NONE',  ( 47.91132485994280188, 163.8167787843871110, -12.13525491562423397 ) ) ;
#29509=CARTESIAN_POINT ( 'NONE',  ( 42.89999999453763024, 159.7113355953771077, 14.49999999999999289 ) ) ;
#29517=CARTESIAN_POINT ( 'NONE',  ( 61.78867513459482552, 155.0000000000000000, 15.00000000000001243 ) ) ;
#29519=ADVANCED_FACE ( 'NONE', ( #32976 ), #15700, .F. ) ;
#29524=DIRECTION ( 'NONE',  ( -1.000000000000000000, -0.000000000000000000, -0.000000000000000000 ) ) ;
#29531=CARTESIAN_POINT ( 'NONE',  ( 40.12499999726880873, 155.0000000000000000, 15.58253174999999402 ) ) ;
#29534=CARTESIAN_POINT ( 'NONE',  ( 40.17499999726881299, 164.1591823560292198, 12.60653300113718167 ) ) ;
#29535=CARTESIAN_POINT ( 'NONE',  ( 125.5000000000000000, 154.9999999999996305, -106.0000000000000142 ) ) ;
#29537=VECTOR ( 'NONE', #32465, 1000.000000000000000 ) ;
#29538=CARTESIAN_POINT ( 'NONE',  ( 55.00000000000000711, 170.2462022514548323, -7.872454543227099337E-15 ) ) ;
#29540=CARTESIAN_POINT ( 'NONE',  ( 77.68867513459484542, 159.8737954434933215, 15.00000000000024336 ) ) ;
#29544=CARTESIAN_POINT ( 'NONE',  ( 56.92499999726881299, 145.8408176439707802, -12.60653300113719588 ) ) ;
#29546=CARTESIAN_POINT ( 'NONE',  ( 37.01132485994280330, 142.2402378747194405, 9.270509831248432420 ) ) ;
#29547=CARTESIAN_POINT ( 'NONE',  ( 67.92499999726881299, 164.1591823560292198, 12.60653300113718167 ) ) ;
#29548=CARTESIAN_POINT ( 'NONE',  ( 75.07499999726879025, 141.7447067706911810, -9.630534252274385310 ) ) ;
#29552=CARTESIAN_POINT ( 'NONE',  ( 53.58867513459482268, 163.8167787843871110, 12.13525491562421621 ) ) ;
#29561=ADVANCED_FACE ( 'NONE', ( #19697 ), #20037, .T. ) ;
#29563=EDGE_LOOP ( 'NONE', ( #6488, #3171, #24357, #15453 ) ) ;
#29564=CARTESIAN_POINT ( 'NONE',  ( 39.71132485994280614, 155.0000000000000000, -15.00000000000002487 ) ) ;
#29566=ORIENTED_EDGE ( 'NONE', *, *, #10125, .F. ) ;
#29572=CARTESIAN_POINT ( 'NONE',  ( 85.52499999726880731, 169.8198683612136222, -4.815267126137197984 ) ) ;
#29575=CARTESIAN_POINT ( 'NONE',  ( 68.52499999726880731, 140.1801316387863778, 4.815267126137185549 ) ) ;
#29580=CARTESIAN_POINT ( 'NONE',  ( 33.89999999999999858, 141.2096805137202580, 4.480746418436733158 ) ) ;
#29589=AXIS2_PLACEMENT_3D ( 'NONE', #2896, #30854, #28954 ) ;
#29591=CARTESIAN_POINT ( 'NONE',  ( 45.52499999726881441, 169.8198683612136222, -4.815267126137197984 ) ) ;
#29600=CARTESIAN_POINT ( 'NONE',  ( 88.69999999453763451, 167.3344367211045096, 8.961492836873468093 ) ) ;
#29603=( BOUNDED_CURVE ( )  B_SPLINE_CURVE ( 2, ( #14232, #16950, #1295, #24800, #6225, #17130, #27516, #25124, #6740, #11686, #4174 ),
 .UNSPECIFIED., .F., .T. ) 
 B_SPLINE_CURVE_WITH_KNOTS ( ( 3, 2, 2, 2, 2, 3 ),
 ( 0.6249999999999998890, 0.6285714285714284477, 0.6321428571428570065, 0.6357142857142855652, 0.6392857142857141239, 0.6428571428571427937 ),
 .UNSPECIFIED. ) 
 CURVE ( )  GEOMETRIC_REPRESENTATION_ITEM ( )  RATIONAL_B_SPLINE_CURVE ( ( 1.000000000000001554, 0.9510565162951518658, 1.000000000000000000, 0.9510565162951534202, 1.000000000000000000, 0.9510565162951534202, 1.000000000000000000, 0.9510565162951534202, 1.000000000000000000, 0.9510565162951549745, 0.9999999999999984457 ) ) 
 REPRESENTATION_ITEM ( '' )  );
#29605=CARTESIAN_POINT ( 'NONE',  ( 32.50000000000000000, 155.0000000000000000, -6.938893903907228378E-15 ) ) ;
#29610=CARTESIAN_POINT ( 'NONE',  ( 73.07499999726880446, 141.7447067706911810, -9.630534252274385310 ) ) ;
#29613=CARTESIAN_POINT ( 'NONE',  ( 78.27499999726880731, 160.0630714827496206, 15.58253174999999224 ) ) ;
#29617=( NAMED_UNIT ( * ) PLANE_ANGLE_UNIT ( ) SI_UNIT ( $, .RADIAN. ) );
#29619=CARTESIAN_POINT ( 'NONE',  ( 69.27499999726880731, 149.9369285172503510, -15.58253175000000823 ) ) ;
#29621=CARTESIAN_POINT ( 'NONE',  ( 61.78867513459482552, 155.0000000000000000, 15.00000000000001243 ) ) ;
#29627=CARTESIAN_POINT ( 'NONE',  ( 85.17499999726882720, 145.8408176439707802, -12.60653300113719588 ) ) ;
#29631=CARTESIAN_POINT ( 'NONE',  ( 42.92499999726881299, 145.8408176439707802, -12.60653300113719588 ) ) ;
#29639=CARTESIAN_POINT ( 'NONE',  ( 77.78867513459483973, 155.0000000000000000, 15.00000000000001243 ) ) ;
#29642=CARTESIAN_POINT ( 'NONE',  ( 66.29999999453762882, 167.3344367211045096, -8.961492836873482304 ) ) ;
#29648=DIRECTION ( 'NONE',  ( 0.000000000000000000, 0.000000000000000000, -1.000000000000000000 ) ) ;
#29658=CARTESIAN_POINT ( 'NONE',  ( 51.67499999726879878, 168.2552932293087906, -9.630534252274387086 ) ) ;
#29659=ORIENTED_EDGE ( 'NONE', *, *, #16996, .T. ) ;
#29660=CARTESIAN_POINT ( 'NONE',  ( 57.92499999726881299, 164.1591823560292198, 12.60653300113718167 ) ) ;
#29662=CARTESIAN_POINT ( 'NONE',  ( 61.18867513459481700, 169.2658477444273331, -4.635254915624224203 ) ) ;
#29665=CARTESIAN_POINT ( 'NONE',  ( 58.87499999726880162, 138.6155565068815463, -3.929120461958505118E-15 ) ) ;
#29669=CARTESIAN_POINT ( 'NONE',  ( 73.70000000000000284, 146.4771138417591203, 11.73074641843673227 ) ) ;
#29670=CARTESIAN_POINT ( 'NONE',  ( 40.68867513459483121, 150.1262045565064227, -15.00000000000002665 ) ) ;
#29671=DIRECTION ( 'NONE',  ( -1.000000000000000000, -0.000000000000000000, -0.000000000000000000 ) ) ;
#29674=CARTESIAN_POINT ( 'NONE',  ( 46.07499999726881157, 168.2552932293087906, 9.630534252274372875 ) ) ;
#29676=CARTESIAN_POINT ( 'NONE',  ( 76.22499999726882436, 149.9369285172503510, 15.58253174999999580 ) ) ;
#29679=CARTESIAN_POINT ( 'NONE',  ( 49.09999999453761887, 150.2886644046228639, 14.49999999999999645 ) ) ;
#29681=DIRECTION ( 'NONE',  ( 0.000000000000000000, 0.000000000000000000, -1.000000000000000000 ) ) ;
#29690=CARTESIAN_POINT ( 'NONE',  ( 50.68867513459483121, 150.1262045565064227, -15.00000000000002665 ) ) ;
#29691=ORIENTED_EDGE ( 'NONE', *, *, #23274, .T. ) ;
#29697=CARTESIAN_POINT ( 'NONE',  ( 39.82499999726880446, 168.2552932293087906, 9.630534252274372875 ) ) ;
#29699=CARTESIAN_POINT ( 'NONE',  ( 42.37499999726881583, 155.0000000000000000, 15.58253174999999402 ) ) ;
#29702=CARTESIAN_POINT ( 'NONE',  ( 53.00000000000000711, 170.2462022514548323, -7.872454543227099337E-15 ) ) ;
#29708=CARTESIAN_POINT ( 'NONE',  ( 59.12499999726881583, 155.0000000000000000, -15.58253175000000823 ) ) ;
#29712=CARTESIAN_POINT ( 'NONE',  ( 82.67499999726879878, 141.7447067706911810, 9.630534252274376428 ) ) ;
#29715=EDGE_CURVE ( 'NONE', #14095, #8954, #23082, .T. ) ;
#29724=CARTESIAN_POINT ( 'NONE',  ( 127.5000000000000000, 155.0000000000000000, -98.00000000000002842 ) ) ;
#29729=EDGE_CURVE ( 'NONE', #7343, #8868, #31539, .T. ) ;
#29730=CARTESIAN_POINT ( 'NONE',  ( 39.21132485994281325, 139.2280666364260071, -4.041636747397287284E-15 ) ) ;
#29735=CARTESIAN_POINT ( 'NONE',  ( 83.72499999726882436, 169.8198683612136222, 4.815267126137181997 ) ) ;
#29738=CARTESIAN_POINT ( 'NONE',  ( 73.42499999726881299, 168.2552932293087906, -9.630534252274385310 ) ) ;
#29743=AXIS2_PLACEMENT_3D ( 'NONE', #32734, #27623, #19801 ) ;
#29745=CARTESIAN_POINT ( 'NONE',  ( 35.80000000000000426, 142.6655632788954620, 8.961492836873471646 ) ) ;
#29753=CARTESIAN_POINT ( 'NONE',  ( 32.50000000000000000, 155.0000000000000000, -15.00000000000002487 ) ) ;
#29754=CARTESIAN_POINT ( 'NONE',  ( 52.92499999726881299, 145.8408176439707802, -12.60653300113719588 ) ) ;
#29756=CARTESIAN_POINT ( 'NONE',  ( 41.11132485994280472, 140.7341522555726669, 4.635254915624211769 ) ) ;
#29761=CARTESIAN_POINT ( 'NONE',  ( 87.79999999453764303, 146.4771138417591203, -11.73074641843674470 ) ) ;
#29768=ORIENTED_EDGE ( 'NONE', *, *, #822, .T. ) ;
#29771=CARTESIAN_POINT ( 'NONE',  ( 74.27499999726880731, 160.0630714827496206, 15.58253174999999402 ) ) ;
#29776=CARTESIAN_POINT ( 'NONE',  ( 80.37499999726881583, 155.0000000000000000, 15.58253174999999402 ) ) ;
#29778=CARTESIAN_POINT ( 'NONE',  ( 127.5000000000000000, 229.9533188057739039, -74.95331880577418815 ) ) ;
#29784=CARTESIAN_POINT ( 'NONE',  ( 66.57499999726881867, 145.8408176439707802, 12.60653300113718345 ) ) ;
#29785=ORIENTED_EDGE ( 'NONE', *, *, #1015, .T. ) ;
#29786=DIRECTION ( 'NONE',  ( 1.000000000000000000, 0.000000000000000000, 0.000000000000000000 ) ) ;
#29787=CARTESIAN_POINT ( 'NONE',  ( 52.58867513459482268, 146.1832212156128890, -12.13525491562423042 ) ) ;
#29791=ADVANCED_FACE ( 'NONE', ( #23271 ), #33494, .T. ) ;
#29799=CARTESIAN_POINT ( 'NONE',  ( 47.32499999726881867, 164.1591823560292198, -12.60653300113719766 ) ) ;
#29804=( BOUNDED_SURFACE ( )  B_SPLINE_SURFACE ( 1, 2, ( 
 ( #31911, #15910, #8253, #26307, #29033, #18310, #29198, #2978, #13357, #8583, #23751, #2650, #5361, #415, #10818, #23917, #10976, #4133, #14525, #27308, #13859, #24925, #9419, #6186, #11975, #1584, #24244, #30035, #29873, #19473, #6532, #22195, #11647, #3969, #16912, #19307, #11807, #32584, #32247, #911, #1086, #24762, #8914, #14368, #24590, #22360, #16745, #3462, #9252, #19646, #22031, #32749, #19814, #32412, #6700, #1416, #17090, #27476, #11309, #16405, #9079, #30207, #26798, #21694, #16577, #32086, #8748, #29697, #26968, #19137, #29531, #3630, #11478, #14023, #6355, #24422, #21856, #27146, #3806, #14195, #1249, #25087, #33267, #20147, #33608, #2439, #17943, #10110, #30892, #27807, #2100, #30543, #20317, #14695, #12647, #23042, #23213, #7381, #20488, #4814, #22707, #7040, #9934, #7206, #17760, #17592, #7556, #28331, #6864, #22876, #2265, #20666, #33095, #14863, #12144, #4989, #25259, #1925, #10287, #1745, #12487, #9764, #17422, #15376, #27983, #28158, #15034, #17253, #32924, #22539, #27640, #15208, #4650, #9583, #30721, #25768, #25426, #25599, #4474, #33438, #12820, #4309, #12311, #19977, #30378, #31711, #18605, #2608, #52, #21315, #12994, #26109, #13483, #3093, #23875, #547, #31225, #31549, #23711, #706, #16039, #31060, #5484, #10939, #28992, #5651, #26268, #8217, #3256, #8383, #18771, #26430, #2936, #29154, #24038, #13319, #5805, #16202, #26591, #13644, #28500, #7719, #372, #11108, #18105, #5153, #20822, #15541, #23388, #10614, #7889, #25933, #10448, #18270, #15707, #28659, #23548, #5318, #2777, #13156, #217, #20989, #31385, #8056, #10776, #18439, #28828, #15873, #21151, #25166, #12224, #8708, #16704, #1045, #1201, #29327, #27728, #4387, #4563, #21988, #1833, #19430, #3590, #21650, #24547, #21814, #32374, #11437, #22612, #9667, #21487, #3766, #17338, #2006, #13983, #29486, #26757, #32999, #6142, #16535, #14950, #16363, #27105, #24380, #32045, #20060, #8869, #9038, #29660, #31871, #13816, #3421, #8536, #29834, #32206, #24209, #14151, #30459, #19267, #6309, #19098, #6948, #11600, #25337, #26932, #14773, #7119, #17500, #27888, #872, #11268, #18932, #5975, #7460, #28581, #18188, #5231, #15618, #12564, #12901, #5067, #15788, #31133, #12396, #20572, #26022, #32588, #20737, #7635, #23297, #18351, #2695, #4899, #10363, #30976, #31304, #12738, #33183, #22956, #7798, #15461, #26179, #13071, #22791, #18018, #23462, #128, #10529, #28409, #20909, #28743, #7967, #15285, #5403, #25854, #9846, #23127, #20228, #30628, #7297, #2515, #17676, #28063, #4725, #15115, #25510, #2179, #33352, #10025, #20405, #30799, #17843, #28243, #25680, #2348, #33515, #10191, #16112, #3011, #16615, #23629, #952, #21232, #10686, #29073, #26350, #13899, #291, #13392, #3337, #23791, #21068, #29238, #26507, #29575, #32121, #24279, #6055, #26843, #460, #31788, #3177, #16286, #31470, #8621, #19017, #19180, #13722, #16447, #792, #18683, #10859, #5889, #13568, #24121, #23958, #3506, #11350, #2848, #18843, #31952, #13233, #5723, #31627, #8137, #21732, #8296, #620, #6227, #18521, #8455, #11019, #21399, #8785, #26675, #11181, #21559, #28905, #5561, #15953, #29405, #27517, #6569, #29738, #19683, #4351, #24801, #4014, #24633, #24971, #16952, #20023, #27187, #11688, #25126, #27688, #14570, #32295, #6404, #17301, #8956, #22070, #9464, #32793, #19851, #30248, #3842, #14735, #1789, #4175, #24462, #12189, #30424, #16786, #22578, #32963, #1124, #6908, #6741, #30077, #17131, #9626, #22238, #1624, #12015, #29916, #22401, #7082, #9122, #11517, #32453, #27011, #19520, #3672, #32628, #14065, #11853, #27348, #19345, #21898, #14234, #14408, #1457, #1297, #9289, #22918, #14911, #22753, #2144, #30762, #12862, #4521, #12529, #28202, #20189, #25302, #31099, #10148, #90, #7419, #4861, #1966, #28547, #12357, #2308, #17638, #13034, #15249, #33146, #30935, #25471, #9980, #2651, #20700, #9809, #23254, #20367, #30588, #20529, #15578, #7253, #4689, #17981, #7599, #33479, #28024, #15075, #17805, #25642, #33310, #12694, #23427, #25978, #33648, #7760, #23090, #10328, #10490, #18152, #28373, #5193, #20870, #17464, #5030, #15420, #31269, #25817, #2480, #27848, #26310, #21194, #5851, #26802, #8099, #7930, #23918, #260, #8585, #21524, #23753, #583, #31589, #10977, #5362, #13683, #5521, #8254, #18981, #10820, #913, #16408 ),
 ( #11312, #2813, #3140, #417, #18482, #6017, #29036, #29199, #16078, #18311, #10655, #13195, #21697, #8420, #18643, #21029, #21355, #29373, #5689, #26470, #15912, #16250, #13526, #28702, #28865, #2979, #3466, #13861, #26636, #23595, #31429, #31913, #13358, #31752, #24081, #750, #11149, #24246, #18806, #3298, #15750, #26145, #17097, #32088, #6535, #24930, #19650, #6705, #27311, #9256, #4314, #11979, #24593, #30040, #16915, #17257, #32417, #19139, #14529, #27481, #3973, #30212, #25091, #14374, #22364, #32590, #4137, #1589, #29534, #8751, #24765, #32753, #6191, #9424, #21859, #14699, #3632, #11651, #32250, #12148, #16579, #6869, #16748, #26970, #1254, #8919, #19818, #14026, #19310, #27645, #29699, #24425, #1420, #22034, #1749, #1089, #11480, #6357, #27150, #3808, #11812, #9082, #22200, #14197, #19478, #29878, #5157, #23049, #25774, #20493, #4654, #22711, #25604, #22880, #33443, #2105, #12491, #15212, #19982, #28337, #20150, #33271, #33612, #25430, #15545, #31065, #25937, #1929, #14867, #33100, #10291, #20670, #10114, #30383, #7723, #2612, #12316, #18109, #28505, #7044, #2445, #2269, #12651, #30896, #4993, #17765, #7561, #17947, #9939, #15380, #12825, #15038, #17427, #7210, #23216, #17597, #22544, #28162, #32928, #7385, #20323, #25264, #9587, #9768, #27988, #30725, #27811, #4478, #4819, #30548, #18274, #31390, #26272, #8387, #56, #8060, #23716, #15712, #20826, #26597, #5656, #29334, #2941, #377, #10452, #24043, #31231, #31553, #13161, #8542, #10780, #7893, #26434, #20993, #5489, #31876, #16208, #28663, #18775, #15878, #5322, #16043, #11114, #26113, #223, #13487, #3099, #28996, #2781, #10619, #13324, #21156, #18444, #28832, #18937, #21492, #29158, #3261, #8221, #5811, #5980, #13650, #18610, #711, #16369, #12998, #23552, #23880, #26763, #551, #21319, #23392, #10944, #31715, #1379, #22326, #3595, #3426, #19435, #29493, #4096, #17047, #19272, #29839, #11767, #26937, #19775, #8714, #16709, #13989, #17213, #24214, #1547, #21821, #11274, #29665, #24385, #14486, #877, #1051, #3930, #11442, #21655, #6499, #27111, #30171, #32714, #24886, #6660, #27443, #32211, #32380, #3773, #16877, #32051, #9220, #19609, #6829, #14328, #11945, #22157, #6315, #8875, #27272, #14157, #24723, #24553, #9381, #13822, #19104, #32545, #30001, #6147, #1210, #11605, #16541, #21995, #9043, #25223, #17901, #12109, #4617, #12273, #30337, #33404, #7170, #20279, #17555, #27601, #19939, #32887, #4269, #30685, #20113, #7003, #12449, #10076, #14999, #27947, #14826, #7348, #30505, #14662, #27772, #22665, #7517, #20454, #17728, #17389, #4437, #30852, #1888, #33054, #2227, #15170, #12610, #23007, #9722, #28114, #22838, #25056, #25563, #1710, #33230, #28295, #4775, #4949, #9896, #22500, #9547, #25387, #2060, #1490, #32486, #9491, #24663, #11382, #6772, #19711, #29943, #22433, #17331, #6599, #14605, #24826, #11885, #27542, #21761, #24315, #16981, #25000, #985, #4207, #24490, #22270, #27377, #27721, #9320, #32151, #9154, #17156, #32655, #30108, #19549, #1651, #30275, #12046, #16818, #32825, #4043, #19879, #1326, #8811, #6941, #4381, #14433, #19211, #29610, #6258, #16644, #27044, #3707, #14096, #1152, #11544, #21929, #32322, #8988, #19375, #29771, #6437, #27214, #3870, #14262, #11714, #22099, #12893, #33175, #22605, #7288, #4555, #25848, #12217, #14943, #15279, #25330, #32992, #7452, #28056, #7791, #10356, #2509, #18011, #5061, #1997, #10017, #4716, #28236, #9660, #20564, #30968, #31127, #25673, #28402, #12732, #30620, #12387, #17834, #15108, #2342, #25502, #15454, #23289, #14764, #30791, #10181, #28575, #17668, #22784, #20053, #33682, #9840, #20221, #18182, #30452, #20398, #2172, #12557, #20730, #22949, #23121, #33345, #25157, #7113, #17493, #1824, #33508, #4892, #27879, #7628, #7109, #31517, #19232, #8347, #32007, #27064, #18736, #3224, #21612, #8830, #23839, #23678, #5940, #16007, #24336, #3557, #5770, #16331, #13611, #13947, #28956, #29122, #6102, #29452, #16499, #26898, #513, #24176, #26723, #3727, #8671, #337, #31837, #1007, #11227, #19064, #18893, #838, #29627, #11403, #16163, #21780, #8502, #6276, #24006, #10737, #32170, #16668, #29288, #21119, #8187, #3385, #18571, #5615, #26399, #3057, #13445, #10906, #13780, #21283, #31677, #26554, #669, #11072, #21453, #27397, #14281, #28380, #1168, #12701, #32506 ) ),
 .UNSPECIFIED., .F., .F., .T. ) 
 B_SPLINE_SURFACE_WITH_KNOTS ( ( 2, 2 ),
 ( 3, 2, 2, 2, 2, 2, 2, 2, 2, 2, 2, 2, 2, 2, 2, 2, 2, 2, 2, 2, 2, 2, 2, 2, 2, 2, 2, 2, 2, 2, 2, 2, 2, 2, 2, 2, 2, 2, 2, 2, 2, 2, 2, 2, 2, 2, 2, 2, 2, 2, 2, 2, 2, 2, 2, 2, 2, 2, 2, 2, 2, 2, 2, 2, 2, 2, 2, 2, 2, 2, 2, 2, 2, 2, 2, 2, 2, 2, 2, 2, 2, 2, 2, 2, 2, 2, 2, 2, 2, 2, 2, 2, 2, 2, 2, 2, 2, 2, 2, 2, 2, 2, 2, 2, 2, 2, 2, 2, 2, 2, 2, 2, 2, 2, 2, 2, 2, 2, 2, 2, 2, 2, 2, 2, 2, 2, 2, 2, 2, 2, 2, 2, 2, 2, 2, 2, 2, 2, 2, 2, 2, 2, 2, 2, 2, 2, 2, 2, 2, 2, 2, 2, 2, 2, 2, 2, 2, 2, 2, 2, 2, 2, 2, 2, 2, 2, 2, 2, 2, 2, 2, 2, 2, 2, 2, 2, 2, 2, 2, 2, 2, 2, 2, 2, 2, 2, 2, 2, 2, 2, 2, 2, 2, 2, 2, 2, 2, 2, 2, 2, 2, 2, 2, 2, 2, 2, 2, 2, 2, 2, 2, 2, 2, 2, 2, 2, 2, 2, 2, 2, 2, 2, 2, 2, 2, 2, 2, 2, 2, 2, 2, 2, 2, 2, 2, 2, 2, 2, 2, 2, 2, 2, 2, 2, 2, 2, 2, 2, 2, 2, 2, 2, 2, 2, 2, 2, 2, 2, 2, 2, 2, 2, 2, 2, 2, 2, 2, 2, 2, 2, 2, 2, 2, 2, 2, 3 ),
 ( 0.000000000000000000, 1.000000000000000000 ),
 ( 0.000000000000000000, 0.003571428571428571317, 0.007142857142857142634, 0.01071428571428571438, 0.01428571428571428527, 0.01785714285714285615, 0.02142857142857142877, 0.02500000000000000139, 0.02857142857142857054, 0.03214285714285713969, 0.03571428571428571230, 0.03928571428571428492, 0.04285714285714285754, 0.04642857142857143016, 0.05000000000000000278, 0.05357142857142856845, 0.05714285714285714107, 0.06071428571428571369, 0.06428571428571427937, 0.06785714285714285199, 0.07142857142857142461, 0.07499999999999999722, 0.07857142857142856984, 0.08214285714285714246, 0.08571428571428571508, 0.08928571428571428770, 0.09285714285714286031, 0.09642857142857143293, 0.1000000000000000056, 0.1035714285714285782, 0.1071428571428571369, 0.1107142857142857095, 0.1142857142857142821, 0.1178571428571428548, 0.1214285714285714274, 0.1250000000000000000, 0.1285714285714285587, 0.1321428571428571452, 0.1357142857142857040, 0.1392857142857142905, 0.1428571428571428492, 0.1464285714285714357, 0.1499999999999999944, 0.1535714285714285809, 0.1571428571428571397, 0.1607142857142857262, 0.1642857142857142849, 0.1678571428571428437, 0.1714285714285714302, 0.1749999999999999889, 0.1785714285714285754, 0.1821428571428571341, 0.1857142857142857206, 0.1892857142857142794, 0.1928571428571428659, 0.1964285714285714246, 0.2000000000000000111, 0.2035714285714285698, 0.2071428571428571563, 0.2107142857142857151, 0.2142857142857142738, 0.2178571428571428603, 0.2214285714285714191, 0.2250000000000000056, 0.2285714285714285643, 0.2321428571428571508, 0.2357142857142857095, 0.2392857142857142960, 0.2428571428571428548, 0.2464285714285714413, 0.2500000000000000000, 0.2535714285714285587, 0.2571428571428571175, 0.2607142857142857317, 0.2642857142857142905, 0.2678571428571428492, 0.2714285714285714080, 0.2750000000000000222, 0.2785714285714285809, 0.2821428571428571397, 0.2857142857142856984, 0.2892857142857143127, 0.2928571428571428714, 0.2964285714285714302, 0.2999999999999999889, 0.3035714285714285476, 0.3071428571428571619, 0.3107142857142857206, 0.3142857142857142794, 0.3178571428571428381, 0.3214285714285714524, 0.3250000000000000111, 0.3285714285714285698, 0.3321428571428571286, 0.3357142857142856873, 0.3392857142857143016, 0.3428571428571428603, 0.3464285714285714191, 0.3499999999999999778, 0.3535714285714285920, 0.3571428571428571508, 0.3607142857142857095, 0.3642857142857142683, 0.3678571428571428825, 0.3714285714285714413, 0.3750000000000000000, 0.3785714285714285587, 0.3821428571428571175, 0.3857142857142857317, 0.3892857142857142905, 0.3928571428571428492, 0.3964285714285714080, 0.4000000000000000222, 0.4035714285714285809, 0.4071428571428571397, 0.4107142857142856984, 0.4142857142857143127, 0.4178571428571428714, 0.4214285714285714302, 0.4249999999999999889, 0.4285714285714285476, 0.4321428571428571619, 0.4357142857142857206, 0.4392857142857142794, 0.4428571428571428381, 0.4464285714285714524, 0.4500000000000000111, 0.4535714285714285698, 0.4571428571428571286, 0.4607142857142856873, 0.4642857142857143016, 0.4678571428571428603, 0.4714285714285714191, 0.4749999999999999778, 0.4785714285714285920, 0.4821428571428571508, 0.4857142857142857095, 0.4892857142857142683, 0.4928571428571428825, 0.4964285714285714413, 0.5000000000000000000, 0.5035714285714285587, 0.5071428571428571175, 0.5107142857142856762, 0.5142857142857142350, 0.5178571428571429047, 0.5214285714285714635, 0.5250000000000000222, 0.5285714285714285809, 0.5321428571428571397, 0.5357142857142856984, 0.5392857142857142572, 0.5428571428571428159, 0.5464285714285713746, 0.5500000000000000444, 0.5535714285714286031, 0.5571428571428571619, 0.5607142857142857206, 0.5642857142857142794, 0.5678571428571428381, 0.5714285714285713969, 0.5749999999999999556, 0.5785714285714286254, 0.5821428571428571841, 0.5857142857142857428, 0.5892857142857143016, 0.5928571428571428603, 0.5964285714285714191, 0.5999999999999999778, 0.6035714285714285365, 0.6071428571428570953, 0.6107142857142857650, 0.6142857142857143238, 0.6178571428571428825, 0.6214285714285714413, 0.6250000000000000000, 0.6285714285714285587, 0.6321428571428571175, 0.6357142857142856762, 0.6392857142857142350, 0.6428571428571429047, 0.6464285714285714635, 0.6500000000000000222, 0.6535714285714285809, 0.6571428571428571397, 0.6607142857142856984, 0.6642857142857142572, 0.6678571428571428159, 0.6714285714285713746, 0.6750000000000000444, 0.6785714285714286031, 0.6821428571428571619, 0.6857142857142857206, 0.6892857142857142794, 0.6928571428571428381, 0.6964285714285713969, 0.6999999999999999556, 0.7035714285714286254, 0.7071428571428571841, 0.7107142857142857428, 0.7142857142857143016, 0.7178571428571428603, 0.7214285714285714191, 0.7249999999999999778, 0.7285714285714285365, 0.7321428571428570953, 0.7357142857142857650, 0.7392857142857143238, 0.7428571428571428825, 0.7464285714285714413, 0.7500000000000000000, 0.7535714285714285587, 0.7571428571428571175, 0.7607142857142856762, 0.7642857142857142350, 0.7678571428571429047, 0.7714285714285714635, 0.7750000000000000222, 0.7785714285714285809, 0.7821428571428571397, 0.7857142857142856984, 0.7892857142857142572, 0.7928571428571428159, 0.7964285714285713746, 0.8000000000000000444, 0.8035714285714286031, 0.8071428571428571619, 0.8107142857142857206, 0.8142857142857142794, 0.8178571428571428381, 0.8214285714285713969, 0.8249999999999999556, 0.8285714285714286254, 0.8321428571428571841, 0.8357142857142857428, 0.8392857142857143016, 0.8428571428571428603, 0.8464285714285714191, 0.8499999999999999778, 0.8535714285714285365, 0.8571428571428570953, 0.8607142857142857650, 0.8642857142857143238, 0.8678571428571428825, 0.8714285714285714413, 0.8750000000000000000, 0.8785714285714285587, 0.8821428571428571175, 0.8857142857142856762, 0.8892857142857142350, 0.8928571428571429047, 0.8964285714285714635, 0.9000000000000000222, 0.9035714285714285809, 0.9071428571428571397, 0.9107142857142856984, 0.9142857142857142572, 0.9178571428571428159, 0.9214285714285713746, 0.9250000000000000444, 0.9285714285714286031, 0.9321428571428571619, 0.9357142857142857206, 0.9392857142857142794, 0.9428571428571428381, 0.9464285714285713969, 0.9499999999999999556, 0.9535714285714286254, 0.9571428571428571841, 0.9607142857142857428, 0.9642857142857143016, 0.9678571428571428603, 0.9714285714285714191, 0.9749999999999999778, 0.9785714285714285365, 0.9821428571428570953 ),
 .UNSPECIFIED. ) 
 GEOMETRIC_REPRESENTATION_ITEM ( )  RATIONAL_B_SPLINE_SURFACE ( (
 ( 1.000000000000000000, 0.9510565162951535312, 1.000000000000000000, 0.9510565162951535312, 1.000000000000000000, 0.9510565162951535312, 1.000000000000000000, 0.9510565162951535312, 1.000000000000000000, 0.9510565162951535312, 1.000000000000000000, 0.9510565162951535312, 1.000000000000000000, 0.9510565162951535312, 1.000000000000000000, 0.9510565162951535312, 1.000000000000000000, 0.9510565162951535312, 1.000000000000000000, 0.9510565162951535312, 1.000000000000000000, 0.9510565162951535312, 1.000000000000000000, 0.9510565162951535312, 1.000000000000000000, 0.9510565162951535312, 1.000000000000000000, 0.9510565162951535312, 1.000000000000000000, 0.9510565162951535312, 1.000000000000000000, 0.9510565162951535312, 1.000000000000000000, 0.9510565162951535312, 1.000000000000000000, 0.9510565162951535312, 1.000000000000000000, 0.9510565162951535312, 1.000000000000000000, 0.9510565162951535312, 1.000000000000000000, 0.9510565162951535312, 1.000000000000000000, 0.9510565162951535312, 1.000000000000000000, 0.9510565162951535312, 1.000000000000000000, 0.9510565162951535312, 1.000000000000000000, 0.9510565162951535312, 1.000000000000000000, 0.9510565162951535312, 1.000000000000000000, 0.9510565162951535312, 1.000000000000000000, 0.9510565162951535312, 1.000000000000000000, 0.9510565162951535312, 1.000000000000000000, 0.9510565162951535312, 1.000000000000000000, 0.9510565162951535312, 1.000000000000000000, 0.9510565162951535312, 1.000000000000000000, 0.9510565162951535312, 1.000000000000000000, 0.9510565162951535312, 1.000000000000000000, 0.9510565162951535312, 1.000000000000000000, 0.9510565162951535312, 1.000000000000000000, 0.9510565162951535312, 1.000000000000000000, 0.9510565162951535312, 1.000000000000000000, 0.9510565162951535312, 1.000000000000000000, 0.9510565162951535312, 1.000000000000000000, 0.9510565162951535312, 1.000000000000000000, 0.9510565162951535312, 1.000000000000000000, 0.9510565162951535312, 1.000000000000000000, 0.9510565162951535312, 1.000000000000000000, 0.9510565162951535312, 1.000000000000000000, 0.9510565162951535312, 1.000000000000000000, 0.9510565162951535312, 1.000000000000000000, 0.9510565162951535312, 1.000000000000000000, 0.9510565162951535312, 1.000000000000000000, 0.9510565162951535312, 1.000000000000000000, 0.9510565162951535312, 1.000000000000000000, 0.9510565162951535312, 1.000000000000000000, 0.9510565162951535312, 1.000000000000000000, 0.9510565162951535312, 1.000000000000000000, 0.9510565162951535312, 1.000000000000000000, 0.9510565162951535312, 1.000000000000000000, 0.9510565162951535312, 1.000000000000000000, 0.9510565162951535312, 1.000000000000000000, 0.9510565162951535312, 1.000000000000000000, 0.9510565162951535312, 1.000000000000000000, 0.9510565162951535312, 1.000000000000000000, 0.9510565162951535312, 1.000000000000000000, 0.9510565162951535312, 1.000000000000000000, 0.9510565162951535312, 1.000000000000000000, 0.9510565162951535312, 1.000000000000000000, 0.9510565162951535312, 1.000000000000000000, 0.9510565162951535312, 1.000000000000000000, 0.9510565162951535312, 1.000000000000000000, 0.9510565162951535312, 1.000000000000000000, 0.9510565162951535312, 1.000000000000000000, 0.9510565162951535312, 1.000000000000000000, 0.9510565162951535312, 1.000000000000000000, 0.9510565162951535312, 1.000000000000000000, 0.9510565162951535312, 1.000000000000000000, 0.9510565162951535312, 1.000000000000000000, 0.9510565162951535312, 1.000000000000000000, 0.9510565162951535312, 1.000000000000000000, 0.9510565162951535312, 1.000000000000000000, 0.9510565162951535312, 1.000000000000000000, 0.9510565162951535312, 1.000000000000000000, 0.9510565162951535312, 1.000000000000000000, 0.9510565162951535312, 1.000000000000000000, 0.9510565162951535312, 1.000000000000000000, 0.9510565162951535312, 1.000000000000000000, 0.9510565162951535312, 1.000000000000000000, 0.9510565162951535312, 1.000000000000000000, 0.9510565162951535312, 1.000000000000000000, 0.9510565162951535312, 1.000000000000000000, 0.9510565162951535312, 1.000000000000000000, 0.9510565162951535312, 1.000000000000000000, 0.9510565162951535312, 1.000000000000000000, 0.9510565162951535312, 1.000000000000000000, 0.9510565162951535312, 1.000000000000000000, 0.9510565162951535312, 1.000000000000000000, 0.9510565162951535312, 1.000000000000000000, 0.9510565162951535312, 1.000000000000000000, 0.9510565162951535312, 1.000000000000000000, 0.9510565162951535312, 1.000000000000000000, 0.9510565162951535312, 1.000000000000000000, 0.9510565162951535312, 1.000000000000000000, 0.9510565162951535312, 1.000000000000000000, 0.9510565162951535312, 1.000000000000000000, 0.9510565162951535312, 1.000000000000000000, 0.9510565162951535312, 1.000000000000000000, 0.9510565162951535312, 1.000000000000000000, 0.9510565162951535312, 1.000000000000000000, 0.9510565162951535312, 1.000000000000000000, 0.9510565162951535312, 1.000000000000000000, 0.9510565162951535312, 1.000000000000000000, 0.9510565162951535312, 1.000000000000000000, 0.9510565162951535312, 1.000000000000000000, 0.9510565162951535312, 1.000000000000000000, 0.9510565162951535312, 1.000000000000000000, 0.9510565162951535312, 1.000000000000000000, 0.9510565162951535312, 1.000000000000000000, 0.9510565162951535312, 1.000000000000000000, 0.9510565162951535312, 1.000000000000000000, 0.9510565162951535312, 1.000000000000000000, 0.9510565162951535312, 1.000000000000000000, 0.9510565162951535312, 1.000000000000000000, 0.9510565162951535312, 1.000000000000000000, 0.9510565162951535312, 1.000000000000000000, 0.9510565162951535312, 1.000000000000000000, 0.9510565162951535312, 1.000000000000000000, 0.9510565162951535312, 1.000000000000000000, 0.9510565162951535312, 1.000000000000000000, 0.9510565162951535312, 1.000000000000000000, 0.9510565162951535312, 1.000000000000000000, 0.9510565162951535312, 1.000000000000000000, 0.9510565162951535312, 1.000000000000000000, 0.9510565162951535312, 1.000000000000000000, 0.9510565162951535312, 1.000000000000000000, 0.9510565162951535312, 1.000000000000000000, 0.9510565162951535312, 1.000000000000000000, 0.9510565162951535312, 1.000000000000000000, 0.9510565162951535312, 1.000000000000000000, 0.9510565162951535312, 1.000000000000000000, 0.9510565162951535312, 1.000000000000000000, 0.9510565162951535312, 1.000000000000000000, 0.9510565162951535312, 1.000000000000000000, 0.9510565162951535312, 1.000000000000000000, 0.9510565162951535312, 1.000000000000000000, 0.9510565162951535312, 1.000000000000000000, 0.9510565162951535312, 1.000000000000000000, 0.9510565162951535312, 1.000000000000000000, 0.9510565162951535312, 1.000000000000000000, 0.9510565162951535312, 1.000000000000000000, 0.9510565162951535312, 1.000000000000000000, 0.9510565162951535312, 1.000000000000000000, 0.9510565162951535312, 1.000000000000000000, 0.9510565162951535312, 1.000000000000000000, 0.9510565162951535312, 1.000000000000000000, 0.9510565162951535312, 1.000000000000000000, 0.9510565162951535312, 1.000000000000000000, 0.9510565162951535312, 1.000000000000000000, 0.9510565162951535312, 1.000000000000000000, 0.9510565162951535312, 1.000000000000000000, 0.9510565162951535312, 1.000000000000000000, 0.9510565162951535312, 1.000000000000000000, 0.9510565162951535312, 1.000000000000000000, 0.9510565162951535312, 1.000000000000000000, 0.9510565162951535312, 1.000000000000000000, 0.9510565162951535312, 1.000000000000000000, 0.9510565162951535312, 1.000000000000000000, 0.9510565162951535312, 1.000000000000000000, 0.9510565162951535312, 1.000000000000000000, 0.9510565162951535312, 1.000000000000000000, 0.9510565162951535312, 1.000000000000000000, 0.9510565162951535312, 1.000000000000000000, 0.9510565162951535312, 1.000000000000000000, 0.9510565162951535312, 1.000000000000000000, 0.9510565162951535312, 1.000000000000000000, 0.9510565162951535312, 1.000000000000000000, 0.9510565162951535312, 1.000000000000000000, 0.9510565162951535312, 1.000000000000000000, 0.9510565162951535312, 1.000000000000000000, 0.9510565162951535312, 1.000000000000000000, 0.9510565162951535312, 1.000000000000000000, 0.9510565162951535312, 1.000000000000000000, 0.9510565162951535312, 1.000000000000000000, 0.9510565162951535312, 1.000000000000000000, 0.9510565162951535312, 1.000000000000000000, 0.9510565162951535312, 1.000000000000000000, 0.9510565162951535312, 1.000000000000000000, 0.9510565162951535312, 1.000000000000000000, 0.9510565162951535312, 1.000000000000000000, 0.9510565162951535312, 1.000000000000000000, 0.9510565162951535312, 1.000000000000000000, 0.9510565162951535312, 1.000000000000000000, 0.9510565162951535312, 1.000000000000000000, 0.9510565162951535312, 1.000000000000000000, 0.9510565162951535312, 1.000000000000000000, 0.9510565162951535312, 1.000000000000000000, 0.9510565162951535312, 1.000000000000000000, 0.9510565162951535312, 1.000000000000000000, 0.9510565162951535312, 1.000000000000000000, 0.9510565162951535312, 1.000000000000000000, 0.9510565162951535312, 1.000000000000000000, 0.9510565162951535312, 1.000000000000000000, 0.9510565162951535312, 1.000000000000000000, 0.9510565162951535312, 1.000000000000000000, 0.9510565162951535312, 1.000000000000000000, 0.9510565162951535312, 1.000000000000000000, 0.9510565162951535312, 1.000000000000000000, 0.9510565162951535312, 1.000000000000000000, 0.9510565162951535312, 1.000000000000000000, 0.9510565162951535312, 1.000000000000000000, 0.9510565162951535312, 1.000000000000000000, 0.9510565162951535312, 1.000000000000000000, 0.9510565162951535312, 1.000000000000000000, 0.9510565162951535312, 1.000000000000000000, 0.9510565162951535312, 1.000000000000000000, 0.9510565162951535312, 1.000000000000000000, 0.9510565162951535312, 1.000000000000000000, 0.9510565162951535312, 1.000000000000000000, 0.9510565162951535312, 1.000000000000000000, 0.9510565162951535312, 1.000000000000000000, 0.9510565162951535312, 1.000000000000000000, 0.9510565162951535312, 1.000000000000000000, 0.9510565162951535312, 1.000000000000000000, 0.9510565162951535312, 1.000000000000000000, 0.9510565162951535312, 1.000000000000000000, 0.9510565162951535312, 1.000000000000000000, 0.9510565162951535312, 1.000000000000000000, 0.9510565162951535312, 1.000000000000000000, 0.9510565162951535312, 1.000000000000000000, 0.9510565162951535312, 1.000000000000000000, 0.9510565162951535312, 1.000000000000000000, 0.9510565162951535312, 1.000000000000000000, 0.9510565162951535312, 1.000000000000000000, 0.9510565162951535312, 1.000000000000000000, 0.9510565162951535312, 1.000000000000000000, 0.9510565162951535312, 1.000000000000000000, 0.9510565162951535312, 1.000000000000000000, 0.9510565162951535312, 1.000000000000000000, 0.9510565162951535312, 1.000000000000000000, 0.9510565162951535312, 1.000000000000000000, 0.9510565162951535312, 1.000000000000000000, 0.9510565162951535312, 1.000000000000000000, 0.9510565162951535312, 1.000000000000000000, 0.9510565162951535312, 1.000000000000000000, 0.9510565162951535312, 1.000000000000000000, 0.9510565162951535312, 1.000000000000000000, 0.9510565162951535312, 1.000000000000000000, 0.9510565162951535312, 1.000000000000000000, 0.9510565162951535312, 1.000000000000000000, 0.9510565162951535312, 1.000000000000000000, 0.9510565162951535312, 1.000000000000000000, 0.9510565162951535312, 1.000000000000000000, 0.9510565162951535312, 1.000000000000000000, 0.9510565162951535312, 1.000000000000000000, 0.9510565162951535312, 1.000000000000000000, 0.9510565162951535312, 1.000000000000000000, 0.9510565162951535312, 1.000000000000000000, 0.9510565162951535312, 1.000000000000000000, 0.9510565162951535312, 1.000000000000000000, 0.9510565162951535312, 1.000000000000000000, 0.9510565162951535312, 1.000000000000000000, 0.9510565162951535312, 1.000000000000000000, 0.9510565162951535312, 1.000000000000000000, 0.9510565162951535312, 1.000000000000000000, 0.9510565162951535312, 1.000000000000000000, 0.9510565162951535312, 1.000000000000000000, 0.9510565162951535312, 1.000000000000000000, 0.9510565162951535312, 1.000000000000000000, 0.9510565162951535312, 1.000000000000000000, 0.9510565162951535312, 1.000000000000000000, 0.9510565162951535312, 1.000000000000000000, 0.9510565162951535312, 1.000000000000000000, 0.9510565162951535312, 1.000000000000000000, 0.9510565162951535312, 1.000000000000000000, 0.9510565162951535312, 1.000000000000000000, 0.9510565162951535312, 1.000000000000000000, 0.9510565162951535312, 1.000000000000000000, 0.9510565162951535312, 1.000000000000000000),
 ( 1.000000000000000000, 0.9510565162951535312, 1.000000000000000000, 0.9510565162951535312, 1.000000000000000000, 0.9510565162951535312, 1.000000000000000000, 0.9510565162951535312, 1.000000000000000000, 0.9510565162951535312, 1.000000000000000000, 0.9510565162951535312, 1.000000000000000000, 0.9510565162951535312, 1.000000000000000000, 0.9510565162951535312, 1.000000000000000000, 0.9510565162951535312, 1.000000000000000000, 0.9510565162951535312, 1.000000000000000000, 0.9510565162951535312, 1.000000000000000000, 0.9510565162951535312, 1.000000000000000000, 0.9510565162951535312, 1.000000000000000000, 0.9510565162951535312, 1.000000000000000000, 0.9510565162951535312, 1.000000000000000000, 0.9510565162951535312, 1.000000000000000000, 0.9510565162951535312, 1.000000000000000000, 0.9510565162951535312, 1.000000000000000000, 0.9510565162951535312, 1.000000000000000000, 0.9510565162951535312, 1.000000000000000000, 0.9510565162951535312, 1.000000000000000000, 0.9510565162951535312, 1.000000000000000000, 0.9510565162951535312, 1.000000000000000000, 0.9510565162951535312, 1.000000000000000000, 0.9510565162951535312, 1.000000000000000000, 0.9510565162951535312, 1.000000000000000000, 0.9510565162951535312, 1.000000000000000000, 0.9510565162951535312, 1.000000000000000000, 0.9510565162951535312, 1.000000000000000000, 0.9510565162951535312, 1.000000000000000000, 0.9510565162951535312, 1.000000000000000000, 0.9510565162951535312, 1.000000000000000000, 0.9510565162951535312, 1.000000000000000000, 0.9510565162951535312, 1.000000000000000000, 0.9510565162951535312, 1.000000000000000000, 0.9510565162951535312, 1.000000000000000000, 0.9510565162951535312, 1.000000000000000000, 0.9510565162951535312, 1.000000000000000000, 0.9510565162951535312, 1.000000000000000000, 0.9510565162951535312, 1.000000000000000000, 0.9510565162951535312, 1.000000000000000000, 0.9510565162951535312, 1.000000000000000000, 0.9510565162951535312, 1.000000000000000000, 0.9510565162951535312, 1.000000000000000000, 0.9510565162951535312, 1.000000000000000000, 0.9510565162951535312, 1.000000000000000000, 0.9510565162951535312, 1.000000000000000000, 0.9510565162951535312, 1.000000000000000000, 0.9510565162951535312, 1.000000000000000000, 0.9510565162951535312, 1.000000000000000000, 0.9510565162951535312, 1.000000000000000000, 0.9510565162951535312, 1.000000000000000000, 0.9510565162951535312, 1.000000000000000000, 0.9510565162951535312, 1.000000000000000000, 0.9510565162951535312, 1.000000000000000000, 0.9510565162951535312, 1.000000000000000000, 0.9510565162951535312, 1.000000000000000000, 0.9510565162951535312, 1.000000000000000000, 0.9510565162951535312, 1.000000000000000000, 0.9510565162951535312, 1.000000000000000000, 0.9510565162951535312, 1.000000000000000000, 0.9510565162951535312, 1.000000000000000000, 0.9510565162951535312, 1.000000000000000000, 0.9510565162951535312, 1.000000000000000000, 0.9510565162951535312, 1.000000000000000000, 0.9510565162951535312, 1.000000000000000000, 0.9510565162951535312, 1.000000000000000000, 0.9510565162951535312, 1.000000000000000000, 0.9510565162951535312, 1.000000000000000000, 0.9510565162951535312, 1.000000000000000000, 0.9510565162951535312, 1.000000000000000000, 0.9510565162951535312, 1.000000000000000000, 0.9510565162951535312, 1.000000000000000000, 0.9510565162951535312, 1.000000000000000000, 0.9510565162951535312, 1.000000000000000000, 0.9510565162951535312, 1.000000000000000000, 0.9510565162951535312, 1.000000000000000000, 0.9510565162951535312, 1.000000000000000000, 0.9510565162951535312, 1.000000000000000000, 0.9510565162951535312, 1.000000000000000000, 0.9510565162951535312, 1.000000000000000000, 0.9510565162951535312, 1.000000000000000000, 0.9510565162951535312, 1.000000000000000000, 0.9510565162951535312, 1.000000000000000000, 0.9510565162951535312, 1.000000000000000000, 0.9510565162951535312, 1.000000000000000000, 0.9510565162951535312, 1.000000000000000000, 0.9510565162951535312, 1.000000000000000000, 0.9510565162951535312, 1.000000000000000000, 0.9510565162951535312, 1.000000000000000000, 0.9510565162951535312, 1.000000000000000000, 0.9510565162951535312, 1.000000000000000000, 0.9510565162951535312, 1.000000000000000000, 0.9510565162951535312, 1.000000000000000000, 0.9510565162951535312, 1.000000000000000000, 0.9510565162951535312, 1.000000000000000000, 0.9510565162951535312, 1.000000000000000000, 0.9510565162951535312, 1.000000000000000000, 0.9510565162951535312, 1.000000000000000000, 0.9510565162951535312, 1.000000000000000000, 0.9510565162951535312, 1.000000000000000000, 0.9510565162951535312, 1.000000000000000000, 0.9510565162951535312, 1.000000000000000000, 0.9510565162951535312, 1.000000000000000000, 0.9510565162951535312, 1.000000000000000000, 0.9510565162951535312, 1.000000000000000000, 0.9510565162951535312, 1.000000000000000000, 0.9510565162951535312, 1.000000000000000000, 0.9510565162951535312, 1.000000000000000000, 0.9510565162951535312, 1.000000000000000000, 0.9510565162951535312, 1.000000000000000000, 0.9510565162951535312, 1.000000000000000000, 0.9510565162951535312, 1.000000000000000000, 0.9510565162951535312, 1.000000000000000000, 0.9510565162951535312, 1.000000000000000000, 0.9510565162951535312, 1.000000000000000000, 0.9510565162951535312, 1.000000000000000000, 0.9510565162951535312, 1.000000000000000000, 0.9510565162951535312, 1.000000000000000000, 0.9510565162951535312, 1.000000000000000000, 0.9510565162951535312, 1.000000000000000000, 0.9510565162951535312, 1.000000000000000000, 0.9510565162951535312, 1.000000000000000000, 0.9510565162951535312, 1.000000000000000000, 0.9510565162951535312, 1.000000000000000000, 0.9510565162951535312, 1.000000000000000000, 0.9510565162951535312, 1.000000000000000000, 0.9510565162951535312, 1.000000000000000000, 0.9510565162951535312, 1.000000000000000000, 0.9510565162951535312, 1.000000000000000000, 0.9510565162951535312, 1.000000000000000000, 0.9510565162951535312, 1.000000000000000000, 0.9510565162951535312, 1.000000000000000000, 0.9510565162951535312, 1.000000000000000000, 0.9510565162951535312, 1.000000000000000000, 0.9510565162951535312, 1.000000000000000000, 0.9510565162951535312, 1.000000000000000000, 0.9510565162951535312, 1.000000000000000000, 0.9510565162951535312, 1.000000000000000000, 0.9510565162951535312, 1.000000000000000000, 0.9510565162951535312, 1.000000000000000000, 0.9510565162951535312, 1.000000000000000000, 0.9510565162951535312, 1.000000000000000000, 0.9510565162951535312, 1.000000000000000000, 0.9510565162951535312, 1.000000000000000000, 0.9510565162951535312, 1.000000000000000000, 0.9510565162951535312, 1.000000000000000000, 0.9510565162951535312, 1.000000000000000000, 0.9510565162951535312, 1.000000000000000000, 0.9510565162951535312, 1.000000000000000000, 0.9510565162951535312, 1.000000000000000000, 0.9510565162951535312, 1.000000000000000000, 0.9510565162951535312, 1.000000000000000000, 0.9510565162951535312, 1.000000000000000000, 0.9510565162951535312, 1.000000000000000000, 0.9510565162951535312, 1.000000000000000000, 0.9510565162951535312, 1.000000000000000000, 0.9510565162951535312, 1.000000000000000000, 0.9510565162951535312, 1.000000000000000000, 0.9510565162951535312, 1.000000000000000000, 0.9510565162951535312, 1.000000000000000000, 0.9510565162951535312, 1.000000000000000000, 0.9510565162951535312, 1.000000000000000000, 0.9510565162951535312, 1.000000000000000000, 0.9510565162951535312, 1.000000000000000000, 0.9510565162951535312, 1.000000000000000000, 0.9510565162951535312, 1.000000000000000000, 0.9510565162951535312, 1.000000000000000000, 0.9510565162951535312, 1.000000000000000000, 0.9510565162951535312, 1.000000000000000000, 0.9510565162951535312, 1.000000000000000000, 0.9510565162951535312, 1.000000000000000000, 0.9510565162951535312, 1.000000000000000000, 0.9510565162951535312, 1.000000000000000000, 0.9510565162951535312, 1.000000000000000000, 0.9510565162951535312, 1.000000000000000000, 0.9510565162951535312, 1.000000000000000000, 0.9510565162951535312, 1.000000000000000000, 0.9510565162951535312, 1.000000000000000000, 0.9510565162951535312, 1.000000000000000000, 0.9510565162951535312, 1.000000000000000000, 0.9510565162951535312, 1.000000000000000000, 0.9510565162951535312, 1.000000000000000000, 0.9510565162951535312, 1.000000000000000000, 0.9510565162951535312, 1.000000000000000000, 0.9510565162951535312, 1.000000000000000000, 0.9510565162951535312, 1.000000000000000000, 0.9510565162951535312, 1.000000000000000000, 0.9510565162951535312, 1.000000000000000000, 0.9510565162951535312, 1.000000000000000000, 0.9510565162951535312, 1.000000000000000000, 0.9510565162951535312, 1.000000000000000000, 0.9510565162951535312, 1.000000000000000000, 0.9510565162951535312, 1.000000000000000000, 0.9510565162951535312, 1.000000000000000000, 0.9510565162951535312, 1.000000000000000000, 0.9510565162951535312, 1.000000000000000000, 0.9510565162951535312, 1.000000000000000000, 0.9510565162951535312, 1.000000000000000000, 0.9510565162951535312, 1.000000000000000000, 0.9510565162951535312, 1.000000000000000000, 0.9510565162951535312, 1.000000000000000000, 0.9510565162951535312, 1.000000000000000000, 0.9510565162951535312, 1.000000000000000000, 0.9510565162951535312, 1.000000000000000000, 0.9510565162951535312, 1.000000000000000000, 0.9510565162951535312, 1.000000000000000000, 0.9510565162951535312, 1.000000000000000000, 0.9510565162951535312, 1.000000000000000000, 0.9510565162951535312, 1.000000000000000000, 0.9510565162951535312, 1.000000000000000000, 0.9510565162951535312, 1.000000000000000000, 0.9510565162951535312, 1.000000000000000000, 0.9510565162951535312, 1.000000000000000000, 0.9510565162951535312, 1.000000000000000000, 0.9510565162951535312, 1.000000000000000000, 0.9510565162951535312, 1.000000000000000000, 0.9510565162951535312, 1.000000000000000000, 0.9510565162951535312, 1.000000000000000000, 0.9510565162951535312, 1.000000000000000000, 0.9510565162951535312, 1.000000000000000000, 0.9510565162951535312, 1.000000000000000000, 0.9510565162951535312, 1.000000000000000000, 0.9510565162951535312, 1.000000000000000000, 0.9510565162951535312, 1.000000000000000000, 0.9510565162951535312, 1.000000000000000000, 0.9510565162951535312, 1.000000000000000000, 0.9510565162951535312, 1.000000000000000000, 0.9510565162951535312, 1.000000000000000000, 0.9510565162951535312, 1.000000000000000000, 0.9510565162951535312, 1.000000000000000000, 0.9510565162951535312, 1.000000000000000000, 0.9510565162951535312, 1.000000000000000000, 0.9510565162951535312, 1.000000000000000000, 0.9510565162951535312, 1.000000000000000000, 0.9510565162951535312, 1.000000000000000000, 0.9510565162951535312, 1.000000000000000000, 0.9510565162951535312, 1.000000000000000000, 0.9510565162951535312, 1.000000000000000000, 0.9510565162951535312, 1.000000000000000000, 0.9510565162951535312, 1.000000000000000000, 0.9510565162951535312, 1.000000000000000000, 0.9510565162951535312, 1.000000000000000000, 0.9510565162951535312, 1.000000000000000000, 0.9510565162951535312, 1.000000000000000000, 0.9510565162951535312, 1.000000000000000000, 0.9510565162951535312, 1.000000000000000000, 0.9510565162951535312, 1.000000000000000000, 0.9510565162951535312, 1.000000000000000000, 0.9510565162951535312, 1.000000000000000000, 0.9510565162951535312, 1.000000000000000000, 0.9510565162951535312, 1.000000000000000000, 0.9510565162951535312, 1.000000000000000000, 0.9510565162951535312, 1.000000000000000000, 0.9510565162951535312, 1.000000000000000000, 0.9510565162951535312, 1.000000000000000000, 0.9510565162951535312, 1.000000000000000000, 0.9510565162951535312, 1.000000000000000000, 0.9510565162951535312, 1.000000000000000000, 0.9510565162951535312, 1.000000000000000000, 0.9510565162951535312, 1.000000000000000000, 0.9510565162951535312, 1.000000000000000000, 0.9510565162951535312, 1.000000000000000000, 0.9510565162951535312, 1.000000000000000000, 0.9510565162951535312, 1.000000000000000000, 0.9510565162951535312, 1.000000000000000000, 0.9510565162951535312, 1.000000000000000000, 0.9510565162951535312, 1.000000000000000000, 0.9510565162951535312, 1.000000000000000000, 0.9510565162951535312, 1.000000000000000000, 0.9510565162951535312, 1.000000000000000000, 0.9510565162951535312, 1.000000000000000000, 0.9510565162951535312, 1.000000000000000000, 0.9510565162951535312, 1.000000000000000000, 0.9510565162951535312, 1.000000000000000000) ) ) 
 REPRESENTATION_ITEM ( '' )  SURFACE ( )  );
#29812=CARTESIAN_POINT ( 'NONE',  ( 69.69999999453762030, 142.6655632788954620, -8.961492836873480528 ) ) ;
#29825=CIRCLE ( 'NONE', #15128, 2.149999999999985256 ) ;
#29831=CARTESIAN_POINT ( 'NONE',  ( 52.57499999726881157, 145.8408176439707802, 12.60653300113718345 ) ) ;
#29833=ORIENTED_EDGE ( 'NONE', *, *, #10224, .F. ) ;
#29834=CARTESIAN_POINT ( 'NONE',  ( 58.42499999726879878, 141.7447067706911810, 9.630534252274376428 ) ) ;
#29839=CARTESIAN_POINT ( 'NONE',  ( 57.67499999726880588, 168.2552932293087906, -9.630534252274385310 ) ) ;
#29841=CARTESIAN_POINT ( 'NONE',  ( 46.88867513459483405, 159.8737954434937478, -14.99999999999993072 ) ) ;
#29843=CARTESIAN_POINT ( 'NONE',  ( 83.10000000000000853, 168.7903194862797420, 4.480746418436729606 ) ) ;
#29847=AXIS2_PLACEMENT_3D ( 'NONE', #6352, #3804, #11476 ) ;
#29849=CARTESIAN_POINT ( 'NONE',  ( 44.37499999726881583, 155.0000000000000000, 15.58253174999999402 ) ) ;
#29852=CARTESIAN_POINT ( 'NONE',  ( 84.72499999726882436, 140.1801316387863778, -4.815267126137194431 ) ) ;
#29855=CARTESIAN_POINT ( 'NONE',  ( 49.61132485994281893, 150.1262045565064227, -15.00000000000002665 ) ) ;
#29856=CARTESIAN_POINT ( 'NONE',  ( 49.49999999453763166, 139.7537977485451393, -4.138211985947621020E-15 ) ) ;
#29859=CARTESIAN_POINT ( 'NONE',  ( 125.5000000000000000, 155.0000000000000000, 100.0000000000000284 ) ) ;
#29860=ORIENTED_EDGE ( 'NONE', *, *, #12023, .F. ) ;
#29866=VERTEX_POINT ( 'NONE', #7944 ) ;
#29868=AXIS2_PLACEMENT_3D ( 'NONE', #8430, #31924, #23764 ) ;
#29871=CARTESIAN_POINT ( 'NONE',  ( 33.37499999726880873, 155.0000000000000000, -15.58253175000000823 ) ) ;
#29873=CARTESIAN_POINT ( 'NONE',  ( 35.92499999726880588, 164.1591823560292198, 12.60653300113718167 ) ) ;
#29874=CARTESIAN_POINT ( 'NONE',  ( 39.48867513459482126, 167.7597621252805880, 9.270509831248428867 ) ) ;
#29878=CARTESIAN_POINT ( 'NONE',  ( 43.87499999726880162, 171.3844434931184253, -7.942151717890132712E-15 ) ) ;
#29881=ADVANCED_FACE ( 'NONE', ( #25484, #28040, #28721, #2323, #22931, #12710, #5377, #23106, #30949, #4701 ), #1981, .T. ) ;
#29884=CARTESIAN_POINT ( 'NONE',  ( 63.70000000000000995, 146.4771138417591203, 11.73074641843673227 ) ) ;
#29887=CARTESIAN_POINT ( 'NONE',  ( 77.38867513459481984, 169.2658477444273331, 4.635254915624208216 ) ) ;
#29889=CARTESIAN_POINT ( 'NONE',  ( 58.52499999726881441, 140.1801316387863778, 4.815267126137185549 ) ) ;
#29893=CARTESIAN_POINT ( 'NONE',  ( 83.77499999726880731, 169.8198683612136222, -4.815267126137197984 ) ) ;
#29907=ORIENTED_EDGE ( 'NONE', *, *, #26337, .F. ) ;
#29912=CARTESIAN_POINT ( 'NONE',  ( 85.62499999726880162, 171.3844434931184253, -7.942151717890134290E-15 ) ) ;
#29916=CARTESIAN_POINT ( 'NONE',  ( 77.62499999726880162, 171.3844434931184253, -7.942151717890132712E-15 ) ) ;
#29917=CARTESIAN_POINT ( 'NONE',  ( 54.78867513459483263, 155.0000000000000000, -15.00000000000002487 ) ) ;
#29921=CARTESIAN_POINT ( 'NONE',  ( 37.50000000000000000, 155.0000000000000000, 14.49999999999999467 ) ) ;
#29926=LINE ( 'NONE', #24981, #29537 ) ;
#29928=CARTESIAN_POINT ( 'NONE',  ( 49.82499999726881157, 168.2552932293087906, 9.630534252274372875 ) ) ;
#29935=CARTESIAN_POINT ( 'NONE',  ( 85.39999999453762314, 141.2096805137202580, 4.480746418436733158 ) ) ;
#29938=EDGE_CURVE ( 'NONE', #3719, #18876, #9334, .T. ) ;
#29940=ORIENTED_EDGE ( 'NONE', *, *, #22229, .F. ) ;
#29943=CARTESIAN_POINT ( 'NONE',  ( 69.27499999726880731, 149.9369285172503510, -15.58253175000000823 ) ) ;
#29947=CARTESIAN_POINT ( 'NONE',  ( 81.77499999726880731, 169.8198683612136222, -4.815267126137197984 ) ) ;
#29953=CARTESIAN_POINT ( 'NONE',  ( 66.97499999726881015, 140.1801316387863778, -4.815267126137194431 ) ) ;
#29955=CARTESIAN_POINT ( 'NONE',  ( 32.50000000000000000, 155.0000000000000000, -15.00000000000002487 ) ) ;
#29962=CARTESIAN_POINT ( 'NONE',  ( 70.71132485994280614, 155.0000000000000000, 15.00000000000001243 ) ) ;
#29965=CARTESIAN_POINT ( 'NONE',  ( 45.32499999726881157, 164.1591823560292198, -12.60653300113719766 ) ) ;
#29967=CARTESIAN_POINT ( 'NONE',  ( 87.49999999999998579, 159.6603719825695862, -14.83369040333126954 ) ) ;
#29973=CARTESIAN_POINT ( 'NONE',  ( 76.48867513459482836, 142.2402378747194405, -9.270509831248439525 ) ) ;
#29978=CARTESIAN_POINT ( 'NONE',  ( 63.79999999453762882, 146.4771138417591203, -11.73074641843674470 ) ) ;
#29984=CARTESIAN_POINT ( 'NONE',  ( 76.31132485994280046, 169.2658477444273331, 4.635254915624208216 ) ) ;
#29988=ORIENTED_EDGE ( 'NONE', *, *, #6328, .T. ) ;
#29989=CARTESIAN_POINT ( 'NONE',  ( 32.50000000000000000, 155.0000000000000000, -6.938893903907228378E-15 ) ) ;
#29993=CARTESIAN_POINT ( 'NONE',  ( 85.31132485994280046, 140.7341522555726669, -4.635254915624220651 ) ) ;
#29995=CARTESIAN_POINT ( 'NONE',  ( 53.27499999726881441, 149.9369285172503510, -15.58253175000000823 ) ) ;
#29999=CARTESIAN_POINT ( 'NONE',  ( 57.21132485994281325, 139.2280666364260071, -4.041636747397287284E-15 ) ) ;
#30001=CARTESIAN_POINT ( 'NONE',  ( 62.47499999726881725, 149.9369285172503510, 15.58253174999999580 ) ) ;
#30006=CARTESIAN_POINT ( 'NONE',  ( 78.20000000000001705, 142.6655632788954620, -8.961492836873480528 ) ) ;
#30010=CARTESIAN_POINT ( 'NONE',  ( 43.07499999726881157, 141.7447067706911810, -9.630534252274385310 ) ) ;
#30012=EDGE_CURVE ( 'NONE', #22486, #19088, #4834, .T. ) ;
#30013=CARTESIAN_POINT ( 'NONE',  ( 82.82499999726881867, 141.7447067706911810, -9.630534252274385310 ) ) ;
#30016=CARTESIAN_POINT ( 'NONE',  ( 47.29999999453762172, 142.6655632788954620, 8.961492836873471646 ) ) ;
#30019=ADVANCED_FACE ( 'NONE', ( #13697 ), #23935, .T. ) ;
#30033=CARTESIAN_POINT ( 'NONE',  ( 34.17499999726881299, 164.1591823560292198, 12.60653300113718167 ) ) ;
#30035=CARTESIAN_POINT ( 'NONE',  ( 35.82499999726880446, 168.2552932293087906, 9.630534252274372875 ) ) ;
#30040=CARTESIAN_POINT ( 'NONE',  ( 38.67499999726879878, 141.7447067706911810, 9.630534252274376428 ) ) ;
#30043=CARTESIAN_POINT ( 'NONE',  ( 62.60000000000000142, 159.7113355953771077, -14.50000000000000888 ) ) ;
#30047=CARTESIAN_POINT ( 'NONE',  ( 32.50000000000000000, 155.0000000000000000, 15.00000000000001243 ) ) ;
#30048=CARTESIAN_POINT ( 'NONE',  ( 65.62499999726880162, 171.3844434931184253, -7.942151717890132712E-15 ) ) ;
#30053=CARTESIAN_POINT ( 'NONE',  ( 80.47499999726881015, 149.9369285172503510, 15.58253174999999580 ) ) ;
#30055=VECTOR ( 'NONE', #20390, 1000.000000000000000 ) ;
#30056=CYLINDRICAL_SURFACE ( 'NONE', #16470, 2.149999999999984812 ) ;
#30067=CARTESIAN_POINT ( 'NONE',  ( 39.51132485994280330, 146.1832212156128890, -12.13525491562423042 ) ) ;
#30072=CARTESIAN_POINT ( 'NONE',  ( 87.12499999726880162, 155.0000000000000000, -15.58253175000000823 ) ) ;
#30074=CARTESIAN_POINT ( 'NONE',  ( 32.50000000000000000, 155.0000000000000000, -15.00000000000002487 ) ) ;
#30077=CARTESIAN_POINT ( 'NONE',  ( 77.02499999726880731, 149.9369285172503510, -15.58253175000000823 ) ) ;
#30078=DIRECTION ( 'NONE',  ( -1.000000000000000000, 0.000000000000000000, 0.000000000000000000 ) ) ;
#30080=CARTESIAN_POINT ( 'NONE',  ( 87.50000000000004263, 170.1307320771869627, -3.377640367381898212 ) ) ;
#30081=CARTESIAN_POINT ( 'NONE',  ( 44.60000000000000142, 159.7113355953771077, -14.50000000000000888 ) ) ;
#30085=DIRECTION ( 'NONE',  ( 1.000000000000000000, 0.000000000000000000, 0.000000000000000000 ) ) ;
#30086=DIRECTION ( 'NONE',  ( 1.000000000000000000, 0.000000000000000000, 0.000000000000000000 ) ) ;
#30087=CARTESIAN_POINT ( 'NONE',  ( 48.92499999726881299, 145.8408176439707802, -12.60653300113719588 ) ) ;
#30088=CARTESIAN_POINT ( 'NONE',  ( 62.77499999726882152, 140.1801316387863778, 4.815267126137185549 ) ) ;
#30090=DIRECTION ( 'NONE',  ( 1.000000000000000000, 0.000000000000000000, 0.000000000000000000 ) ) ;
#30096=CARTESIAN_POINT ( 'NONE',  ( 88.09999999453761177, 159.7113355953771077, -14.50000000000000888 ) ) ;
#30100=AXIS2_PLACEMENT_3D ( 'NONE', #19807, #24917, #22697 ) ;
#30103=AXIS2_PLACEMENT_3D ( 'NONE', #11016, #32408, #10857 ) ;
#30108=CARTESIAN_POINT ( 'NONE',  ( 71.57499999726881867, 164.1591823560292198, -12.60653300113719766 ) ) ;
#30111=CARTESIAN_POINT ( 'NONE',  ( 82.57499999726880446, 145.8408176439707802, 12.60653300113718345 ) ) ;
#30114=VECTOR ( 'NONE', #12923, 1000.000000000000114 ) ;
#30124=CARTESIAN_POINT ( 'NONE',  ( 85.71132485994282035, 155.0000000000000000, -15.00000000000002487 ) ) ;
#30129=CARTESIAN_POINT ( 'NONE',  ( 67.38867513459481984, 169.2658477444273331, 4.635254915624208216 ) ) ;
#30133=CARTESIAN_POINT ( 'NONE',  ( 46.62499999726880873, 138.6155565068815463, -3.929120461958505118E-15 ) ) ;
#30135=CARTESIAN_POINT ( 'NONE',  ( 87.49999999999995737, 158.6695690980871518, -15.06022462549181817 ) ) ;
#30141=DIRECTION ( 'NONE',  ( 0.000000000000000000, 0.000000000000000000, -1.000000000000000000 ) ) ;
#30146=CARTESIAN_POINT ( 'NONE',  ( 67.29999999453761461, 142.6655632788954620, 8.961492836873471646 ) ) ;
#30152=CARTESIAN_POINT ( 'NONE',  ( 75.71132485994280614, 155.0000000000000000, -15.00000000000002487 ) ) ;
#30153=VERTEX_POINT ( 'NONE', #5538 ) ;
#30156=ORIENTED_EDGE ( 'NONE', *, *, #16367, .T. ) ;
#30157=DIRECTION ( 'NONE',  ( 1.000000000000000000, 0.000000000000000000, 0.000000000000000000 ) ) ;
#30162=CARTESIAN_POINT ( 'NONE',  ( 84.91132485994279477, 146.1832212156128890, 12.13525491562421976 ) ) ;
#30164=CARTESIAN_POINT ( 'NONE',  ( 54.47499999726880304, 149.9369285172503510, 15.58253174999999580 ) ) ;
#30167=CARTESIAN_POINT ( 'NONE',  ( 67.51132485994278909, 146.1832212156128890, -12.13525491562423042 ) ) ;
#30169=CARTESIAN_POINT ( 'NONE',  ( 57.31132485994280756, 140.7341522555726669, -4.635254915624220651 ) ) ;
#30171=CARTESIAN_POINT ( 'NONE',  ( 59.87499999726882294, 171.3844434931184253, -7.942151717890132712E-15 ) ) ;
#30173=CARTESIAN_POINT ( 'NONE',  ( 70.38867513459481984, 140.7341522555726669, -4.635254915624220651 ) ) ;
#30177=CARTESIAN_POINT ( 'NONE',  ( 78.60000000000000853, 159.7113355953771077, -14.50000000000000888 ) ) ;
#30182=CARTESIAN_POINT ( 'NONE',  ( 44.27499999726881441, 160.0630714827496206, 15.58253174999999402 ) ) ;
#30185=CARTESIAN_POINT ( 'NONE',  ( 86.52499999726882152, 140.1801316387863778, 4.815267126137185549 ) ) ;
#30188=CARTESIAN_POINT ( 'NONE',  ( 49.59999999453763309, 141.2096805137202580, -4.480746418436742040 ) ) ;
#30191=CARTESIAN_POINT ( 'NONE',  ( 80.71132485994280614, 155.0000000000000000, 15.00000000000001243 ) ) ;
#30202=ADVANCED_FACE ( 'NONE', ( #12124 ), #28133, .T. ) ;
#30207=CARTESIAN_POINT ( 'NONE',  ( 39.22499999726881015, 160.0630714827496206, -15.58253175000000823 ) ) ;
#30208=DIRECTION ( 'NONE',  ( 1.000000000000000000, 0.000000000000000000, 0.000000000000000000 ) ) ;
#30212=CARTESIAN_POINT ( 'NONE',  ( 39.47499999726881015, 160.0630714827496206, -15.58253175000000823 ) ) ;
#30217=CARTESIAN_POINT ( 'NONE',  ( 58.30000000000000426, 146.4771138417591203, -11.73074641843674470 ) ) ;
#30218=CARTESIAN_POINT ( 'NONE',  ( 64.11132485994281183, 169.2658477444273331, -4.635254915624224203 ) ) ;
#30220=DIRECTION ( 'NONE',  ( 1.000000000000000000, 0.000000000000000000, 0.000000000000000000 ) ) ;
#30224=CARTESIAN_POINT ( 'NONE',  ( 67.22499999726879594, 160.0630714827496206, -15.58253175000000823 ) ) ;
#30226=ORIENTED_EDGE ( 'NONE', *, *, #13733, .T. ) ;
#30228=CARTESIAN_POINT ( 'NONE',  ( 80.37499999726881583, 155.0000000000000000, 15.58253174999999402 ) ) ;
#30244=ORIENTED_EDGE ( 'NONE', *, *, #30492, .F. ) ;
#30245=CARTESIAN_POINT ( 'NONE',  ( 83.82499999726880446, 168.2552932293087906, 9.630534252274372875 ) ) ;
#30248=CARTESIAN_POINT ( 'NONE',  ( 75.62499999726881583, 171.3844434931184253, -7.942151717890132712E-15 ) ) ;
#30252=CARTESIAN_POINT ( 'NONE',  ( 40.19999999999999574, 142.6655632788954620, -8.961492836873480528 ) ) ;
#30257=LINE ( 'NONE', #25138, #2972 ) ;
#30258=CARTESIAN_POINT ( 'NONE',  ( 48.12499999726880873, 155.0000000000000000, 15.58253174999999402 ) ) ;
#30259=CARTESIAN_POINT ( 'NONE',  ( 61.57499999726881157, 164.1591823560292198, -12.60653300113719766 ) ) ;
#30271=DIRECTION ( 'NONE',  ( 0.000000000000000000, 0.000000000000000000, -1.000000000000000000 ) ) ;
#30275=CARTESIAN_POINT ( 'NONE',  ( 71.87499999726881583, 171.3844434931184253, -7.942151717890132712E-15 ) ) ;
#30277=VERTEX_POINT ( 'NONE', #17064 ) ;
#30279=CARTESIAN_POINT ( 'NONE',  ( 82.17499999726882720, 164.1591823560292198, 12.60653300113718167 ) ) ;
#30298=CARTESIAN_POINT ( 'NONE',  ( 42.22499999726879594, 149.9369285172503510, 15.58253174999999580 ) ) ;
#30300=CARTESIAN_POINT ( 'NONE',  ( 34.62499999726881583, 138.6155565068815747, -3.929120461958505118E-15 ) ) ;
#30302=CARTESIAN_POINT ( 'NONE',  ( 127.5000000000000000, 155.0000000000000000, -98.00000000000002842 ) ) ;
#30307=AXIS2_PLACEMENT_3D ( 'NONE', #1702, #6819, #25213 ) ;
#30311=CARTESIAN_POINT ( 'NONE',  ( 71.99999999453763166, 155.0000000000000000, -14.50000000000000711 ) ) ;
#30316=CARTESIAN_POINT ( 'NONE',  ( 45.11132485994280472, 140.7341522555726669, 4.635254915624211769 ) ) ;
#30319=ORIENTED_EDGE ( 'NONE', *, *, #27480, .T. ) ;
#30320=ORIENTED_EDGE ( 'NONE', *, *, #1464, .T. ) ;
#30321=CARTESIAN_POINT ( 'NONE',  ( 42.38867513459481984, 140.7341522555726669, -4.635254915624220651 ) ) ;
#30326=CARTESIAN_POINT ( 'NONE',  ( 85.71132485994282035, 155.0000000000000000, -15.00000000000002487 ) ) ;
#30329=CARTESIAN_POINT ( 'NONE',  ( 56.07499999726881157, 168.2552932293087906, 9.630534252274372875 ) ) ;
#30332=CARTESIAN_POINT ( 'NONE',  ( 67.41132485994280898, 142.2402378747194405, -9.270509831248439525 ) ) ;
#30337=CARTESIAN_POINT ( 'NONE',  ( 63.67499999726880588, 168.2552932293087906, -9.630534252274385310 ) ) ;
#30339=CARTESIAN_POINT ( 'NONE',  ( 70.18867513459481700, 140.7341522555726669, 4.635254915624211769 ) ) ;
#30344=CARTESIAN_POINT ( 'NONE',  ( 78.99999999999998579, 170.2462022514548323, -7.872454543227099337E-15 ) ) ;
#30349=CARTESIAN_POINT ( 'NONE',  ( 50.37499999726881583, 155.0000000000000000, 15.58253174999999402 ) ) ;
#30351=CARTESIAN_POINT ( 'NONE',  ( 80.22499999726881015, 149.9369285172503510, 15.58253174999999580 ) ) ;
#30352=EDGE_CURVE ( 'NONE', #31659, #31983, #21700, .T. ) ;
#30354=CARTESIAN_POINT ( 'NONE',  ( 50.69999999453762740, 167.3344367211045096, 8.961492836873468093 ) ) ;
#30355=( BOUNDED_CURVE ( )  B_SPLINE_CURVE ( 2, ( #21368, #31764, #11323, #29546, #24093, #21707, #10831, #16589, #760, #31600, #3645 ),
 .UNSPECIFIED., .F., .F. ) 
 B_SPLINE_CURVE_WITH_KNOTS ( ( 3, 2, 2, 2, 2, 3 ),
 ( 0.05357142857142861703, 0.05714285714285716883, 0.06071428571428571369, 0.06428571428571425161, 0.06785714285714281035, 0.07142857142857135522 ),
 .UNSPECIFIED. ) 
 CURVE ( )  GEOMETRIC_REPRESENTATION_ITEM ( )  RATIONAL_B_SPLINE_CURVE ( ( 0.9999999999999994449, 0.9510565162951540863, 1.000000000000000000, 0.9510565162951534202, 1.000000000000000000, 0.9510565162951534202, 1.000000000000000000, 0.9510565162951534202, 1.000000000000000000, 0.9510565162951544194, 0.9999999999999990008 ) ) 
 REPRESENTATION_ITEM ( '' )  );
#30359=CARTESIAN_POINT ( 'NONE',  ( 125.5000000000000000, 48.99999999999998579, -2.149999999999999023 ) ) ;
#30361=AXIS2_PLACEMENT_3D ( 'NONE', #2386, #12939, #12775 ) ;
#30363=ORIENTED_EDGE ( 'NONE', *, *, #27227, .F. ) ;
#30371=EDGE_LOOP ( 'NONE', ( #11679, #20303 ) ) ;
#30376=CARTESIAN_POINT ( 'NONE',  ( 40.47499999726881725, 149.9369285172503510, 15.58253174999999580 ) ) ;
#30378=CARTESIAN_POINT ( 'NONE',  ( 47.52499999726881441, 169.8198683612136222, -4.815267126137197984 ) ) ;
#30379=CARTESIAN_POINT ( 'NONE',  ( 38.98867513459482126, 163.8167787843871110, -12.13525491562423397 ) ) ;
#30380=CARTESIAN_POINT ( 'NONE',  ( 54.51132485994281041, 163.8167787843871110, 12.13525491562421621 ) ) ;
#30383=CARTESIAN_POINT ( 'NONE',  ( 46.67499999726880588, 141.7447067706911810, 9.630534252274376428 ) ) ;
#30386=CARTESIAN_POINT ( 'NONE',  ( 58.61132485994280472, 159.8737954434936910, 14.99999999999996447 ) ) ;
#30387=CARTESIAN_POINT ( 'NONE',  ( 57.90000000000000568, 141.2096805137202580, 4.480746418436733158 ) ) ;
#30389=CARTESIAN_POINT ( 'NONE',  ( 47.71132485994280614, 155.0000000000000000, -15.00000000000002487 ) ) ;
#30394=VECTOR ( 'NONE', #14288, 1000.000000000000000 ) ;
#30395=CARTESIAN_POINT ( 'NONE',  ( 65.22499999726881015, 160.0630714827496206, -15.58253175000000823 ) ) ;
#30399=CARTESIAN_POINT ( 'NONE',  ( 84.57499999726880446, 145.8408176439707802, 12.60653300113718345 ) ) ;
#30401=EDGE_CURVE ( 'NONE', #25104, #534, #10653, .T. ) ;
#30403=CARTESIAN_POINT ( 'NONE',  ( 72.58867513459482268, 146.1832212156128890, -12.13525491562423042 ) ) ;
#30423=VERTEX_POINT ( 'NONE', #15853 ) ;
#30424=CARTESIAN_POINT ( 'NONE',  ( 76.32499999726881867, 145.8408176439707802, 12.60653300113718345 ) ) ;
#30428=CARTESIAN_POINT ( 'NONE',  ( 43.20000000000000995, 167.3344367211045096, 8.961492836873468093 ) ) ;
#30434=CARTESIAN_POINT ( 'NONE',  ( 50.12499999726881583, 155.0000000000000000, 15.58253174999999402 ) ) ;
#30435=CARTESIAN_POINT ( 'NONE',  ( 61.17499999726882010, 145.8408176439707802, -12.60653300113719588 ) ) ;
#30443=DIRECTION ( 'NONE',  ( -1.000000000000000000, -0.000000000000000000, 0.000000000000000000 ) ) ;
#30445=CARTESIAN_POINT ( 'NONE',  ( 83.41132485994282320, 142.2402378747194405, -9.270509831248439525 ) ) ;
#30452=CARTESIAN_POINT ( 'NONE',  ( 79.77499999726880731, 169.8198683612136222, -4.815267126137197984 ) ) ;
#30456=CARTESIAN_POINT ( 'NONE',  ( 84.57499999726880446, 145.8408176439707802, 12.60653300113718345 ) ) ;
#30458=DIRECTION ( 'NONE',  ( 0.000000000000000000, -1.000000000000000000, 1.290957005378097920E-14 ) ) ;
#30459=CARTESIAN_POINT ( 'NONE',  ( 58.82499999726881867, 141.7447067706911810, -9.630534252274385310 ) ) ;
#30462=VERTEX_POINT ( 'NONE', #4967 ) ;
#30472=CARTESIAN_POINT ( 'NONE',  ( 53.12499999726881583, 155.0000000000000000, -15.58253175000000823 ) ) ;
#30474=CARTESIAN_POINT ( 'NONE',  ( 87.49999999999998579, 148.5314199800102415, -13.68475861882792088 ) ) ;
#30483=CARTESIAN_POINT ( 'NONE',  ( 74.69999999453764872, 167.3344367211045096, 8.961492836873468093 ) ) ;
#30492=EDGE_CURVE ( 'NONE', #23167, #22913, #26069, .T. ) ;
#30493=CARTESIAN_POINT ( 'NONE',  ( 58.08867513459483689, 142.2402378747194405, 9.270509831248432420 ) ) ;
#30494=CARTESIAN_POINT ( 'NONE',  ( 32.50000000000000000, 155.0000000000000000, -6.938893903907228378E-15 ) ) ;
#30499=CARTESIAN_POINT ( 'NONE',  ( 56.47499999726882436, 149.9369285172503510, 15.58253174999999580 ) ) ;
#30505=CARTESIAN_POINT ( 'NONE',  ( 65.47499999726881015, 160.0630714827496206, -15.58253175000000823 ) ) ;
#30507=DIRECTION ( 'NONE',  ( 0.000000000000000000, 0.7071067811865442421, -0.7071067811865506814 ) ) ;
#30511=CARTESIAN_POINT ( 'NONE',  ( 82.20000000000000284, 142.6655632788954620, -8.961492836873480528 ) ) ;
#30516=CARTESIAN_POINT ( 'NONE',  ( 52.37499999726881583, 155.0000000000000000, 15.58253174999999402 ) ) ;
#30518=CARTESIAN_POINT ( 'NONE',  ( 83.82499999726880446, 168.2552932293087906, 9.630534252274372875 ) ) ;
#30521=CARTESIAN_POINT ( 'NONE',  ( 51.99999999453763166, 155.0000000000000000, -14.50000000000000711 ) ) ;
#30524=DIRECTION ( 'NONE',  ( -1.000000000000000000, 0.000000000000000000, 0.000000000000000000 ) ) ;
#30528=ORIENTED_EDGE ( 'NONE', *, *, #19093, .F. ) ;
#30541=CARTESIAN_POINT ( 'NONE',  ( 35.77499999726881441, 169.8198683612136222, -4.815267126137197984 ) ) ;
#30543=CARTESIAN_POINT ( 'NONE',  ( 42.22499999726879594, 149.9369285172503510, 15.58253174999999580 ) ) ;
#30544=CARTESIAN_POINT ( 'NONE',  ( 39.08867513459482268, 167.7597621252805880, -9.270509831248443078 ) ) ;
#30546=CARTESIAN_POINT ( 'NONE',  ( 54.21132485994281325, 170.7719333635740497, -7.904646289410545231E-15 ) ) ;
#30548=CARTESIAN_POINT ( 'NONE',  ( 50.27499999726880731, 160.0630714827496206, 15.58253174999999402 ) ) ;
#30551=CARTESIAN_POINT ( 'NONE',  ( 58.51132485994281041, 163.8167787843871110, 12.13525491562421621 ) ) ;
#30552=CARTESIAN_POINT ( 'NONE',  ( 61.10000000000000142, 168.7903194862797420, 4.480746418436729606 ) ) ;
#30553=( BOUNDED_CURVE ( )  B_SPLINE_CURVE ( 2, ( #11031, #17473, #22250, #28035, #11863, #6579, #6749, #27858, #32637, #1307, #19532 ),
 .UNSPECIFIED., .F., .F. ) 
 B_SPLINE_CURVE_WITH_KNOTS ( ( 3, 2, 2, 2, 2, 3 ),
 ( 0.6964285714285713969, 0.6999999999999999556, 0.7035714285714286254, 0.7071428571428570731, 0.7107142857142856318, 0.7142857142857141906 ),
 .UNSPECIFIED. ) 
 CURVE ( )  GEOMETRIC_REPRESENTATION_ITEM ( )  RATIONAL_B_SPLINE_CURVE ( ( 1.000000000000000000, 0.9510565162951534202, 1.000000000000000000, 0.9510565162951534202, 1.000000000000000000, 0.9510565162951534202, 1.000000000000000000, 0.9510565162951534202, 1.000000000000000000, 0.9510565162951549745, 0.9999999999999984457 ) ) 
 REPRESENTATION_ITEM ( '' )  );
#30558=CARTESIAN_POINT ( 'NONE',  ( 33.67499999726881299, 168.2552932293087906, -9.630534252274385310 ) ) ;
#30560=CARTESIAN_POINT ( 'NONE',  ( 64.62499999726881583, 138.6155565068815463, -3.929120461958505118E-15 ) ) ;
#30564=CARTESIAN_POINT ( 'NONE',  ( 86.77499999726882152, 140.1801316387863778, 4.815267126137185549 ) ) ;
#30568=FACE_OUTER_BOUND ( 'NONE', #21839, .T. ) ;
#30583=CARTESIAN_POINT ( 'NONE',  ( 125.5000000000000000, 155.0000000000000000, -6.938893903907228378E-15 ) ) ;
#30587=CARTESIAN_POINT ( 'NONE',  ( 73.67499999726879878, 168.2552932293087906, -9.630534252274387086 ) ) ;
#30588=CARTESIAN_POINT ( 'NONE',  ( 82.82499999726881867, 141.7447067706911810, -9.630534252274385310 ) ) ;
#30595=CARTESIAN_POINT ( 'NONE',  ( 44.90000000000000568, 168.7903194862797420, -4.480746418436745593 ) ) ;
#30597=ADVANCED_FACE ( 'NONE', ( #2899 ), #13286, .T. ) ;
#30601=CARTESIAN_POINT ( 'NONE',  ( 57.22499999726880304, 160.0630714827496206, -15.58253175000000823 ) ) ;
#30602=CARTESIAN_POINT ( 'NONE',  ( 66.47499999726882436, 149.9369285172503510, 15.58253174999999580 ) ) ;
#30620=CARTESIAN_POINT ( 'NONE',  ( 77.87499999726881583, 171.3844434931184253, -7.942151717890132712E-15 ) ) ;
#30625=CARTESIAN_POINT ( 'NONE',  ( 70.32499999726881867, 145.8408176439707802, 12.60653300113718345 ) ) ;
#30626=CARTESIAN_POINT ( 'NONE',  ( 32.50000000000000000, 155.0000000000000000, -15.00000000000002487 ) ) ;
#30628=CARTESIAN_POINT ( 'NONE',  ( 64.92499999726881299, 145.8408176439707802, -12.60653300113719588 ) ) ;
#30629=ADVANCED_FACE ( 'NONE', ( #9900 ), #28118, .T. ) ;
#30635=AXIS2_PLACEMENT_3D ( 'NONE', #5627, #21294, #31688 ) ;
#30636=CARTESIAN_POINT ( 'NONE',  ( 127.5000000000000000, 80.04668119422662187, 74.95331880577468553 ) ) ;
#30640=CARTESIAN_POINT ( 'NONE',  ( 45.18867513459481700, 169.2658477444273331, -4.635254915624224203 ) ) ;
#30647=CARTESIAN_POINT ( 'NONE',  ( 35.82499999726880446, 168.2552932293087906, 9.630534252274372875 ) ) ;
#30653=CIRCLE ( 'NONE', #30103, 15.00000000000001776 ) ;
#30658=CARTESIAN_POINT ( 'NONE',  ( 73.39999999453763735, 141.2096805137202580, 4.480746418436733158 ) ) ;
#30664=ORIENTED_EDGE ( 'NONE', *, *, #12713, .F. ) ;
#30666=ORIENTED_EDGE ( 'NONE', *, *, #537, .F. ) ;
#30669=CARTESIAN_POINT ( 'NONE',  ( 51.38867513459482694, 169.2658477444273331, 4.635254915624208216 ) ) ;
#30670=CARTESIAN_POINT ( 'NONE',  ( 127.5000000000000000, 152.8499999999996533, -106.0000000000000000 ) ) ;
#30674=CIRCLE ( 'NONE', #17037, 2.149999999999985256 ) ;
#30675=CARTESIAN_POINT ( 'NONE',  ( 55.61132485994281183, 150.1262045565064227, -15.00000000000002665 ) ) ;
#30678=CARTESIAN_POINT ( 'NONE',  ( 54.27499999726880731, 160.0630714827496206, 15.58253174999999224 ) ) ;
#30685=CARTESIAN_POINT ( 'NONE',  ( 64.57499999726881867, 145.8408176439707802, 12.60653300113718345 ) ) ;
#30691=CARTESIAN_POINT ( 'NONE',  ( 84.90000000000000568, 168.7903194862797420, -4.480746418436745593 ) ) ;
#30692=DIRECTION ( 'NONE',  ( 1.000000000000000000, 0.000000000000000000, 0.000000000000000000 ) ) ;
#30695=CARTESIAN_POINT ( 'NONE',  ( 125.5000000000000000, 155.0000000000000000, -112.0000000000000711 ) ) ;
#30696=CARTESIAN_POINT ( 'NONE',  ( 48.47499999726880304, 149.9369285172503510, 15.58253174999999580 ) ) ;
#30699=CARTESIAN_POINT ( 'NONE',  ( 52.51132485994281041, 163.8167787843871110, 12.13525491562421621 ) ) ;
#30701=CARTESIAN_POINT ( 'NONE',  ( 51.39999999453763735, 141.2096805137202580, 4.480746418436733158 ) ) ;
#30704=CARTESIAN_POINT ( 'NONE',  ( 47.01132485994281041, 142.2402378747194405, 9.270509831248432420 ) ) ;
#30708=ORIENTED_EDGE ( 'NONE', *, *, #3053, .T. ) ;
#30719=CARTESIAN_POINT ( 'NONE',  ( 35.67499999726880588, 168.2552932293087906, -9.630534252274387086 ) ) ;
#30721=CARTESIAN_POINT ( 'NONE',  ( 46.52499999726881441, 140.1801316387863778, 4.815267126137185549 ) ) ;
#30725=CARTESIAN_POINT ( 'NONE',  ( 49.87499999726880162, 171.3844434931184253, -7.942151717890132712E-15 ) ) ;
#30729=CARTESIAN_POINT ( 'NONE',  ( 68.90000000000000568, 168.7903194862797420, -4.480746418436745593 ) ) ;
#30737=CARTESIAN_POINT ( 'NONE',  ( 61.42499999726882010, 168.2552932293087906, -9.630534252274385310 ) ) ;
#30741=CARTESIAN_POINT ( 'NONE',  ( 36.79999999453762882, 163.5228861582408797, 11.73074641843673049 ) ) ;
#30749=CARTESIAN_POINT ( 'NONE',  ( 66.58867513459482268, 146.1832212156128890, -12.13525491562423042 ) ) ;
#30752=ORIENTED_EDGE ( 'NONE', *, *, #19153, .T. ) ;
#30755=ORIENTED_EDGE ( 'NONE', *, *, #17013, .F. ) ;
#30756=CARTESIAN_POINT ( 'NONE',  ( 38.78867513459481842, 155.0000000000000000, -15.00000000000002487 ) ) ;
#30757=ORIENTED_EDGE ( 'NONE', *, *, #12320, .F. ) ;
#30758=CARTESIAN_POINT ( 'NONE',  ( 80.71132485994280614, 155.0000000000000000, 15.00000000000001243 ) ) ;
#30760=( BOUNDED_CURVE ( )  B_SPLINE_CURVE ( 2, ( #28116, #7350, #14828, #25058, #30173, #9724, #30339, #32547, #14488, #27774, #15172 ),
 .UNSPECIFIED., .F., .T. ) 
 B_SPLINE_CURVE_WITH_KNOTS ( ( 3, 2, 2, 2, 2, 3 ),
 ( 0.3035714285714283256, 0.3071428571428568843, 0.3107142857142855541, 0.3142857142857141128, 0.3178571428571426716, 0.3214285714285712303 ),
 .UNSPECIFIED. ) 
 CURVE ( )  GEOMETRIC_REPRESENTATION_ITEM ( )  RATIONAL_B_SPLINE_CURVE ( ( 1.000000000000002220, 0.9510565162951510887, 1.000000000000000000, 0.9510565162951534202, 1.000000000000000000, 0.9510565162951534202, 1.000000000000000000, 0.9510565162951534202, 1.000000000000000000, 0.9510565162951557516, 0.9999999999999976685 ) ) 
 REPRESENTATION_ITEM ( '' )  );
#30762=CARTESIAN_POINT ( 'NONE',  ( 80.02499999726882152, 160.0630714827496206, 15.58253174999999402 ) ) ;
#30766=CARTESIAN_POINT ( 'NONE',  ( 38.69999999999999574, 163.5228861582408797, -11.73074641843674470 ) ) ;
#30769=DIRECTION ( 'NONE',  ( -1.000000000000000000, 0.000000000000000000, 0.000000000000000000 ) ) ;
#30772=CARTESIAN_POINT ( 'NONE',  ( 57.62499999726880873, 171.3844434931184253, -7.942151717890134290E-15 ) ) ;
#30773=CARTESIAN_POINT ( 'NONE',  ( 70.67499999726881299, 141.7447067706911810, 9.630534252274376428 ) ) ;
#30775=CARTESIAN_POINT ( 'NONE',  ( 127.5000000000000000, 155.0000000000000000, -6.938893903907228378E-15 ) ) ;
#30778=ADVANCED_FACE ( 'NONE', ( #9083 ), #24931, .T. ) ;
#30791=CARTESIAN_POINT ( 'NONE',  ( 78.77499999726880731, 140.1801316387863778, 4.815267126137185549 ) ) ;
#30795=CARTESIAN_POINT ( 'NONE',  ( 69.32499999726881867, 164.1591823560292198, -12.60653300113719766 ) ) ;
#30799=CARTESIAN_POINT ( 'NONE',  ( 66.12499999726881583, 155.0000000000000000, 15.58253174999999402 ) ) ;
#30805=CARTESIAN_POINT ( 'NONE',  ( 57.78867513459481842, 155.0000000000000000, 15.00000000000001243 ) ) ;
#30809=CYLINDRICAL_SURFACE ( 'NONE', #16929, 100.0000000000000000 ) ;
#30813=CARTESIAN_POINT ( 'NONE',  ( 86.77499999726882152, 140.1801316387863778, 4.815267126137185549 ) ) ;
#30815=CARTESIAN_POINT ( 'NONE',  ( 38.52499999726881441, 140.1801316387863778, 4.815267126137185549 ) ) ;
#30823=CARTESIAN_POINT ( 'NONE',  ( 71.69999999453763451, 142.6655632788954620, -8.961492836873480528 ) ) ;
#30838=CIRCLE ( 'NONE', #20498, 112.0000000000000711 ) ;
#30840=CARTESIAN_POINT ( 'NONE',  ( 56.28867513459483263, 139.2280666364260071, -4.041636747397287284E-15 ) ) ;
#30846=CARTESIAN_POINT ( 'NONE',  ( 54.67499999726881299, 141.7447067706911810, 9.630534252274376428 ) ) ;
#30847=EDGE_LOOP ( 'NONE', ( #14225, #24909, #31543, #14215 ) ) ;
#30849=CARTESIAN_POINT ( 'NONE',  ( 68.28867513459482552, 139.2280666364260071, -4.041636747397287284E-15 ) ) ;
#30852=CARTESIAN_POINT ( 'NONE',  ( 66.37499999726881583, 155.0000000000000000, 15.58253174999999402 ) ) ;
#30854=DIRECTION ( 'NONE',  ( 1.000000000000000000, 0.000000000000000000, 0.000000000000000000 ) ) ;
#30860=CARTESIAN_POINT ( 'NONE',  ( 86.99999999999998579, 170.2462022514548323, -7.872454543227099337E-15 ) ) ;
#30862=CARTESIAN_POINT ( 'NONE',  ( 32.50000000000000000, 155.0000000000000000, -15.00000000000002487 ) ) ;
#30864=CARTESIAN_POINT ( 'NONE',  ( 47.98867513459481415, 146.1832212156128890, 12.13525491562421976 ) ) ;
#30865=CARTESIAN_POINT ( 'NONE',  ( 50.47499999726880304, 149.9369285172503510, 15.58253174999999580 ) ) ;
#30868=CIRCLE ( 'NONE', #3628, 70.00000000000000000 ) ;
#30869=CARTESIAN_POINT ( 'NONE',  ( 88.12499999726880162, 155.0000000000000000, 15.58253174999999402 ) ) ;
#30870=CARTESIAN_POINT ( 'NONE',  ( 77.81132485994280046, 159.8737954434936057, -15.00000000000002665 ) ) ;
#30872=CARTESIAN_POINT ( 'NONE',  ( 53.19999999453762740, 146.4771138417591203, 11.73074641843673227 ) ) ;
#30873=ORIENTED_EDGE ( 'NONE', *, *, #16655, .F. ) ;
#30881=VECTOR ( 'NONE', #22661, 1000.000000000000000 ) ;
#30884=STYLED_ITEM ( 'NONE', ( #658 ), #789 ) ;
#30889=CARTESIAN_POINT ( 'NONE',  ( 37.97499999726881015, 169.8198683612136222, 4.815267126137181997 ) ) ;
#30892=CARTESIAN_POINT ( 'NONE',  ( 41.92499999726881299, 164.1591823560292198, 12.60653300113718167 ) ) ;
#30896=CARTESIAN_POINT ( 'NONE',  ( 47.67499999726880588, 168.2552932293087906, -9.630534252274385310 ) ) ;
#30900=CARTESIAN_POINT ( 'NONE',  ( 68.79999999999999716, 167.3344367211045096, -8.961492836873482304 ) ) ;
#30906=CARTESIAN_POINT ( 'NONE',  ( 33.77499999726880731, 169.8198683612136222, -4.815267126137197984 ) ) ;
#30909=CARTESIAN_POINT ( 'NONE',  ( 73.32499999726880446, 164.1591823560292198, -12.60653300113719766 ) ) ;
#30910=ORIENTED_EDGE ( 'NONE', *, *, #14399, .T. ) ;
#30912=CARTESIAN_POINT ( 'NONE',  ( 37.19999999453762740, 146.4771138417591203, 11.73074641843673227 ) ) ;
#30914=( BOUNDED_CURVE ( )  B_SPLINE_CURVE ( 2, ( #4682, #1959, #2300, #9971, #2137, #27680, #15068, #12522, #33304, #12685, #18432 ),
 .UNSPECIFIED., .F., .F. ) 
 B_SPLINE_CURVE_WITH_KNOTS ( ( 3, 2, 2, 2, 2, 3 ),
 ( 0.6428571428571427937, 0.6464285714285713524, 0.6499999999999999112, 0.6535714285714285809, 0.6571428571428571397, 0.6607142857142856984 ),
 .UNSPECIFIED. ) 
 CURVE ( )  GEOMETRIC_REPRESENTATION_ITEM ( )  RATIONAL_B_SPLINE_CURVE ( ( 1.000000000000001554, 0.9510565162951518658, 1.000000000000000000, 0.9510565162951534202, 1.000000000000000000, 0.9510565162951534202, 1.000000000000000000, 0.9510565162951534202, 1.000000000000000000, 0.9510565162951534202, 1.000000000000000000 ) ) 
 REPRESENTATION_ITEM ( '' )  );
#30917=EDGE_LOOP ( 'NONE', ( #6685, #33088, #9525, #18122 ) ) ;
#30928=VERTEX_POINT ( 'NONE', #7045 ) ;
#30935=CARTESIAN_POINT ( 'NONE',  ( 82.02499999726879309, 160.0630714827496206, 15.58253174999999402 ) ) ;
#30940=CARTESIAN_POINT ( 'NONE',  ( 45.80000000000000426, 142.6655632788954620, 8.961492836873471646 ) ) ;
#30945=CARTESIAN_POINT ( 'NONE',  ( 59.12499999726881583, 155.0000000000000000, -15.58253175000000823 ) ) ;
#30946=CARTESIAN_POINT ( 'NONE',  ( 72.77499999726882152, 140.1801316387863778, 4.815267126137185549 ) ) ;
#30949=FACE_BOUND ( 'NONE', #12429, .T. ) ;
#30960=CARTESIAN_POINT ( 'NONE',  ( 34.68867513459483831, 150.1262045565065364, -15.00000000000012434 ) ) ;
#30968=CARTESIAN_POINT ( 'NONE',  ( 77.37499999726881583, 155.0000000000000000, -15.58253175000000823 ) ) ;
#30970=ORIENTED_EDGE ( 'NONE', *, *, #9401, .T. ) ;
#30972=CARTESIAN_POINT ( 'NONE',  ( 73.82499999726880446, 168.2552932293087906, 9.630534252274372875 ) ) ;
#30976=CARTESIAN_POINT ( 'NONE',  ( 62.52499999726882152, 140.1801316387863778, 4.815267126137185549 ) ) ;
#30977=CYLINDRICAL_SURFACE ( 'NONE', #2600, 13.00000000000001776 ) ;
#30983=FACE_OUTER_BOUND ( 'NONE', #19306, .T. ) ;
#30987=CARTESIAN_POINT ( 'NONE',  ( 62.78867513459482552, 155.0000000000000000, -15.00000000000002487 ) ) ;
#30991=DIRECTION ( 'NONE',  ( 0.000000000000000000, -0.7071067811865411334, 0.7071067811865540120 ) ) ;
#30993=CARTESIAN_POINT ( 'NONE',  ( 39.12499999726880873, 155.0000000000000000, -15.58253175000000823 ) ) ;
#30999=CARTESIAN_POINT ( 'NONE',  ( 32.50000000000000000, 155.0000000000000000, -15.00000000000002487 ) ) ;
#31002=CARTESIAN_POINT ( 'NONE',  ( 70.39999999453763735, 168.7903194862797420, -4.480746418436745593 ) ) ;
#31005=VECTOR ( 'NONE', #1723, 1000.000000000000000 ) ;
#31007=EDGE_CURVE ( 'NONE', #27265, #7110, #33003, .T. ) ;
#31010=ORIENTED_EDGE ( 'NONE', *, *, #27884, .T. ) ;
#31013=ORIENTED_EDGE ( 'NONE', *, *, #29333, .T. ) ;
#31019=CARTESIAN_POINT ( 'NONE',  ( 61.67499999726881299, 168.2552932293087906, -9.630534252274387086 ) ) ;
#31027=EDGE_CURVE ( 'NONE', #25327, #14208, #31338, .T. ) ;
#31031=CARTESIAN_POINT ( 'NONE',  ( 34.72499999726881015, 140.1801316387863778, -4.815267126137194431 ) ) ;
#31033=DIRECTION ( 'NONE',  ( 1.000000000000000000, 0.000000000000000000, 0.000000000000000000 ) ) ;
#31035=CARTESIAN_POINT ( 'NONE',  ( 53.67499999726879878, 168.2552932293087906, -9.630534252274385310 ) ) ;
#31038=CARTESIAN_POINT ( 'NONE',  ( 34.78867513459482552, 155.0000000000000000, -15.00000000000002487 ) ) ;
#31039=CARTESIAN_POINT ( 'NONE',  ( 78.51132485994280330, 163.8167787843871110, 12.13525491562421621 ) ) ;
#31040=DIRECTION ( 'NONE',  ( 1.000000000000000000, 0.000000000000000000, 0.000000000000000000 ) ) ;
#31041=CARTESIAN_POINT ( 'NONE',  ( 56.49999999453761745, 170.2462022514548323, -7.872454543227099337E-15 ) ) ;
#31047=CARTESIAN_POINT ( 'NONE',  ( 60.71132485994280614, 155.0000000000000000, 15.00000000000001243 ) ) ;
#31054=CARTESIAN_POINT ( 'NONE',  ( 77.87499999726883004, 171.3844434931184253, -7.942151717890134290E-15 ) ) ;
#31058=CARTESIAN_POINT ( 'NONE',  ( 38.27499999726881441, 160.0630714827496206, 15.58253174999999224 ) ) ;
#31060=CARTESIAN_POINT ( 'NONE',  ( 49.22499999726881725, 160.0630714827496206, -15.58253175000000823 ) ) ;
#31065=CARTESIAN_POINT ( 'NONE',  ( 45.87499999726880162, 171.3844434931184253, -7.942151717890132712E-15 ) ) ;
#31069=EDGE_CURVE ( 'NONE', #17976, #7786, #1087, .T. ) ;
#31070=CARTESIAN_POINT ( 'NONE',  ( 65.99999999999998579, 139.7537977485451393, -4.138211985947621020E-15 ) ) ;
#31078=CARTESIAN_POINT ( 'NONE',  ( 68.32499999726881867, 145.8408176439707802, 12.60653300113718345 ) ) ;
#31081=CARTESIAN_POINT ( 'NONE',  ( 37.69999999453763451, 142.6655632788954620, -8.961492836873480528 ) ) ;
#31088=CARTESIAN_POINT ( 'NONE',  ( 85.71132485994282035, 155.0000000000000000, -15.00000000000002487 ) ) ;
#31090=ORIENTED_EDGE ( 'NONE', *, *, #13726, .F. ) ;
#31092=CARTESIAN_POINT ( 'NONE',  ( 127.5000000000000000, 231.4735983853249763, -73.43303922622311575 ) ) ;
#31093=ORIENTED_EDGE ( 'NONE', *, *, #29387, .F. ) ;
#31099=CARTESIAN_POINT ( 'NONE',  ( 80.72499999726881015, 140.1801316387863778, -4.815267126137194431 ) ) ;
#31104=CARTESIAN_POINT ( 'NONE',  ( 51.10000000000000853, 168.7903194862797420, 4.480746418436729606 ) ) ;
#31108=CARTESIAN_POINT ( 'NONE',  ( 54.22499999726881015, 149.9369285172503510, 15.58253174999999580 ) ) ;
#31111=CARTESIAN_POINT ( 'NONE',  ( 60.22499999726880304, 149.9369285172503510, 15.58253174999999580 ) ) ;
#31112=CARTESIAN_POINT ( 'NONE',  ( 68.77499999726880731, 140.1801316387863778, 4.815267126137185549 ) ) ;
#31114=CARTESIAN_POINT ( 'NONE',  ( 46.61132485994281893, 159.8737954434935489, 15.00000000000006040 ) ) ;
#31127=CARTESIAN_POINT ( 'NONE',  ( 77.47499999726878173, 160.0630714827496206, -15.58253175000000823 ) ) ;
#31130=CARTESIAN_POINT ( 'NONE',  ( 68.82499999726880446, 141.7447067706911810, -9.630534252274387086 ) ) ;
#31133=CARTESIAN_POINT ( 'NONE',  ( 61.32499999726881157, 164.1591823560292198, -12.60653300113719766 ) ) ;
#31141=CARTESIAN_POINT ( 'NONE',  ( 45.38867513459482694, 169.2658477444273331, 4.635254915624208216 ) ) ;
#31148=CARTESIAN_POINT ( 'NONE',  ( 35.02499999726880020, 149.9369285172503510, -15.58253175000000823 ) ) ;
#31152=EDGE_CURVE ( 'NONE', #11884, #5188, #9000, .T. ) ;
#31157=CARTESIAN_POINT ( 'NONE',  ( 76.99999999453763166, 155.0000000000000000, 14.49999999999999467 ) ) ;
#31171=CARTESIAN_POINT ( 'NONE',  ( 82.31132485994280046, 169.2658477444273331, 4.635254915624208216 ) ) ;
#31174=CARTESIAN_POINT ( 'NONE',  ( 60.17499999726881299, 164.1591823560292198, 12.60653300113718167 ) ) ;
#31175=ORIENTED_EDGE ( 'NONE', *, *, #6640, .T. ) ;
#31177=VECTOR ( 'NONE', #14743, 1000.000000000000000 ) ;
#31179=DIRECTION ( 'NONE',  ( 1.000000000000000000, 0.000000000000000000, 0.000000000000000000 ) ) ;
#31184=CARTESIAN_POINT ( 'NONE',  ( 79.81132485994281467, 159.8737954434937478, -14.99999999999993072 ) ) ;
#31191=CARTESIAN_POINT ( 'NONE',  ( 86.20000000000000284, 142.6655632788954620, -8.961492836873480528 ) ) ;
#31196=CARTESIAN_POINT ( 'NONE',  ( 55.97499999726881015, 169.8198683612136222, 4.815267126137181997 ) ) ;
#31201=CARTESIAN_POINT ( 'NONE',  ( 42.71132485994280614, 155.0000000000000000, 15.00000000000001243 ) ) ;
#31202=CARTESIAN_POINT ( 'NONE',  ( 65.11132485994281183, 140.7341522555726669, 4.635254915624211769 ) ) ;
#31203=CARTESIAN_POINT ( 'NONE',  ( 55.39999999453763024, 141.2096805137202580, 4.480746418436733158 ) ) ;
#31206=CYLINDRICAL_SURFACE ( 'NONE', #14882, 2.149999999999985256 ) ;
#31211=VECTOR ( 'NONE', #28835, 1000.000000000000000 ) ;
#31223=CARTESIAN_POINT ( 'NONE',  ( 44.07499999726881157, 168.2552932293087906, 9.630534252274372875 ) ) ;
#31225=CARTESIAN_POINT ( 'NONE',  ( 48.72499999726881725, 140.1801316387863778, -4.815267126137194431 ) ) ;
#31231=CARTESIAN_POINT ( 'NONE',  ( 51.97499999726881725, 169.8198683612136222, 4.815267126137181997 ) ) ;
#31234=LINE ( 'NONE', #21321, #31729 ) ;
#31235=CARTESIAN_POINT ( 'NONE',  ( 64.79999999999998295, 167.3344367211045096, -8.961492836873482304 ) ) ;
#31243=CARTESIAN_POINT ( 'NONE',  ( 70.92499999726881299, 145.8408176439707802, -12.60653300113719588 ) ) ;
#31246=CARTESIAN_POINT ( 'NONE',  ( 88.07499999726879025, 168.2552932293087906, 9.630534252274372875 ) ) ;
#31249=ORIENTED_EDGE ( 'NONE', *, *, #8459, .T. ) ;
#31258=CARTESIAN_POINT ( 'NONE',  ( 125.5000000000000000, 78.52640161467553526, 73.43303922622362734 ) ) ;
#31269=CARTESIAN_POINT ( 'NONE',  ( 85.62499999726880162, 171.3844434931184253, -7.942151717890132712E-15 ) ) ;
#31272=DIRECTION ( 'NONE',  ( 1.000000000000000000, 0.000000000000000000, 0.000000000000000000 ) ) ;
#31275=CARTESIAN_POINT ( 'NONE',  ( 46.50000000000000000, 155.0000000000000000, -14.50000000000000711 ) ) ;
#31278=CARTESIAN_POINT ( 'NONE',  ( 49.72499999726881725, 169.8198683612136222, 4.815267126137181997 ) ) ;
#31281=CARTESIAN_POINT ( 'NONE',  ( 58.72499999726881015, 140.1801316387863778, -4.815267126137194431 ) ) ;
#31282=CARTESIAN_POINT ( 'NONE',  ( 67.27499999726879309, 149.9369285172503510, -15.58253175000000823 ) ) ;
#31284=CARTESIAN_POINT ( 'NONE',  ( 32.50000000000000000, 155.0000000000000000, -6.938893903907228378E-15 ) ) ;
#31301=CARTESIAN_POINT ( 'NONE',  ( 76.82499999726881867, 141.7447067706911810, -9.630534252274387086 ) ) ;
#31304=CARTESIAN_POINT ( 'NONE',  ( 62.62499999726881583, 138.6155565068815463, -3.929120461958505118E-15 ) ) ;
#31307=ORIENTED_EDGE ( 'NONE', *, *, #3214, .T. ) ;
#31317=CARTESIAN_POINT ( 'NONE',  ( 43.78867513459481842, 155.0000000000000000, 15.00000000000001243 ) ) ;
#31319=CARTESIAN_POINT ( 'NONE',  ( 35.42499999726880588, 168.2552932293087906, -9.630534252274387086 ) ) ;
#31326=CARTESIAN_POINT ( 'NONE',  ( 81.49999999453761745, 139.7537977485451393, -4.138211985947621020E-15 ) ) ;
#31331=ORIENTED_EDGE ( 'NONE', *, *, #18464, .F. ) ;
#31333=VERTEX_POINT ( 'NONE', #14445 ) ;
#31334=ORIENTED_EDGE ( 'NONE', *, *, #12823, .T. ) ;
#31338=( BOUNDED_CURVE ( )  B_SPLINE_CURVE ( 2, ( #12652, #2782, #15713, #20671, #18110, #15546, #4655, #26114, #7894, #5158, #18275 ),
 .UNSPECIFIED., .F., .T. ) 
 B_SPLINE_CURVE_WITH_KNOTS ( ( 3, 2, 2, 2, 2, 3 ),
 ( 0.8035714285714286031, 0.8071428571428571619, 0.8107142857142857206, 0.8142857142857143904, 0.8178571428571429491, 0.8214285714285715079 ),
 .UNSPECIFIED. ) 
 CURVE ( )  GEOMETRIC_REPRESENTATION_ITEM ( )  RATIONAL_B_SPLINE_CURVE ( ( 1.000000000000000000, 0.9510565162951534202, 1.000000000000000000, 0.9510565162951534202, 1.000000000000000000, 0.9510565162951534202, 1.000000000000000000, 0.9510565162951534202, 1.000000000000000000, 0.9510565162951518658, 1.000000000000001554 ) ) 
 REPRESENTATION_ITEM ( '' )  );
#31340=EDGE_CURVE ( 'NONE', #19849, #12770, #24839, .T. ) ;
#31342=CARTESIAN_POINT ( 'NONE',  ( 64.27499999726880731, 160.0630714827496206, 15.58253174999999224 ) ) ;
#31345=( NAMED_UNIT ( * ) PLANE_ANGLE_UNIT ( ) SI_UNIT ( $, .RADIAN. ) );
#31346=CYLINDRICAL_SURFACE ( 'NONE', #3845, 15.00000000000001776 ) ;
#31349=FACE_OUTER_BOUND ( 'NONE', #31734, .T. ) ;
#31354=CARTESIAN_POINT ( 'NONE',  ( 84.80000000000001137, 167.3344367211045096, -8.961492836873482304 ) ) ;
#31358=CARTESIAN_POINT ( 'NONE',  ( 63.78867513459482552, 155.0000000000000000, 15.00000000000001243 ) ) ;
#31359=CARTESIAN_POINT ( 'NONE',  ( 56.67499999726881299, 141.7447067706911810, 9.630534252274376428 ) ) ;
#31363=CARTESIAN_POINT ( 'NONE',  ( 87.12499999726880162, 155.0000000000000000, -15.58253175000000823 ) ) ;
#31365=CARTESIAN_POINT ( 'NONE',  ( 54.78867513459483263, 155.0000000000000000, -15.00000000000002487 ) ) ;
#31367=CARTESIAN_POINT ( 'NONE',  ( 59.09999999453762598, 150.2886644046228639, 14.49999999999999645 ) ) ;
#31371=CARTESIAN_POINT ( 'NONE',  ( 32.50000000000000000, 155.0000000000000000, -6.938893903907228378E-15 ) ) ;
#31373=EDGE_LOOP ( 'NONE', ( #7790, #29691, #33626, #1744 ) ) ;
#31383=CARTESIAN_POINT ( 'NONE',  ( 44.77499999726881441, 140.1801316387863778, 4.815267126137185549 ) ) ;
#31385=CARTESIAN_POINT ( 'NONE',  ( 53.32499999726881157, 164.1591823560292198, -12.60653300113719766 ) ) ;
#31388=VECTOR ( 'NONE', #19051, 1000.000000000000000 ) ;
#31390=CARTESIAN_POINT ( 'NONE',  ( 50.47499999726880304, 149.9369285172503510, 15.58253174999999580 ) ) ;
#31393=CARTESIAN_POINT ( 'NONE',  ( 43.88867513459482694, 150.1262045565064227, 15.00000000000001599 ) ) ;
#31396=CARTESIAN_POINT ( 'NONE',  ( 66.10000000000000853, 141.2096805137202580, -4.480746418436742040 ) ) ;
#31400=CARTESIAN_POINT ( 'NONE',  ( 85.78867513459481131, 155.0000000000000000, 15.00000000000001243 ) ) ;
#31401=CARTESIAN_POINT ( 'NONE',  ( 39.37499999726880873, 155.0000000000000000, -15.58253175000000823 ) ) ;
#31403=CARTESIAN_POINT ( 'NONE',  ( 71.92499999726881299, 164.1591823560292198, 12.60653300113718167 ) ) ;
#31406=CARTESIAN_POINT ( 'NONE',  ( 41.69999999453762740, 142.6655632788954620, -8.961492836873480528 ) ) ;
#31412=VERTEX_POINT ( 'NONE', #9333 ) ;
#31425=CARTESIAN_POINT ( 'NONE',  ( 56.11132485994280472, 169.2658477444273331, -4.635254915624224203 ) ) ;
#31427=DIRECTION ( 'NONE',  ( 0.000000000000000000, 0.000000000000000000, -1.000000000000000000 ) ) ;
#31429=CARTESIAN_POINT ( 'NONE',  ( 36.37499999726881583, 155.0000000000000000, 15.58253174999999402 ) ) ;
#31434=CARTESIAN_POINT ( 'NONE',  ( 50.29999999999999716, 146.4771138417591203, -11.73074641843674470 ) ) ;
#31441=CARTESIAN_POINT ( 'NONE',  ( 50.32499999726881157, 145.8408176439707802, 12.60653300113718345 ) ) ;
#31444=CARTESIAN_POINT ( 'NONE',  ( 66.22499999726879594, 149.9369285172503510, 15.58253174999999580 ) ) ;
#31445=CARTESIAN_POINT ( 'NONE',  ( 70.37499999726881583, 155.0000000000000000, 15.58253174999999402 ) ) ;
#31447=CARTESIAN_POINT ( 'NONE',  ( 49.31132485994280756, 140.7341522555726669, -4.635254915624220651 ) ) ;
#31454=CARTESIAN_POINT ( 'NONE',  ( 68.51132485994280330, 163.8167787843871110, 12.13525491562421621 ) ) ;
#31459=CIRCLE ( 'NONE', #9118, 2.149999999999985256 ) ;
#31462=ORIENTED_EDGE ( 'NONE', *, *, #25842, .F. ) ;
#31466=CARTESIAN_POINT ( 'NONE',  ( 76.32499999726881867, 145.8408176439707802, 12.60653300113718345 ) ) ;
#31468=FACE_OUTER_BOUND ( 'NONE', #19835, .T. ) ;
#31470=CARTESIAN_POINT ( 'NONE',  ( 69.42499999726881299, 168.2552932293087906, -9.630534252274385310 ) ) ;
#31486=CARTESIAN_POINT ( 'NONE',  ( 42.42499999726881299, 141.7447067706911810, 9.630534252274376428 ) ) ;
#31494=CARTESIAN_POINT ( 'NONE',  ( 81.29999999453762882, 142.6655632788954620, 8.961492836873471646 ) ) ;
#31498=CARTESIAN_POINT ( 'NONE',  ( 49.68867513459482410, 159.8737954434933499, 15.00000000000019895 ) ) ;
#31504=VECTOR ( 'NONE', #9545, 1000.000000000000000 ) ;
#31509=CARTESIAN_POINT ( 'NONE',  ( 64.97499999726881015, 140.1801316387863778, -4.815267126137194431 ) ) ;
#31511=VERTEX_POINT ( 'NONE', #30805 ) ;
#31517=CARTESIAN_POINT ( 'NONE',  ( 81.47499999726879594, 160.0630714827496206, -15.58253175000000823 ) ) ;
#31520=CARTESIAN_POINT ( 'NONE',  ( 35.62499999726880873, 171.3844434931184253, -7.942151717890132712E-15 ) ) ;
#31521=CARTESIAN_POINT ( 'NONE',  ( 52.71132485994279904, 155.0000000000000000, 15.00000000000001243 ) ) ;
#31525=CARTESIAN_POINT ( 'NONE',  ( 64.08867513459483689, 142.2402378747194405, 9.270509831248432420 ) ) ;
#31526=CARTESIAN_POINT ( 'NONE',  ( 57.47499999726879594, 160.0630714827496206, -15.58253175000000823 ) ) ;
#31531=CARTESIAN_POINT ( 'NONE',  ( 63.59999999453764019, 141.2096805137202580, -4.480746418436742040 ) ) ;
#31539=( BOUNDED_CURVE ( )  B_SPLINE_CURVE ( 2, ( #18326, #15091, #20886, #105, #22767, #5209, #5045, #28388, #15435, #31114, #20546 ),
 .UNSPECIFIED., .F., .T. ) 
 B_SPLINE_CURVE_WITH_KNOTS ( ( 3, 2, 2, 2, 2, 3 ),
 ( 0.2142857142857143293, 0.2178571428571429158, 0.2214285714285714746, 0.2250000000000000611, 0.2285714285714286198, 0.2321428571428572063 ),
 .UNSPECIFIED. ) 
 CURVE ( )  GEOMETRIC_REPRESENTATION_ITEM ( )  RATIONAL_B_SPLINE_CURVE ( ( 0.9999999999999992228, 0.9510565162951541973, 1.000000000000000000, 0.9510565162951534202, 1.000000000000000000, 0.9510565162951534202, 1.000000000000000000, 0.9510565162951534202, 1.000000000000000000, 0.9510565162951526430, 1.000000000000000666 ) ) 
 REPRESENTATION_ITEM ( '' )  );
#31542=CARTESIAN_POINT ( 'NONE',  ( 44.01132485994281751, 167.7597621252805880, -9.270509831248443078 ) ) ;
#31543=ORIENTED_EDGE ( 'NONE', *, *, #16594, .T. ) ;
#31547=CARTESIAN_POINT ( 'NONE',  ( 45.87499999726880162, 171.3844434931184253, -7.942151717890134290E-15 ) ) ;
#31549=CARTESIAN_POINT ( 'NONE',  ( 48.82499999726880446, 141.7447067706911810, -9.630534252274385310 ) ) ;
#31553=CARTESIAN_POINT ( 'NONE',  ( 52.07499999726881157, 168.2552932293087906, 9.630534252274372875 ) ) ;
#31557=CARTESIAN_POINT ( 'NONE',  ( 76.09999999999999432, 141.2096805137202580, -4.480746418436742040 ) ) ;
#31561=CARTESIAN_POINT ( 'NONE',  ( 57.38867513459481984, 169.2658477444273331, 4.635254915624208216 ) ) ;
#31562=CARTESIAN_POINT ( 'NONE',  ( 40.67499999726880588, 141.7447067706911810, 9.630534252274376428 ) ) ;
#31564=CARTESIAN_POINT ( 'NONE',  ( 68.22499999726881015, 149.9369285172503510, 15.58253174999999580 ) ) ;
#31567=CARTESIAN_POINT ( 'NONE',  ( 42.19999999453762740, 163.5228861582408797, -11.73074641843674470 ) ) ;
#31571=EDGE_CURVE ( 'NONE', #6338, #29398, #30838, .T. ) ;
#31581=EDGE_CURVE ( 'NONE', #14343, #10137, #16123, .T. ) ;
#31586=CARTESIAN_POINT ( 'NONE',  ( 56.21132485994281325, 170.7719333635740497, -7.904646289410545231E-15 ) ) ;
#31589=CARTESIAN_POINT ( 'NONE',  ( 87.22499999726881015, 160.0630714827496206, -15.58253175000000823 ) ) ;
#31593=CARTESIAN_POINT ( 'NONE',  ( 51.89999999999999858, 141.2096805137202580, 4.480746418436733158 ) ) ;
#31598=CARTESIAN_POINT ( 'NONE',  ( 51.92499999726880588, 164.1591823560292198, 12.60653300113718167 ) ) ;
#31600=CARTESIAN_POINT ( 'NONE',  ( 37.61132485994281183, 150.1262045565063374, -14.99999999999996803 ) ) ;
#31601=CARTESIAN_POINT ( 'NONE',  ( 66.92499999726881299, 145.8408176439707802, -12.60653300113719588 ) ) ;
#31602=CARTESIAN_POINT ( 'NONE',  ( 77.27499999726880731, 149.9369285172503510, -15.58253175000000823 ) ) ;
#31604=CARTESIAN_POINT ( 'NONE',  ( 49.71132485994280614, 155.0000000000000000, -15.00000000000002487 ) ) ;
#31611=AXIS2_PLACEMENT_3D ( 'NONE', #8192, #18899, #21958 ) ;
#31613=CARTESIAN_POINT ( 'NONE',  ( 68.41132485994282320, 167.7597621252805880, 9.270509831248428867 ) ) ;
#31619=VERTEX_POINT ( 'NONE', #5567 ) ;
#31622=ORIENTED_EDGE ( 'NONE', *, *, #13726, .T. ) ;
#31623=CARTESIAN_POINT ( 'NONE',  ( 75.02499999726879309, 149.9369285172503510, -15.58253175000000823 ) ) ;
#31624=FACE_OUTER_BOUND ( 'NONE', #25668, .T. ) ;
#31627=CARTESIAN_POINT ( 'NONE',  ( 71.42499999726879878, 168.2552932293087906, -9.630534252274385310 ) ) ;
#31641=CARTESIAN_POINT ( 'NONE',  ( 43.42499999726881299, 168.2552932293087906, -9.630534252274387086 ) ) ;
#31642=( BOUNDED_CURVE ( )  B_SPLINE_CURVE ( 2, ( #22682, #12462, #31, #4792, #4966, #9739, #10427, #20125, #20799, #4630, #31201 ),
 .UNSPECIFIED., .F., .T. ) 
 B_SPLINE_CURVE_WITH_KNOTS ( ( 3, 2, 2, 2, 2, 3 ),
 ( 0.1428571428571428492, 0.1464285714285714357, 0.1499999999999999944, 0.1535714285714285532, 0.1571428571428571119, 0.1607142857142856984 ),
 .UNSPECIFIED. ) 
 CURVE ( )  GEOMETRIC_REPRESENTATION_ITEM ( )  RATIONAL_B_SPLINE_CURVE ( ( 1.000000000000000000, 0.9510565162951534202, 1.000000000000000000, 0.9510565162951534202, 1.000000000000000000, 0.9510565162951534202, 1.000000000000000000, 0.9510565162951534202, 1.000000000000000000, 0.9510565162951537532, 0.9999999999999996669 ) ) 
 REPRESENTATION_ITEM ( '' )  );
#31649=AXIS2_PLACEMENT_3D ( 'NONE', #556, #29671, #5819 ) ;
#31650=CARTESIAN_POINT ( 'NONE',  ( 78.09999999453762598, 159.7113355953771077, -14.50000000000000888 ) ) ;
#31659=VERTEX_POINT ( 'NONE', #20742 ) ;
#31661=EDGE_CURVE ( 'NONE', #20912, #14808, #21026, .T. ) ;
#31662=CARTESIAN_POINT ( 'NONE',  ( 74.07499999726881867, 168.2552932293087906, 9.630534252274372875 ) ) ;
#31666=EDGE_CURVE ( 'NONE', #31659, #19344, #5728, .T. ) ;
#31669=CARTESIAN_POINT ( 'NONE',  ( 63.97499999726881725, 169.8198683612136222, 4.815267126137181997 ) ) ;
#31671=CARTESIAN_POINT ( 'NONE',  ( 36.41132485994280898, 167.7597621252805880, 9.270509831248428867 ) ) ;
#31677=CARTESIAN_POINT ( 'NONE',  ( 87.37499999726880162, 155.0000000000000000, -15.58253175000000823 ) ) ;
#31680=CARTESIAN_POINT ( 'NONE',  ( 41.72499999726881015, 169.8198683612136222, 4.815267126137181997 ) ) ;
#31684=CARTESIAN_POINT ( 'NONE',  ( 58.27499999726880731, 160.0630714827496206, 15.58253174999999402 ) ) ;
#31688=DIRECTION ( 'NONE',  ( 0.000000000000000000, -0.7071067811865506814, -0.7071067811865442421 ) ) ;
#31691=CARTESIAN_POINT ( 'NONE',  ( 60.99999999453763166, 155.0000000000000000, 14.49999999999999467 ) ) ;
#31696=CARTESIAN_POINT ( 'NONE',  ( 70.78867513459482552, 155.0000000000000000, -15.00000000000002487 ) ) ;
#31707=DIRECTION ( 'NONE',  ( 0.000000000000000000, 0.000000000000000000, -1.000000000000000000 ) ) ;
#31709=CARTESIAN_POINT ( 'NONE',  ( 42.57499999726881157, 145.8408176439707802, 12.60653300113718345 ) ) ;
#31711=CARTESIAN_POINT ( 'NONE',  ( 47.62499999726880162, 171.3844434931184253, -7.942151717890132712E-15 ) ) ;
#31712=CARTESIAN_POINT ( 'NONE',  ( 32.50000000000000000, 155.0000000000000000, -15.00000000000002487 ) ) ;
#31715=CARTESIAN_POINT ( 'NONE',  ( 56.67499999726881299, 141.7447067706911810, 9.630534252274376428 ) ) ;
#31717=CARTESIAN_POINT ( 'NONE',  ( 47.68867513459483831, 159.8737954434934920, 15.00000000000010836 ) ) ;
#31719=CARTESIAN_POINT ( 'NONE',  ( 75.19999999999998863, 167.3344367211045096, 8.961492836873468093 ) ) ;
#31724=CARTESIAN_POINT ( 'NONE',  ( 39.97499999726881015, 169.8198683612136222, 4.815267126137181997 ) ) ;
#31726=CARTESIAN_POINT ( 'NONE',  ( 78.52499999726880731, 140.1801316387863778, 4.815267126137185549 ) ) ;
#31727=VERTEX_POINT ( 'NONE', #2701 ) ;
#31729=VECTOR ( 'NONE', #2615, 1000.000000000000000 ) ;
#31730=CARTESIAN_POINT ( 'NONE',  ( 44.29999999453762882, 167.3344367211045096, -8.961492836873482304 ) ) ;
#31734=EDGE_LOOP ( 'NONE', ( #28356, #9369, #3075, #18919 ) ) ;
#31743=EDGE_LOOP ( 'NONE', ( #31770, #7199 ) ) ;
#31751=AXIS2_PLACEMENT_3D ( 'NONE', #904, #29524, #3799 ) ;
#31752=CARTESIAN_POINT ( 'NONE',  ( 36.67499999726879878, 141.7447067706911810, 9.630534252274376428 ) ) ;
#31757=CARTESIAN_POINT ( 'NONE',  ( 53.29999999999999716, 163.5228861582408797, 11.73074641843673049 ) ) ;
#31760=CARTESIAN_POINT ( 'NONE',  ( 60.62499999726879452, 138.6155565068815463, -3.929120461958505118E-15 ) ) ;
#31764=CARTESIAN_POINT ( 'NONE',  ( 36.81132485994281467, 150.1262045565063943, 14.99999999999997691 ) ) ;
#31765=CARTESIAN_POINT ( 'NONE',  ( 64.92499999726881299, 145.8408176439707802, -12.60653300113719588 ) ) ;
#31766=CARTESIAN_POINT ( 'NONE',  ( 74.47499999726881015, 149.9369285172503510, 15.58253174999999580 ) ) ;
#31770=ORIENTED_EDGE ( 'NONE', *, *, #7424, .F. ) ;
#31779=VERTEX_POINT ( 'NONE', #13078 ) ;
#31785=CARTESIAN_POINT ( 'NONE',  ( 80.82499999726880446, 141.7447067706911810, -9.630534252274387086 ) ) ;
#31788=CARTESIAN_POINT ( 'NONE',  ( 69.12499999726881583, 155.0000000000000000, -15.58253175000000823 ) ) ;
#31793=CARTESIAN_POINT ( 'NONE',  ( 32.60000000000000853, 159.7113355953771077, -14.50000000000000888 ) ) ;
#31802=CARTESIAN_POINT ( 'NONE',  ( 46.12499999726880873, 155.0000000000000000, 15.58253174999999402 ) ) ;
#31809=CARTESIAN_POINT ( 'NONE',  ( 81.19999999453763451, 146.4771138417591203, 11.73074641843673227 ) ) ;
#31814=FACE_OUTER_BOUND ( 'NONE', #22783, .T. ) ;
#31821=CARTESIAN_POINT ( 'NONE',  ( 77.37499999726881583, 155.0000000000000000, -15.58253175000000823 ) ) ;
#31827=CARTESIAN_POINT ( 'NONE',  ( 72.37499999726881583, 155.0000000000000000, 15.58253174999999402 ) ) ;
#31829=CARTESIAN_POINT ( 'NONE',  ( 41.18867513459483121, 169.2658477444273331, -4.635254915624224203 ) ) ;
#31837=CARTESIAN_POINT ( 'NONE',  ( 84.57499999726880446, 145.8408176439707802, 12.60653300113718345 ) ) ;
#31839=CARTESIAN_POINT ( 'NONE',  ( 36.32499999726881157, 145.8408176439707802, 12.60653300113718345 ) ) ;
#31844=CARTESIAN_POINT ( 'NONE',  ( 59.47499999726879594, 160.0630714827496206, -15.58253175000000823 ) ) ;
#31852=CARTESIAN_POINT ( 'NONE',  ( 62.49999999453763166, 170.2462022514548323, -7.872454543227099337E-15 ) ) ;
#31858=FACE_OUTER_BOUND ( 'NONE', #24023, .T. ) ;
#31859=EDGE_LOOP ( 'NONE', ( #30708, #10608, #7080, #21146, #10447 ) ) ;
#31861=ADVANCED_FACE ( 'NONE', ( #1127 ), #23279, .F. ) ;
#31869=CARTESIAN_POINT ( 'NONE',  ( 49.17499999726881299, 145.8408176439707802, -12.60653300113719588 ) ) ;
#31871=CARTESIAN_POINT ( 'NONE',  ( 58.02499999726880731, 160.0630714827496206, 15.58253174999999402 ) ) ;
#31876=CARTESIAN_POINT ( 'NONE',  ( 52.87499999726880162, 138.6155565068815463, -3.929120461958505118E-15 ) ) ;
#31878=CARTESIAN_POINT ( 'NONE',  ( 47.38867513459482694, 169.2658477444273331, 4.635254915624208216 ) ) ;
#31880=ADVANCED_FACE ( 'NONE', ( #20467 ), #20968, .F. ) ;
#31882=CARTESIAN_POINT ( 'NONE',  ( 71.29999999999999716, 163.5228861582408797, 11.73074641843673049 ) ) ;
#31883=CARTESIAN_POINT ( 'NONE',  ( 62.01132485994281751, 167.7597621252805880, -9.270509831248443078 ) ) ;
#31887=CARTESIAN_POINT ( 'NONE',  ( 35.27499999726881441, 149.9369285172503510, -15.58253175000000823 ) ) ;
#31889=CARTESIAN_POINT ( 'NONE',  ( 74.72499999726881015, 140.1801316387863778, -4.815267126137194431 ) ) ;
#31892=CARTESIAN_POINT ( 'NONE',  ( 38.89999999453763024, 159.7113355953771077, 14.49999999999999289 ) ) ;
#31901=ORIENTED_EDGE ( 'NONE', *, *, #26464, .F. ) ;
#31904=CARTESIAN_POINT ( 'NONE',  ( 51.41132485994281609, 142.2402378747194405, -9.270509831248439525 ) ) ;
#31911=CARTESIAN_POINT ( 'NONE',  ( 33.12499999726880873, 155.0000000000000000, -15.58253175000000823 ) ) ;
#31913=CARTESIAN_POINT ( 'NONE',  ( 36.47499999726881015, 149.9369285172503510, 15.58253174999999580 ) ) ;
#31917=CARTESIAN_POINT ( 'NONE',  ( 54.30000000000000426, 146.4771138417591203, -11.73074641843674470 ) ) ;
#31922=CARTESIAN_POINT ( 'NONE',  ( 57.72499999726881015, 169.8198683612136222, 4.815267126137181997 ) ) ;
#31924=DIRECTION ( 'NONE',  ( 1.000000000000000000, 0.000000000000000000, 0.000000000000000000 ) ) ;
#31925=CARTESIAN_POINT ( 'NONE',  ( 63.12499999726880873, 155.0000000000000000, -15.58253175000000823 ) ) ;
#31926=CARTESIAN_POINT ( 'NONE',  ( 77.97499999726881015, 169.8198683612136222, 4.815267126137181997 ) ) ;
#31939=ADVANCED_FACE ( 'NONE', ( #33584 ), #7864, .T. ) ;
#31940=VERTEX_POINT ( 'NONE', #31038 ) ;
#31947=AXIS2_PLACEMENT_3D ( 'NONE', #2838, #23622, #13225 ) ;
#31948=CARTESIAN_POINT ( 'NONE',  ( 78.02499999726879309, 160.0630714827496206, 15.58253174999999224 ) ) ;
#31949=VERTEX_POINT ( 'NONE', #8032 ) ;
#31952=CARTESIAN_POINT ( 'NONE',  ( 71.12499999726881583, 155.0000000000000000, -15.58253175000000823 ) ) ;
#31957=CARTESIAN_POINT ( 'NONE',  ( 34.70000000000000284, 163.5228861582408797, -11.73074641843674470 ) ) ;
#31964=CARTESIAN_POINT ( 'NONE',  ( 60.18867513459482410, 140.7341522555726669, 4.635254915624211769 ) ) ;
#31965=CARTESIAN_POINT ( 'NONE',  ( 47.32499999726881867, 164.1591823560292198, -12.60653300113719766 ) ) ;
#31967=CARTESIAN_POINT ( 'NONE',  ( 32.50000000000000000, 155.0000000000000000, 15.00000000000001243 ) ) ;
#31975=CARTESIAN_POINT ( 'NONE',  ( 88.19999999453763451, 163.5228861582408797, -11.73074641843674470 ) ) ;
#31978=( BOUNDED_CURVE ( )  B_SPLINE_CURVE ( 2, ( #10065, #5601, #26216, #10400, #33557, #30840, #15825, #10233, #2557, #18556, #25716 ),
 .UNSPECIFIED., .F., .T. ) 
 B_SPLINE_CURVE_WITH_KNOTS ( ( 3, 2, 2, 2, 2, 3 ),
 ( 0.5535714285714284921, 0.5571428571428570509, 0.5607142857142856096, 0.5642857142857142794, 0.5678571428571428381, 0.5714285714285713969 ),
 .UNSPECIFIED. ) 
 CURVE ( )  GEOMETRIC_REPRESENTATION_ITEM ( )  RATIONAL_B_SPLINE_CURVE ( ( 1.000000000000001554, 0.9510565162951518658, 1.000000000000000000, 0.9510565162951534202, 1.000000000000000000, 0.9510565162951534202, 1.000000000000000000, 0.9510565162951534202, 1.000000000000000000, 0.9510565162951534202, 1.000000000000000000 ) ) 
 REPRESENTATION_ITEM ( '' )  );
#31983=VERTEX_POINT ( 'NONE', #5131 ) ;
#31988=CARTESIAN_POINT ( 'NONE',  ( 75.47499999726881015, 160.0630714827496206, -15.58253175000000823 ) ) ;
#31990=EDGE_CURVE ( 'NONE', #3282, #12765, #14112, .T. ) ;
#31997=CARTESIAN_POINT ( 'NONE',  ( 67.07499999726880446, 141.7447067706911810, -9.630534252274387086 ) ) ;
#31999=CARTESIAN_POINT ( 'NONE',  ( 62.18867513459482410, 140.7341522555726669, 4.635254915624211769 ) ) ;
#32007=CARTESIAN_POINT ( 'NONE',  ( 81.77499999726880731, 169.8198683612136222, -4.815267126137197984 ) ) ;
#32011=CARTESIAN_POINT ( 'NONE',  ( 39.72499999726881015, 169.8198683612136222, 4.815267126137181997 ) ) ;
#32015=CARTESIAN_POINT ( 'NONE',  ( 64.07499999726881867, 168.2552932293087906, 9.630534252274372875 ) ) ;
#32023=CARTESIAN_POINT ( 'NONE',  ( 61.09999999453762598, 150.2886644046228639, 14.49999999999999645 ) ) ;
#32027=CARTESIAN_POINT ( 'NONE',  ( 37.38867513459481984, 169.2658477444273331, 4.635254915624208216 ) ) ;
#32030=CARTESIAN_POINT ( 'NONE',  ( 59.01132485994281751, 142.2402378747194405, 9.270509831248432420 ) ) ;
#32036=DIRECTION ( 'NONE',  ( 0.000000000000000000, -0.000000000000000000, -1.000000000000000000 ) ) ;
#32040=ADVANCED_FACE ( 'NONE', ( #7533 ), #17740, .T. ) ;
#32041=CYLINDRICAL_SURFACE ( 'NONE', #10718, 15.00000000000001776 ) ;
#32043=CARTESIAN_POINT ( 'NONE',  ( 52.17499999726880588, 164.1591823560292198, 12.60653300113718167 ) ) ;
#32045=CARTESIAN_POINT ( 'NONE',  ( 57.52499999726881441, 169.8198683612136222, -4.815267126137197984 ) ) ;
#32051=CARTESIAN_POINT ( 'NONE',  ( 60.77499999726881441, 140.1801316387863778, 4.815267126137185549 ) ) ;
#32053=CARTESIAN_POINT ( 'NONE',  ( 72.88867513459481984, 159.8737954434938615, -14.99999999999984190 ) ) ;
#32056=CARTESIAN_POINT ( 'NONE',  ( 72.59999999999996589, 159.7113355953771077, -14.50000000000000888 ) ) ;
#32057=CARTESIAN_POINT ( 'NONE',  ( 125.5000000000000000, 157.1499999999996362, -106.0000000000000284 ) ) ;
#32060=CARTESIAN_POINT ( 'NONE',  ( 33.48867513459482836, 167.7597621252805880, 9.270509831248428867 ) ) ;
#32061=CARTESIAN_POINT ( 'NONE',  ( 43.97499999726881015, 169.8198683612136222, 4.815267126137181997 ) ) ;
#32065=CARTESIAN_POINT ( 'NONE',  ( 74.82499999726881867, 141.7447067706911810, -9.630534252274385310 ) ) ;
#32068=CARTESIAN_POINT ( 'NONE',  ( 44.19999999453762740, 163.5228861582408797, -11.73074641843674470 ) ) ;
#32072=ORIENTED_EDGE ( 'NONE', *, *, #12430, .T. ) ;
#32074=CARTESIAN_POINT ( 'NONE',  ( 52.78867513459482552, 155.0000000000000000, -15.00000000000002487 ) ) ;
#32079=CARTESIAN_POINT ( 'NONE',  ( 51.71132485994281325, 155.0000000000000000, -15.00000000000002487 ) ) ;
#32086=CARTESIAN_POINT ( 'NONE',  ( 39.62499999726880162, 171.3844434931184253, -7.942151717890132712E-15 ) ) ;
#32088=CARTESIAN_POINT ( 'NONE',  ( 37.67499999726881299, 168.2552932293087906, -9.630534252274385310 ) ) ;
#32092=CARTESIAN_POINT ( 'NONE',  ( 51.50000000000000711, 155.0000000000000000, 14.49999999999999467 ) ) ;
#32094=CARTESIAN_POINT ( 'NONE',  ( 75.71132485994280614, 155.0000000000000000, -15.00000000000002487 ) ) ;
#32095=CARTESIAN_POINT ( 'NONE',  ( 56.72499999726881015, 140.1801316387863778, -4.815267126137194431 ) ) ;
#32097=ORIENTED_EDGE ( 'NONE', *, *, #24751, .T. ) ;
#32099=CARTESIAN_POINT ( 'NONE',  ( 66.02499999726879309, 160.0630714827496206, 15.58253174999999224 ) ) ;
#32100=CARTESIAN_POINT ( 'NONE',  ( 79.17499999726881299, 145.8408176439707802, -12.60653300113719588 ) ) ;
#32103=CARTESIAN_POINT ( 'NONE',  ( 83.98867513459481415, 146.1832212156128890, 12.13525491562421976 ) ) ;
#32114=ORIENTED_EDGE ( 'NONE', *, *, #20169, .F. ) ;
#32118=CARTESIAN_POINT ( 'NONE',  ( 84.62499999726880162, 138.6155565068815747, -3.929120461958505118E-15 ) ) ;
#32121=CARTESIAN_POINT ( 'NONE',  ( 68.62499999726880162, 138.6155565068815463, -3.929120461958505118E-15 ) ) ;
#32127=CARTESIAN_POINT ( 'NONE',  ( 37.80000000000000426, 142.6655632788954620, 8.961492836873471646 ) ) ;
#32135=CARTESIAN_POINT ( 'NONE',  ( 45.62499999726880162, 171.3844434931184253, -7.942151717890134290E-15 ) ) ;
#32142=CARTESIAN_POINT ( 'NONE',  ( 87.89999999453760893, 150.2886644046228639, -14.50000000000000888 ) ) ;
#32150=ORIENTED_EDGE ( 'NONE', *, *, #17637, .T. ) ;
#32151=CARTESIAN_POINT ( 'NONE',  ( 71.17499999726881299, 145.8408176439707802, -12.60653300113719588 ) ) ;
#32154=CARTESIAN_POINT ( 'NONE',  ( 76.87499999726881583, 138.6155565068815747, -3.929120461958505118E-15 ) ) ;
#32158=LINE ( 'NONE', #32329, #31388 ) ;
#32160=CARTESIAN_POINT ( 'NONE',  ( 66.27499999726880731, 160.0630714827496206, 15.58253174999999224 ) ) ;
#32161=EDGE_LOOP ( 'NONE', ( #7846, #1868 ) ) ;
#32162=CARTESIAN_POINT ( 'NONE',  ( 35.81132485994280756, 159.8737954434936626, -15.00000000000000178 ) ) ;
#32170=CARTESIAN_POINT ( 'NONE',  ( 85.97499999726882436, 169.8198683612136222, 4.815267126137181997 ) ) ;
#32171=PRODUCT_CONTEXT ( 'NONE', #16582, 'mechanical' ) ;
#32174=CARTESIAN_POINT ( 'NONE',  ( 44.32499999726881157, 145.8408176439707802, 12.60653300113718345 ) ) ;
#32180=( BOUNDED_CURVE ( )  B_SPLINE_CURVE ( 2, ( #5987, #29670, #24559, #16375, #3104, #32385, #13492, #6322, #1215, #9049, #19441 ),
 .UNSPECIFIED., .F., .T. ) 
 B_SPLINE_CURVE_WITH_KNOTS ( ( 3, 2, 2, 2, 2, 3 ),
 ( 0.8392857142857141906, 0.8428571428571427493, 0.8464285714285714191, 0.8499999999999999778, 0.8535714285714285365, 0.8571428571428570953 ),
 .UNSPECIFIED. ) 
 CURVE ( )  GEOMETRIC_REPRESENTATION_ITEM ( )  RATIONAL_B_SPLINE_CURVE ( ( 1.000000000000000000, 0.9510565162951534202, 1.000000000000000000, 0.9510565162951534202, 1.000000000000000000, 0.9510565162951534202, 1.000000000000000000, 0.9510565162951534202, 1.000000000000000000, 0.9510565162951534202, 1.000000000000000000 ) ) 
 REPRESENTATION_ITEM ( '' )  );
#32187=CARTESIAN_POINT ( 'NONE',  ( 63.69999999453762740, 142.6655632788954620, -8.961492836873480528 ) ) ;
#32188=CIRCLE ( 'NONE', #7175, 98.00000000000000000 ) ;
#32193=CARTESIAN_POINT ( 'NONE',  ( 45.71132485994280614, 155.0000000000000000, -15.00000000000002487 ) ) ;
#32204=CARTESIAN_POINT ( 'NONE',  ( 50.67499999726880588, 141.7447067706911810, 9.630534252274376428 ) ) ;
#32206=CARTESIAN_POINT ( 'NONE',  ( 58.52499999726881441, 140.1801316387863778, 4.815267126137185549 ) ) ;
#32211=CARTESIAN_POINT ( 'NONE',  ( 60.37499999726880873, 155.0000000000000000, 15.58253174999999402 ) ) ;
#32213=CARTESIAN_POINT ( 'NONE',  ( 72.98867513459481415, 163.8167787843871110, -12.13525491562423397 ) ) ;
#32216=CARTESIAN_POINT ( 'NONE',  ( 74.50000000000001421, 155.0000000000000000, -14.50000000000000711 ) ) ;
#32220=CARTESIAN_POINT ( 'NONE',  ( 125.5000000000000000, 80.04668119422662187, 74.95331880577468553 ) ) ;
#32221=CARTESIAN_POINT ( 'NONE',  ( 43.27499999726880020, 149.9369285172503510, -15.58253175000000823 ) ) ;
#32223=CARTESIAN_POINT ( 'NONE',  ( 75.42499999726879878, 168.2552932293087906, -9.630534252274385310 ) ) ;
#32228=CARTESIAN_POINT ( 'NONE',  ( 45.29999999453762172, 142.6655632788954620, 8.961492836873471646 ) ) ;
#32247=CARTESIAN_POINT ( 'NONE',  ( 36.92499999726880588, 145.8408176439707802, -12.60653300113719588 ) ) ;
#32250=CARTESIAN_POINT ( 'NONE',  ( 41.17499999726881299, 145.8408176439707802, -12.60653300113719588 ) ) ;
#32253=PRODUCT ( 'air chamber shell front', 'air chamber shell front', '', ( #32171 ) ) ;
#32255=CARTESIAN_POINT ( 'NONE',  ( 51.70000000000000284, 146.4771138417591203, 11.73074641843673227 ) ) ;
#32256=FACE_BOUND ( 'NONE', #21515, .T. ) ;
#32258=CARTESIAN_POINT ( 'NONE',  ( 77.78867513459483973, 155.0000000000000000, 15.00000000000001243 ) ) ;
#32261=CARTESIAN_POINT ( 'NONE',  ( 58.42499999726879878, 141.7447067706911810, 9.630534252274376428 ) ) ;
#32265=CARTESIAN_POINT ( 'NONE',  ( 74.97499999726881015, 140.1801316387863778, -4.815267126137194431 ) ) ;
#32290=ORIENTED_EDGE ( 'NONE', *, *, #24751, .F. ) ;
#32291=CIRCLE ( 'NONE', #2394, 112.0000000000000711 ) ;
#32292=CARTESIAN_POINT ( 'NONE',  ( 81.82499999726879025, 168.2552932293087906, 9.630534252274372875 ) ) ;
#32295=CARTESIAN_POINT ( 'NONE',  ( 74.82499999726881867, 141.7447067706911810, -9.630534252274385310 ) ) ;
#32297=CARTESIAN_POINT ( 'NONE',  ( 87.50000000000001421, 167.6893833810455305, 8.204385406124638180 ) ) ;
#32299=CARTESIAN_POINT ( 'NONE',  ( 36.79999999999999716, 167.3344367211045096, -8.961492836873482304 ) ) ;
#32307=CARTESIAN_POINT ( 'NONE',  ( 48.22499999726881015, 149.9369285172503510, 15.58253174999999580 ) ) ;
#32309=CARTESIAN_POINT ( 'NONE',  ( 41.01132485994281041, 142.2402378747194405, 9.270509831248432420 ) ) ;
#32314=CARTESIAN_POINT ( 'NONE',  ( 83.09999999453761177, 150.2886644046228639, 14.49999999999999645 ) ) ;
#32322=CARTESIAN_POINT ( 'NONE',  ( 73.97499999726881015, 169.8198683612136222, 4.815267126137181997 ) ) ;
#32325=CARTESIAN_POINT ( 'NONE',  ( 83.97499999726882436, 169.8198683612136222, 4.815267126137181997 ) ) ;
#32329=CARTESIAN_POINT ( 'NONE',  ( 125.5000000000000000, 157.1499999999996362, -106.0000000000000284 ) ) ;
#32331=CARTESIAN_POINT ( 'NONE',  ( 71.17499999726881299, 145.8408176439707802, -12.60653300113719588 ) ) ;
#32335=CARTESIAN_POINT ( 'NONE',  ( 51.78867513459482552, 155.0000000000000000, 15.00000000000001243 ) ) ;
#32336=ADVANCED_BREP_SHAPE_REPRESENTATION ( '', ( #789, #2404 ), #8406 ) ;
#32341=CARTESIAN_POINT ( 'NONE',  ( 37.81132485994280756, 159.8737954434935489, -15.00000000000008527 ) ) ;
#32345=CARTESIAN_POINT ( 'NONE',  ( 45.72499999726881015, 169.8198683612136222, 4.815267126137181997 ) ) ;
#32347=CARTESIAN_POINT ( 'NONE',  ( 33.12499999726880873, 155.0000000000000000, -15.58253175000000823 ) ) ;
#32356=CARTESIAN_POINT ( 'NONE',  ( 67.99999999453761745, 155.0000000000000000, -14.50000000000000711 ) ) ;
#32357=ORIENTED_EDGE ( 'NONE', *, *, #31581, .T. ) ;
#32360=CARTESIAN_POINT ( 'NONE',  ( 74.38867513459481984, 140.7341522555726669, -4.635254915624220651 ) ) ;
#32366=CARTESIAN_POINT ( 'NONE',  ( 58.48867513459484258, 142.2402378747194405, -9.270509831248439525 ) ) ;
#32372=CARTESIAN_POINT ( 'NONE',  ( 52.37499999726881583, 155.0000000000000000, 15.58253174999999402 ) ) ;
#32374=CARTESIAN_POINT ( 'NONE',  ( 55.72499999726881015, 169.8198683612136222, 4.815267126137181997 ) ) ;
#32378=DIRECTION ( 'NONE',  ( 0.000000000000000000, 0.000000000000000000, -1.000000000000000000 ) ) ;
#32380=CARTESIAN_POINT ( 'NONE',  ( 60.47499999726881725, 149.9369285172503510, 15.58253174999999580 ) ) ;
#32384=CARTESIAN_POINT ( 'NONE',  ( 79.69999999999998863, 146.4771138417591203, 11.73074641843673227 ) ) ;
#32385=CARTESIAN_POINT ( 'NONE',  ( 40.28867513459482552, 139.2280666364260071, -4.041636747397287284E-15 ) ) ;
#32388=CYLINDRICAL_SURFACE ( 'NONE', #17278, 15.00000000000001776 ) ;
#32389=CARTESIAN_POINT ( 'NONE',  ( 43.47499999726881015, 160.0630714827496206, -15.58253175000000823 ) ) ;
#32391=CARTESIAN_POINT ( 'NONE',  ( 76.72499999726881015, 140.1801316387863778, -4.815267126137194431 ) ) ;
#32395=CARTESIAN_POINT ( 'NONE',  ( 45.99999999453763166, 155.0000000000000000, -14.50000000000000711 ) ) ;
#32408=DIRECTION ( 'NONE',  ( 1.000000000000000000, 0.000000000000000000, 0.000000000000000000 ) ) ;
#32412=CARTESIAN_POINT ( 'NONE',  ( 38.42499999726879878, 141.7447067706911810, 9.630534252274376428 ) ) ;
#32415=SHAPE_REPRESENTATION ( 'air chamber shell front', ( #2404 ), #8406 ) ;
#32417=CARTESIAN_POINT ( 'NONE',  ( 38.97499999726881015, 140.1801316387863778, -4.815267126137194431 ) ) ;
#32420=CARTESIAN_POINT ( 'NONE',  ( 60.10000000000000142, 141.2096805137202580, -4.480746418436742040 ) ) ;
#32421=DIRECTION ( 'NONE',  ( -1.000000000000000000, 0.000000000000000000, -0.000000000000000000 ) ) ;
#32425=EDGE_CURVE ( 'NONE', #4684, #18787, #11586, .T. ) ;
#32426=CARTESIAN_POINT ( 'NONE',  ( 59.82499999726879736, 168.2552932293087906, 9.630534252274372875 ) ) ;
#32428=EDGE_LOOP ( 'NONE', ( #22615, #26421, #12337, #15016 ) ) ;
#32430=CARTESIAN_POINT ( 'NONE',  ( 83.17499999726882720, 145.8408176439707802, -12.60653300113719588 ) ) ;
#32445=CARTESIAN_POINT ( 'NONE',  ( 63.01132485994281751, 142.2402378747194405, 9.270509831248432420 ) ) ;
#32450=CARTESIAN_POINT ( 'NONE',  ( 82.62499999726881583, 138.6155565068815747, -3.929120461958505118E-15 ) ) ;
#32453=CARTESIAN_POINT ( 'NONE',  ( 78.12499999726883004, 155.0000000000000000, 15.58253174999999402 ) ) ;
#32457=LINE ( 'NONE', #6911, #15669 ) ;
#32460=CARTESIAN_POINT ( 'NONE',  ( 33.70000000000000284, 146.4771138417591203, 11.73074641843673227 ) ) ;
#32462=ADVANCED_FACE ( 'NONE', ( #14634 ), #9692, .T. ) ;
#32465=DIRECTION ( 'NONE',  ( 1.000000000000000000, 0.000000000000000000, 0.000000000000000000 ) ) ;
#32468=CARTESIAN_POINT ( 'NONE',  ( 53.02499999726881441, 149.9369285172503510, -15.58253175000000823 ) ) ;
#32476=CARTESIAN_POINT ( 'NONE',  ( 86.49999999453761745, 170.2462022514548323, -7.872454543227099337E-15 ) ) ;
#32482=FACE_OUTER_BOUND ( 'NONE', #19321, .T. ) ;
#32483=ORIENTED_EDGE ( 'NONE', *, *, #29099, .F. ) ;
#32486=CARTESIAN_POINT ( 'NONE',  ( 68.67499999726879878, 141.7447067706911810, 9.630534252274376428 ) ) ;
#32489=AXIS2_PLACEMENT_3D ( 'NONE', #6876, #33280, #19991 ) ;
#32490=CARTESIAN_POINT ( 'NONE',  ( 82.77499999726880731, 140.1801316387863778, 4.815267126137185549 ) ) ;
#32496=CARTESIAN_POINT ( 'NONE',  ( 71.97499999726881015, 169.8198683612136222, 4.815267126137181997 ) ) ;
#32506=CARTESIAN_POINT ( 'NONE',  ( 88.37499999726880162, 155.0000000000000000, 15.58253174999999402 ) ) ;
#32507=VECTOR ( 'NONE', #17796, 1000.000000000000000 ) ;
#32511=CARTESIAN_POINT ( 'NONE',  ( 45.62499999726880162, 171.3844434931184253, -7.942151717890132712E-15 ) ) ;
#32517=CARTESIAN_POINT ( 'NONE',  ( 76.68867513459481700, 150.1262045565067922, -15.00000000000028599 ) ) ;
#32518=DIRECTION ( 'NONE',  ( 1.000000000000000000, 0.000000000000000000, 0.000000000000000000 ) ) ;
#32521=CARTESIAN_POINT ( 'NONE',  ( 68.89999999453763735, 159.7113355953771077, 14.49999999999999289 ) ) ;
#32522=ORIENTED_EDGE ( 'NONE', *, *, #20142, .F. ) ;
#32531=CARTESIAN_POINT ( 'NONE',  ( 87.49999999999995737, 162.7917165882215329, -13.53300274343441956 ) ) ;
#32537=CARTESIAN_POINT ( 'NONE',  ( 47.37499999726880873, 155.0000000000000000, -15.58253175000000823 ) ) ;
#32538=AXIS2_PLACEMENT_3D ( 'NONE', #4190, #30090, #19863 ) ;
#32541=CARTESIAN_POINT ( 'NONE',  ( 32.50000000000000000, 155.0000000000000000, -15.00000000000002487 ) ) ;
#32545=CARTESIAN_POINT ( 'NONE',  ( 62.37499999726880873, 155.0000000000000000, 15.58253174999999402 ) ) ;
#32547=CARTESIAN_POINT ( 'NONE',  ( 70.08867513459482268, 142.2402378747194405, 9.270509831248432420 ) ) ;
#32550=CARTESIAN_POINT ( 'NONE',  ( 81.79999999999999716, 142.6655632788954620, 8.961492836873471646 ) ) ;
#32556=CARTESIAN_POINT ( 'NONE',  ( 42.87499999726881583, 138.6155565068815463, -3.929120461958505118E-15 ) ) ;
#32560=CARTESIAN_POINT ( 'NONE',  ( 85.52499999726880731, 169.8198683612136222, -4.815267126137197984 ) ) ;
#32564=CARTESIAN_POINT ( 'NONE',  ( 46.79999999453762882, 163.5228861582408797, 11.73074641843673049 ) ) ;
#32567=CARTESIAN_POINT ( 'NONE',  ( 60.81132485994280756, 150.1262045565063659, 14.99999999999997158 ) ) ;
#32569=CARTESIAN_POINT ( 'NONE',  ( 66.01132485994280330, 167.7597621252805880, -9.270509831248443078 ) ) ;
#32570=EDGE_LOOP ( 'NONE', ( #25194, #16481 ) ) ;
#32576=CARTESIAN_POINT ( 'NONE',  ( 51.21132485994281325, 139.2280666364260071, -4.041636747397287284E-15 ) ) ;
#32580=CARTESIAN_POINT ( 'NONE',  ( 32.50000000000000000, 155.0000000000000000, -13.00000000000002487 ) ) ;
#32584=CARTESIAN_POINT ( 'NONE',  ( 36.82499999726881157, 141.7447067706911810, -9.630534252274385310 ) ) ;
#32588=CARTESIAN_POINT ( 'NONE',  ( 61.72499999726881015, 169.8198683612136222, 4.815267126137181997 ) ) ;
#32590=CARTESIAN_POINT ( 'NONE',  ( 39.87499999726880162, 171.3844434931184253, -7.942151717890132712E-15 ) ) ;
#32594=CARTESIAN_POINT ( 'NONE',  ( 63.00000000000000000, 170.2462022514548323, -7.872454543227099337E-15 ) ) ;
#32598=LINE ( 'NONE', #30047, #24339 ) ;
#32600=CARTESIAN_POINT ( 'NONE',  ( 66.52499999726880731, 140.1801316387863778, 4.815267126137185549 ) ) ;
#32604=CARTESIAN_POINT ( 'NONE',  ( 85.77499999726880731, 169.8198683612136222, -4.815267126137197984 ) ) ;
#32617=EDGE_CURVE ( 'NONE', #10137, #14343, #13214, .T. ) ;
#32624=CARTESIAN_POINT ( 'NONE',  ( 83.62499999726881583, 171.3844434931184253, -7.942151717890134290E-15 ) ) ;
#32626=CARTESIAN_POINT ( 'NONE',  ( 69.58867513459482268, 163.8167787843871110, 12.13525491562421621 ) ) ;
#32628=CARTESIAN_POINT ( 'NONE',  ( 78.52499999726880731, 140.1801316387863778, 4.815267126137185549 ) ) ;
#32631=DIRECTION ( 'NONE',  ( -1.000000000000000000, -0.000000000000000000, -0.000000000000000000 ) ) ;
#32633=CARTESIAN_POINT ( 'NONE',  ( 43.99999999999999289, 139.7537977485451393, -4.138211985947621020E-15 ) ) ;
#32637=CARTESIAN_POINT ( 'NONE',  ( 73.51132485994280330, 146.1832212156128890, -12.13525491562423042 ) ) ;
#32638=LINE ( 'NONE', #9301, #18608 ) ;
#32639=CARTESIAN_POINT ( 'NONE',  ( 48.32499999726881157, 145.8408176439707802, 12.60653300113718345 ) ) ;
#32640=CARTESIAN_POINT ( 'NONE',  ( 60.87499999726879452, 138.6155565068815463, -3.929120461958505118E-15 ) ) ;
#32645=EDGE_CURVE ( 'NONE', #27342, #31940, #11740, .T. ) ;
#32648=CARTESIAN_POINT ( 'NONE',  ( 86.99999999453764588, 155.0000000000000000, 14.49999999999999467 ) ) ;
#32655=CARTESIAN_POINT ( 'NONE',  ( 71.47499999726879594, 160.0630714827496206, -15.58253175000000823 ) ) ;
#32659=CARTESIAN_POINT ( 'NONE',  ( 85.17499999726882720, 145.8408176439707802, -12.60653300113719588 ) ) ;
#32668=DIRECTION ( 'NONE',  ( 1.000000000000000000, 0.000000000000000000, 0.000000000000000000 ) ) ;
#32669=DIRECTION ( 'NONE',  ( 0.000000000000000000, 0.000000000000000000, 1.000000000000000000 ) ) ;
#32676=CARTESIAN_POINT ( 'NONE',  ( 42.52499999726880731, 140.1801316387863778, 4.815267126137185549 ) ) ;
#32677=CARTESIAN_POINT ( 'NONE',  ( 87.49999999999998579, 151.6435044740348417, -14.93273091701168909 ) ) ;
#32682=CARTESIAN_POINT ( 'NONE',  ( 32.50000000000000000, 155.0000000000000000, -6.938893903907228378E-15 ) ) ;
#32686=CARTESIAN_POINT ( 'NONE',  ( 63.89999999453763024, 150.2886644046228639, -14.50000000000000888 ) ) ;
#32687=ORIENTED_EDGE ( 'NONE', *, *, #13334, .T. ) ;
#32690=EDGE_CURVE ( 'NONE', #12765, #22989, #11915, .T. ) ;
#32692=EDGE_CURVE ( 'NONE', #3666, #1492, #18701, .T. ) ;
#32693=CARTESIAN_POINT ( 'NONE',  ( 76.11132485994281183, 169.2658477444273331, -4.635254915624224203 ) ) ;
#32697=ORIENTED_EDGE ( 'NONE', *, *, #26515, .T. ) ;
#32700=CARTESIAN_POINT ( 'NONE',  ( 42.18867513459481700, 140.7341522555726669, 4.635254915624211769 ) ) ;
#32706=CARTESIAN_POINT ( 'NONE',  ( 56.37499999726880873, 155.0000000000000000, 15.58253174999999402 ) ) ;
#32710=AXIS2_PLACEMENT_3D ( 'NONE', #5988, #3268, #19442 ) ;
#32714=CARTESIAN_POINT ( 'NONE',  ( 59.97499999726881015, 169.8198683612136222, 4.815267126137181997 ) ) ;
#32716=CYLINDRICAL_SURFACE ( 'NONE', #8860, 15.00000000000001776 ) ;
#32719=CARTESIAN_POINT ( 'NONE',  ( 77.79999999999999716, 142.6655632788954620, 8.961492836873471646 ) ) ;
#32724=CARTESIAN_POINT ( 'NONE',  ( 43.77499999726881441, 169.8198683612136222, -4.815267126137197984 ) ) ;
#32726=CARTESIAN_POINT ( 'NONE',  ( 86.32499999726880446, 145.8408176439707802, 12.60653300113718345 ) ) ;
#32729=CARTESIAN_POINT ( 'NONE',  ( 48.29999999453762882, 167.3344367211045096, -8.961492836873482304 ) ) ;
#32730=( BOUNDED_CURVE ( )  B_SPLINE_CURVE ( 2, ( #9891, #9719, #22323, #27267, #17043, #7165, #3924, #30332, #30167, #24720, #27437 ),
 .UNSPECIFIED., .F., .F. ) 
 B_SPLINE_CURVE_WITH_KNOTS ( ( 3, 2, 2, 2, 2, 3 ),
 ( 0.5892857142857140795, 0.5928571428571426383, 0.5964285714285711970, 0.5999999999999998668, 0.6035714285714284255, 0.6071428571428569843 ),
 .UNSPECIFIED. ) 
 CURVE ( )  GEOMETRIC_REPRESENTATION_ITEM ( )  RATIONAL_B_SPLINE_CURVE ( ( 1.000000000000003109, 0.9510565162951504226, 1.000000000000000000, 0.9510565162951534202, 1.000000000000000000, 0.9510565162951534202, 1.000000000000000000, 0.9510565162951534202, 1.000000000000000000, 0.9510565162951549745, 0.9999999999999984457 ) ) 
 REPRESENTATION_ITEM ( '' )  );
#32734=CARTESIAN_POINT ( 'NONE',  ( 32.50000000000000000, 155.0000000000000000, -6.938893903907228378E-15 ) ) ;
#32735=VERTEX_POINT ( 'NONE', #18210 ) ;
#32742=ORIENTED_EDGE ( 'NONE', *, *, #27884, .F. ) ;
#32748=VERTEX_POINT ( 'NONE', #10214 ) ;
#32749=CARTESIAN_POINT ( 'NONE',  ( 38.22499999726881015, 149.9369285172503510, 15.58253174999999580 ) ) ;
#32753=CARTESIAN_POINT ( 'NONE',  ( 40.47499999726881725, 149.9369285172503510, 15.58253174999999580 ) ) ;
#32758=CARTESIAN_POINT ( 'NONE',  ( 62.00000000000000000, 139.7537977485451393, -4.138211985947621020E-15 ) ) ;
#32764=CARTESIAN_POINT ( 'NONE',  ( 62.92499999726880588, 145.8408176439707802, -12.60653300113719588 ) ) ;
#32769=CARTESIAN_POINT ( 'NONE',  ( 83.57499999726880446, 164.1591823560292198, -12.60653300113719766 ) ) ;
#32772=DIRECTION ( 'NONE',  ( -1.000000000000000000, 0.000000000000000000, 0.000000000000000000 ) ) ;
#32782=CYLINDRICAL_SURFACE ( 'NONE', #18127, 15.00000000000001776 ) ;
#32787=EDGE_CURVE ( 'NONE', #3834, #31333, #9866, .T. ) ;
#32788=CARTESIAN_POINT ( 'NONE',  ( 81.02499999726880731, 149.9369285172503510, -15.58253175000000823 ) ) ;
#32793=CARTESIAN_POINT ( 'NONE',  ( 75.42499999726879878, 168.2552932293087906, -9.630534252274385310 ) ) ;
#32799=CARTESIAN_POINT ( 'NONE',  ( 42.30000000000000426, 146.4771138417591203, -11.73074641843674470 ) ) ;
#32803=CARTESIAN_POINT ( 'NONE',  ( 77.78867513459483973, 155.0000000000000000, 15.00000000000001243 ) ) ;
#32805=CARTESIAN_POINT ( 'NONE',  ( 47.82499999726881867, 168.2552932293087906, 9.630534252274372875 ) ) ;
#32806=CARTESIAN_POINT ( 'NONE',  ( 66.67499999726881299, 141.7447067706911810, 9.630534252274376428 ) ) ;
#32825=CARTESIAN_POINT ( 'NONE',  ( 72.17499999726881299, 164.1591823560292198, 12.60653300113718167 ) ) ;
#32829=CARTESIAN_POINT ( 'NONE',  ( 80.57499999726880446, 145.8408176439707802, 12.60653300113718345 ) ) ;
#32845=CARTESIAN_POINT ( 'NONE',  ( 67.08867513459482268, 167.7597621252805880, -9.270509831248443078 ) ) ;
#32849=CARTESIAN_POINT ( 'NONE',  ( 44.12499999726881583, 155.0000000000000000, 15.58253174999999402 ) ) ;
#32851=CARTESIAN_POINT ( 'NONE',  ( 34.72499999726881015, 140.1801316387863778, -4.815267126137194431 ) ) ;
#32854=EDGE_CURVE ( 'NONE', #9113, #8437, #17871, .T. ) ;
#32857=CARTESIAN_POINT ( 'NONE',  ( 76.08867513459483689, 142.2402378747194405, 9.270509831248432420 ) ) ;
#32862=CARTESIAN_POINT ( 'NONE',  ( 66.59999999453764019, 168.7903194862797420, 4.480746418436729606 ) ) ;
#32871=EDGE_LOOP ( 'NONE', ( #1827, #32097, #24950, #9711 ) ) ;
#32872=VECTOR ( 'NONE', #4048, 1000.000000000000000 ) ;
#32878=CARTESIAN_POINT ( 'NONE',  ( 84.71132485994282035, 155.0000000000000000, 15.00000000000001243 ) ) ;
#32880=CARTESIAN_POINT ( 'NONE',  ( 53.87499999726881583, 171.3844434931184253, -7.942151717890134290E-15 ) ) ;
#32887=CARTESIAN_POINT ( 'NONE',  ( 64.37499999726881583, 155.0000000000000000, 15.58253174999999402 ) ) ;
#32893=CARTESIAN_POINT ( 'NONE',  ( 79.19999999999998863, 167.3344367211045096, 8.961492836873468093 ) ) ;
#32897=CYLINDRICAL_SURFACE ( 'NONE', #16200, 15.00000000000001776 ) ;
#32898=CARTESIAN_POINT ( 'NONE',  ( 50.17499999726881299, 164.1591823560292198, 12.60653300113718167 ) ) ;
#32902=CARTESIAN_POINT ( 'NONE',  ( 84.42499999726881299, 141.7447067706911810, 9.630534252274376428 ) ) ;
#32903=LINE ( 'NONE', #6842, #31005 ) ;
#32905=CARTESIAN_POINT ( 'NONE',  ( 48.89999999453763735, 159.7113355953771077, 14.49999999999999289 ) ) ;
#32906=ORIENTED_EDGE ( 'NONE', *, *, #23457, .F. ) ;
#32922=CARTESIAN_POINT ( 'NONE',  ( 40.37499999726880873, 155.0000000000000000, 15.58253174999999402 ) ) ;
#32924=CARTESIAN_POINT ( 'NONE',  ( 45.92499999726881299, 164.1591823560292198, 12.60653300113718167 ) ) ;
#32926=CARTESIAN_POINT ( 'NONE',  ( 53.81132485994281467, 159.8737954434934920, -15.00000000000012434 ) ) ;
#32928=CARTESIAN_POINT ( 'NONE',  ( 49.17499999726881299, 145.8408176439707802, -12.60653300113719588 ) ) ;
#32929=CARTESIAN_POINT ( 'NONE',  ( 32.50000000000000000, 155.0000000000000000, -6.938893903907228378E-15 ) ) ;
#32932=CARTESIAN_POINT ( 'NONE',  ( 58.20000000000000284, 142.6655632788954620, -8.961492836873480528 ) ) ;
#32933=( BOUNDED_CURVE ( )  B_SPLINE_CURVE ( 2, ( #7730, #13006, #18452, #10459, #28839, #10299, #10787, #28670, #18615, #23561, #2618 ),
 .UNSPECIFIED., .F., .F. ) 
 B_SPLINE_CURVE_WITH_KNOTS ( ( 3, 2, 2, 2, 2, 3 ),
 ( 0.8750000000000000000, 0.8785714285714285587, 0.8821428571428571175, 0.8857142857142856762, 0.8892857142857142350, 0.8928571428571427937 ),
 .UNSPECIFIED. ) 
 CURVE ( )  GEOMETRIC_REPRESENTATION_ITEM ( )  RATIONAL_B_SPLINE_CURVE ( ( 1.000000000000000000, 0.9510565162951534202, 1.000000000000000000, 0.9510565162951534202, 1.000000000000000000, 0.9510565162951534202, 1.000000000000000000, 0.9510565162951534202, 1.000000000000000000, 0.9510565162951534202, 1.000000000000000000 ) ) 
 REPRESENTATION_ITEM ( '' )  );
#32938=CARTESIAN_POINT ( 'NONE',  ( 127.5000000000000000, 48.99999999999998579, -2.149999999999999023 ) ) ;
#32940=CARTESIAN_POINT ( 'NONE',  ( 64.82499999726881867, 141.7447067706911810, -9.630534252274385310 ) ) ;
#32944=CARTESIAN_POINT ( 'NONE',  ( 82.87499999726878741, 138.6155565068815463, -3.929120461958505118E-15 ) ) ;
#32963=CARTESIAN_POINT ( 'NONE',  ( 76.62499999726880162, 138.6155565068815463, -3.929120461958505118E-15 ) ) ;
#32967=CARTESIAN_POINT ( 'NONE',  ( 40.10000000000000142, 141.2096805137202580, -4.480746418436742040 ) ) ;
#32972=LINE ( 'NONE', #29753, #18071 ) ;
#32973=CARTESIAN_POINT ( 'NONE',  ( 49.02499999726880731, 149.9369285172503510, -15.58253175000000823 ) ) ;
#32974=CARTESIAN_POINT ( 'NONE',  ( 64.17499999726879878, 164.1591823560292198, 12.60653300113718167 ) ) ;
#32976=FACE_OUTER_BOUND ( 'NONE', #21017, .T. ) ;
#32985=CARTESIAN_POINT ( 'NONE',  ( 73.98867513459481415, 146.1832212156128890, 12.13525491562421976 ) ) ;
#32992=CARTESIAN_POINT ( 'NONE',  ( 75.97499999726881015, 169.8198683612136222, 4.815267126137181997 ) ) ;
#32994=ORIENTED_EDGE ( 'NONE', *, *, #1015, .F. ) ;
#32996=CARTESIAN_POINT ( 'NONE',  ( 81.67499999726884141, 168.2552932293087906, -9.630534252274387086 ) ) ;
#32999=CARTESIAN_POINT ( 'NONE',  ( 56.82499999726880446, 141.7447067706911810, -9.630534252274385310 ) ) ;
#33002=ORIENTED_EDGE ( 'NONE', *, *, #13220, .T. ) ;
#33003=CIRCLE ( 'NONE', #15598, 70.00000000000000000 ) ;
#33012=CARTESIAN_POINT ( 'NONE',  ( 52.52499999726881441, 140.1801316387863778, 4.815267126137185549 ) ) ;
#33014=CARTESIAN_POINT ( 'NONE',  ( 87.50000000000002842, 145.7452232778646817, -11.80462230752951136 ) ) ;
#33026=CARTESIAN_POINT ( 'NONE',  ( 74.49999999453764588, 170.2462022514548323, -7.872454543227099337E-15 ) ) ;
#33037=VERTEX_POINT ( 'NONE', #6909 ) ;
#33038=CARTESIAN_POINT ( 'NONE',  ( 58.68867513459483121, 150.1262045565064227, -15.00000000000002665 ) ) ;
#33043=CARTESIAN_POINT ( 'NONE',  ( 55.41132485994280898, 142.2402378747194405, -9.270509831248439525 ) ) ;
#33046=CARTESIAN_POINT ( 'NONE',  ( 58.07499999726880446, 168.2552932293087906, 9.630534252274372875 ) ) ;
#33054=CARTESIAN_POINT ( 'NONE',  ( 66.57499999726881867, 145.8408176439707802, 12.60653300113718345 ) ) ;
#33059=CARTESIAN_POINT ( 'NONE',  ( 80.80000000000001137, 167.3344367211045096, -8.961492836873482304 ) ) ;
#33064=CARTESIAN_POINT ( 'NONE',  ( 50.07499999726881157, 168.2552932293087906, 9.630534252274372875 ) ) ;
#33067=CARTESIAN_POINT ( 'NONE',  ( 82.72499999726881015, 140.1801316387863778, -4.815267126137194431 ) ) ;
#33069=CARTESIAN_POINT ( 'NONE',  ( 64.81132485994280046, 150.1262045565066785, 15.00000000000020250 ) ) ;
#33070=CARTESIAN_POINT ( 'NONE',  ( 52.69999999453762740, 167.3344367211045096, 8.961492836873468093 ) ) ;
#33073=CIRCLE ( 'NONE', #26543, 98.00000000000002842 ) ;
#33078=VERTEX_POINT ( 'NONE', #1790 ) ;
#33082=( BOUNDED_CURVE ( )  B_SPLINE_CURVE ( 2, ( #30152, #11424, #9200, #27580, #32693, #9361, #29984, #11925, #6983, #14644, #27253 ),
 .UNSPECIFIED., .F., .T. ) 
 B_SPLINE_CURVE_WITH_KNOTS ( ( 3, 2, 2, 2, 2, 3 ),
 ( 0.7500000000000000000, 0.7535714285714285587, 0.7571428571428571175, 0.7607142857142855652, 0.7642857142857141239, 0.7678571428571427937 ),
 .UNSPECIFIED. ) 
 CURVE ( )  GEOMETRIC_REPRESENTATION_ITEM ( )  RATIONAL_B_SPLINE_CURVE ( ( 1.000000000000000000, 0.9510565162951534202, 1.000000000000000000, 0.9510565162951534202, 1.000000000000000000, 0.9510565162951534202, 1.000000000000000000, 0.9510565162951534202, 1.000000000000000000, 0.9510565162951549745, 0.9999999999999984457 ) ) 
 REPRESENTATION_ITEM ( '' )  );
#33087=CARTESIAN_POINT ( 'NONE',  ( 49.98867513459481415, 146.1832212156128890, 12.13525491562421976 ) ) ;
#33088=ORIENTED_EDGE ( 'NONE', *, *, #7298, .T. ) ;
#33093=CARTESIAN_POINT ( 'NONE',  ( 38.47499999726881015, 149.9369285172503510, 15.58253174999999580 ) ) ;
#33095=CARTESIAN_POINT ( 'NONE',  ( 44.32499999726881157, 145.8408176439707802, 12.60653300113718345 ) ) ;
#33099=EDGE_CURVE ( 'NONE', #30928, #8859, #12704, .T. ) ;
#33100=CARTESIAN_POINT ( 'NONE',  ( 46.27499999726881441, 160.0630714827496206, 15.58253174999999402 ) ) ;
#33106=CARTESIAN_POINT ( 'NONE',  ( 63.29999999999999716, 163.5228861582408797, 11.73074641843673049 ) ) ;
#33111=CARTESIAN_POINT ( 'NONE',  ( 34.47499999726881015, 149.9369285172503510, 15.58253174999999580 ) ) ;
#33114=CARTESIAN_POINT ( 'NONE',  ( 61.12499999726880873, 155.0000000000000000, -15.58253175000000823 ) ) ;
#33116=EDGE_LOOP ( 'NONE', ( #11799, #1231 ) ) ;
#33117=CARTESIAN_POINT ( 'NONE',  ( 86.78867513459481131, 155.0000000000000000, -15.00000000000002487 ) ) ;
#33118=CARTESIAN_POINT ( 'NONE',  ( 86.87499999726880162, 138.6155565068815463, -3.929120461958505118E-15 ) ) ;
#33120=DIRECTION ( 'NONE',  ( 1.000000000000000000, 0.000000000000000000, 0.000000000000000000 ) ) ;
#33125=LINE ( 'NONE', #22566, #155 ) ;
#33130=EDGE_CURVE ( 'NONE', #12310, #2726, #1276, .T. ) ;
#33138=ORIENTED_EDGE ( 'NONE', *, *, #32645, .T. ) ;
#33141=AXIS2_PLACEMENT_3D ( 'NONE', #7520, #2403, #33234 ) ;
#33142=FACE_OUTER_BOUND ( 'NONE', #6986, .T. ) ;
#33145=CARTESIAN_POINT ( 'NONE',  ( 73.47499999726879594, 160.0630714827496206, -15.58253175000000823 ) ) ;
#33146=CARTESIAN_POINT ( 'NONE',  ( 81.92499999726882720, 164.1591823560292198, 12.60653300113718167 ) ) ;
#33151=CARTESIAN_POINT ( 'NONE',  ( 44.10000000000000142, 141.2096805137202580, -4.480746418436742040 ) ) ;
#33153=VECTOR ( 'NONE', #21007, 1000.000000000000000 ) ;
#33157=CARTESIAN_POINT ( 'NONE',  ( 60.02499999726881441, 160.0630714827496206, 15.58253174999999224 ) ) ;
#33158=CARTESIAN_POINT ( 'NONE',  ( 63.17499999726880588, 145.8408176439707802, -12.60653300113719588 ) ) ;
#33168=CARTESIAN_POINT ( 'NONE',  ( 68.11132485994281183, 169.2658477444273331, -4.635254915624224203 ) ) ;
#33175=CARTESIAN_POINT ( 'NONE',  ( 75.07499999726879025, 141.7447067706911810, -9.630534252274385310 ) ) ;
#33178=VERTEX_POINT ( 'NONE', #29917 ) ;
#33179=ADVANCED_FACE ( 'NONE', ( #14409 ), #24802, .T. ) ;
#33180=CARTESIAN_POINT ( 'NONE',  ( 68.72499999726881015, 140.1801316387863778, -4.815267126137194431 ) ) ;
#33183=CARTESIAN_POINT ( 'NONE',  ( 62.82499999726881867, 141.7447067706911810, -9.630534252274385310 ) ) ;
#33189=CARTESIAN_POINT ( 'NONE',  ( 86.41132485994282320, 167.7597621252805880, 9.270509831248428867 ) ) ;
#33197=CARTESIAN_POINT ( 'NONE',  ( 37.52499999726881441, 169.8198683612136222, -4.815267126137197984 ) ) ;
#33204=CARTESIAN_POINT ( 'NONE',  ( 54.48867513459482836, 142.2402378747194405, -9.270509831248439525 ) ) ;
#33207=CARTESIAN_POINT ( 'NONE',  ( 72.79999999453762882, 163.5228861582408797, 11.73074641843673049 ) ) ;
#33216=ORIENTED_EDGE ( 'NONE', *, *, #14492, .T. ) ;
#33221=CARTESIAN_POINT ( 'NONE',  ( 55.11132485994280472, 140.7341522555726669, 4.635254915624211769 ) ) ;
#33224=CARTESIAN_POINT ( 'NONE',  ( 59.47499999726880304, 160.0630714827496206, -15.58253175000000823 ) ) ;
#33228=CARTESIAN_POINT ( 'NONE',  ( 57.01132485994281041, 142.2402378747194405, 9.270509831248432420 ) ) ;
#33230=CARTESIAN_POINT ( 'NONE',  ( 67.67499999726881299, 168.2552932293087906, -9.630534252274385310 ) ) ;
#33234=DIRECTION ( 'NONE',  ( 0.000000000000000000, 0.000000000000000000, -1.000000000000000000 ) ) ;
#33237=CARTESIAN_POINT ( 'NONE',  ( 86.79999999999998295, 167.3344367211045096, -8.961492836873482304 ) ) ;
#33242=CARTESIAN_POINT ( 'NONE',  ( 53.87499999726881583, 171.3844434931184253, -7.942151717890132712E-15 ) ) ;
#33244=CARTESIAN_POINT ( 'NONE',  ( 87.32499999726880446, 164.1591823560292198, -12.60653300113719766 ) ) ;
#33245=CARTESIAN_POINT ( 'NONE',  ( 52.11132485994280472, 169.2658477444273331, -4.635254915624224203 ) ) ;
#33247=CARTESIAN_POINT ( 'NONE',  ( 55.09999999453761887, 150.2886644046228639, 14.49999999999999645 ) ) ;
#33253=ORIENTED_EDGE ( 'NONE', *, *, #24584, .F. ) ;
#33263=ADVANCED_FACE ( 'NONE', ( #261, #22919 ), #2309, .F. ) ;
#33265=CARTESIAN_POINT ( 'NONE',  ( 38.37499999726880873, 155.0000000000000000, 15.58253174999999402 ) ) ;
#33266=VERTEX_POINT ( 'NONE', #25818 ) ;
#33267=CARTESIAN_POINT ( 'NONE',  ( 41.32499999726881157, 164.1591823560292198, -12.60653300113719766 ) ) ;
#33271=CARTESIAN_POINT ( 'NONE',  ( 45.47499999726881015, 160.0630714827496206, -15.58253175000000823 ) ) ;
#33276=CARTESIAN_POINT ( 'NONE',  ( 66.29999999999999716, 146.4771138417591203, -11.73074641843674470 ) ) ;
#33278=CARTESIAN_POINT ( 'NONE',  ( 63.91132485994280188, 163.8167787843871110, -12.13525491562423397 ) ) ;
#33280=DIRECTION ( 'NONE',  ( 1.000000000000000000, 0.000000000000000000, 0.000000000000000000 ) ) ;
#33283=CARTESIAN_POINT ( 'NONE',  ( 63.82499999726881867, 168.2552932293087906, 9.630534252274372875 ) ) ;
#33288=CARTESIAN_POINT ( 'NONE',  ( 34.69999999453763451, 167.3344367211045096, 8.961492836873468093 ) ) ;
#33291=( BOUNDED_CURVE ( )  B_SPLINE_CURVE ( 2, ( #1408, #29690, #13675, #29363, #6347, #16398, #26792, #3455, #33087, #14516, #12638 ),
 .UNSPECIFIED., .F., .F. ) 
 B_SPLINE_CURVE_WITH_KNOTS ( ( 3, 2, 2, 2, 2, 3 ),
 ( 0.6607142857142855874, 0.6642857142857142572, 0.6678571428571427049, 0.6714285714285712636, 0.6749999999999997113, 0.6785714285714283811 ),
 .UNSPECIFIED. ) 
 CURVE ( )  GEOMETRIC_REPRESENTATION_ITEM ( )  RATIONAL_B_SPLINE_CURVE ( ( 1.000000000000000000, 0.9510565162951534202, 1.000000000000000000, 0.9510565162951534202, 1.000000000000000000, 0.9510565162951534202, 1.000000000000000000, 0.9510565162951534202, 1.000000000000000000, 0.9510565162951564178, 0.9999999999999970024 ) ) 
 REPRESENTATION_ITEM ( '' )  );
#33304=CARTESIAN_POINT ( 'NONE',  ( 70.51132485994280330, 163.8167787843871110, 12.13525491562421621 ) ) ;
#33307=CARTESIAN_POINT ( 'NONE',  ( 34.01132485994281041, 167.7597621252805880, -9.270509831248443078 ) ) ;
#33310=CARTESIAN_POINT ( 'NONE',  ( 84.02499999726882152, 160.0630714827496206, 15.58253174999999402 ) ) ;
#33313=DIRECTION ( 'NONE',  ( 0.000000000000000000, 1.000000000000000000, -1.224646799147353207E-16 ) ) ;
#33316=CARTESIAN_POINT ( 'NONE',  ( 42.89999999999999858, 168.7903194862797420, -4.480746418436745593 ) ) ;
#33323=CARTESIAN_POINT ( 'NONE',  ( 55.32499999726881157, 164.1591823560292198, -12.60653300113719766 ) ) ;
#33324=CARTESIAN_POINT ( 'NONE',  ( 69.97499999726881015, 169.8198683612136222, 4.815267126137181997 ) ) ;
#33335=CARTESIAN_POINT ( 'NONE',  ( 73.88867513459481984, 150.1262045565060248, 14.99999999999975842 ) ) ;
#33337=ADVANCED_FACE ( 'NONE', ( #28703 ), #10656, .F. ) ;
#33345=CARTESIAN_POINT ( 'NONE',  ( 80.47499999726881015, 149.9369285172503510, 15.58253174999999580 ) ) ;
#33349=CARTESIAN_POINT ( 'NONE',  ( 70.22499999726879594, 149.9369285172503510, 15.58253174999999580 ) ) ;
#33352=CARTESIAN_POINT ( 'NONE',  ( 65.82499999726881867, 168.2552932293087906, 9.630534252274372875 ) ) ;
#33363=DIRECTION ( 'NONE',  ( 0.000000000000000000, 0.000000000000000000, -1.000000000000000000 ) ) ;
#33370=CARTESIAN_POINT ( 'NONE',  ( 38.12499999726880873, 155.0000000000000000, 15.58253174999999402 ) ) ;
#33379=CARTESIAN_POINT ( 'NONE',  ( 76.19999999453763451, 163.5228861582408797, -11.73074641843674470 ) ) ;
#33387=ORIENTED_EDGE ( 'NONE', *, *, #10237, .F. ) ;
#33390=CARTESIAN_POINT ( 'NONE',  ( 51.18867513459482410, 169.2658477444273331, -4.635254915624224203 ) ) ;
#33392=ORIENTED_EDGE ( 'NONE', *, *, #9725, .T. ) ;
#33399=CARTESIAN_POINT ( 'NONE',  ( 58.67499999726880588, 141.7447067706911810, 9.630534252274376428 ) ) ;
#33404=CARTESIAN_POINT ( 'NONE',  ( 63.77499999726880731, 169.8198683612136222, -4.815267126137197984 ) ) ;
#33407=DIRECTION ( 'NONE',  ( 1.000000000000000000, 0.000000000000000000, 0.000000000000000000 ) ) ;
#33409=CARTESIAN_POINT ( 'NONE',  ( 34.52499999726880731, 140.1801316387863778, 4.815267126137185549 ) ) ;
#33411=CARTESIAN_POINT ( 'NONE',  ( 125.5000000000000000, 228.4330392262239116, 76.47359838532422316 ) ) ;
#33414=CARTESIAN_POINT ( 'NONE',  ( 49.07499999726880446, 141.7447067706911810, -9.630534252274385310 ) ) ;
#33419=CARTESIAN_POINT ( 'NONE',  ( 55.99999999453762456, 155.0000000000000000, -14.50000000000000711 ) ) ;
#33429=ORIENTED_EDGE ( 'NONE', *, *, #12430, .F. ) ;
#33436=CARTESIAN_POINT ( 'NONE',  ( 37.77499999726881441, 169.8198683612136222, -4.815267126137197984 ) ) ;
#33438=CARTESIAN_POINT ( 'NONE',  ( 47.02499999726881441, 149.9369285172503510, -15.58253175000000823 ) ) ;
#33443=CARTESIAN_POINT ( 'NONE',  ( 44.77499999726881441, 140.1801316387863778, 4.815267126137185549 ) ) ;
#33446=CARTESIAN_POINT ( 'NONE',  ( 58.71132485994280614, 155.0000000000000000, 15.00000000000001243 ) ) ;
#33447=CARTESIAN_POINT ( 'NONE',  ( 69.60000000000000853, 150.2886644046228639, 14.49999999999999645 ) ) ;
#33454=CARTESIAN_POINT ( 'NONE',  ( 67.62499999726881583, 171.3844434931184253, -7.942151717890132712E-15 ) ) ;
#33457=CARTESIAN_POINT ( 'NONE',  ( 36.99999999453763166, 155.0000000000000000, 14.49999999999999467 ) ) ;
#33472=LINE ( 'NONE', #7412, #32507 ) ;
#33474=ORIENTED_EDGE ( 'NONE', *, *, #27431, .F. ) ;
#33476=ORIENTED_EDGE ( 'NONE', *, *, #11256, .T. ) ;
#33477=CARTESIAN_POINT ( 'NONE',  ( 81.61132485994282604, 150.1262045565065364, -15.00000000000012434 ) ) ;
#33479=CARTESIAN_POINT ( 'NONE',  ( 83.52499999726880731, 169.8198683612136222, -4.815267126137197984 ) ) ;
#33483=DIRECTION ( 'NONE',  ( 0.000000000000000000, 0.000000000000000000, -1.000000000000000000 ) ) ;
#33484=CARTESIAN_POINT ( 'NONE',  ( 50.50000000000000000, 155.0000000000000000, -14.50000000000000711 ) ) ;
#33486=CARTESIAN_POINT ( 'NONE',  ( 71.51132485994280330, 146.1832212156128890, -12.13525491562423042 ) ) ;
#33491=CARTESIAN_POINT ( 'NONE',  ( 59.02499999726880731, 149.9369285172503510, -15.58253175000000823 ) ) ;
#33492=CARTESIAN_POINT ( 'NONE',  ( 72.67499999726881299, 141.7447067706911810, 9.630534252274376428 ) ) ;
#33494=CYLINDRICAL_SURFACE ( 'NONE', #28767, 15.00000000000001776 ) ;
#33508=CARTESIAN_POINT ( 'NONE',  ( 80.97499999726881015, 140.1801316387863778, -4.815267126137194431 ) ) ;
#33512=CARTESIAN_POINT ( 'NONE',  ( 73.02499999726882152, 149.9369285172503510, -15.58253175000000823 ) ) ;
#33515=CARTESIAN_POINT ( 'NONE',  ( 66.62499999726881583, 138.6155565068815463, -3.929120461958505118E-15 ) ) ;
#33524=( BOUNDED_CURVE ( )  B_SPLINE_CURVE ( 2, ( #10627, #5001, #2952, #387, #3107, #21002, #10790, #8069, #25946, #10301, #31400 ),
 .UNSPECIFIED., .F., .T. ) 
 B_SPLINE_CURVE_WITH_KNOTS ( ( 3, 2, 2, 2, 2, 3 ),
 ( 0.01785714285714287350, 0.02142857142857142530, 0.02499999999999997710, 0.02857142857142853237, 0.03214285714285719520, 0.03571428571428574700 ),
 .UNSPECIFIED. ) 
 CURVE ( )  GEOMETRIC_REPRESENTATION_ITEM ( )  RATIONAL_B_SPLINE_CURVE ( ( 0.9999999999999988898, 0.9510565162951545304, 1.000000000000000000, 0.9510565162951534202, 1.000000000000000000, 0.9510565162951534202, 1.000000000000000000, 0.9510565162951534202, 1.000000000000000000, 0.9510565162951527540, 1.000000000000000666 ) ) 
 REPRESENTATION_ITEM ( '' )  );
#33528=CARTESIAN_POINT ( 'NONE',  ( 117.5000000000000142, 155.0000000000000000, -70.00000000000002842 ) ) ;
#33532=CARTESIAN_POINT ( 'NONE',  ( 45.78867513459482552, 155.0000000000000000, 15.00000000000001243 ) ) ;
#33533=CARTESIAN_POINT ( 'NONE',  ( 32.50000000000000000, 155.0000000000000000, 15.00000000000001243 ) ) ;
#33534=CARTESIAN_POINT ( 'NONE',  ( 41.12499999726880873, 155.0000000000000000, -15.58253175000000823 ) ) ;
#33542=CARTESIAN_POINT ( 'NONE',  ( 71.19999999453763451, 146.4771138417591203, 11.73074641843673227 ) ) ;
#33543=ORIENTED_EDGE ( 'NONE', *, *, #13907, .F. ) ;
#33552=ORIENTED_EDGE ( 'NONE', *, *, #24122, .T. ) ;
#33553=ORIENTED_EDGE ( 'NONE', *, *, #8366, .F. ) ;
#33555=VECTOR ( 'NONE', #27228, 1000.000000000000000 ) ;
#33556=CARTESIAN_POINT ( 'NONE',  ( 51.28867513459482552, 170.7719333635740497, -7.904646289410545231E-15 ) ) ;
#33557=CARTESIAN_POINT ( 'NONE',  ( 56.38867513459481984, 140.7341522555726669, -4.635254915624220651 ) ) ;
#33563=CARTESIAN_POINT ( 'NONE',  ( 59.97499999726881015, 169.8198683612136222, 4.815267126137181997 ) ) ;
#33576=CARTESIAN_POINT ( 'NONE',  ( 34.62499999726880873, 138.6155565068815463, -3.929120461958505118E-15 ) ) ;
#33581=CARTESIAN_POINT ( 'NONE',  ( 52.67499999726880588, 141.7447067706911810, 9.630534252274376428 ) ) ;
#33583=VECTOR ( 'NONE', #589, 1000.000000000000000 ) ;
#33584=FACE_OUTER_BOUND ( 'NONE', #13626, .T. ) ;
#33585=CARTESIAN_POINT ( 'NONE',  ( 52.21132485994282035, 170.7719333635740497, -7.904646289410545231E-15 ) ) ;
#33587=CARTESIAN_POINT ( 'NONE',  ( 56.69999999453763451, 167.3344367211045096, 8.961492836873468093 ) ) ;
#33602=CARTESIAN_POINT ( 'NONE',  ( 79.67499999726881299, 168.2552932293087906, -9.630534252274387086 ) ) ;
#33606=CARTESIAN_POINT ( 'NONE',  ( 34.57499999726881157, 145.8408176439707802, 12.60653300113718345 ) ) ;
#33608=CARTESIAN_POINT ( 'NONE',  ( 41.52499999726881441, 169.8198683612136222, -4.815267126137197984 ) ) ;
#33612=CARTESIAN_POINT ( 'NONE',  ( 45.57499999726881157, 164.1591823560292198, -12.60653300113719766 ) ) ;
#33616=CARTESIAN_POINT ( 'NONE',  ( 70.29999999999999716, 146.4771138417591203, -11.73074641843674470 ) ) ;
#33625=CARTESIAN_POINT ( 'NONE',  ( 72.32499999726880446, 145.8408176439707802, 12.60653300113718345 ) ) ;
#33626=ORIENTED_EDGE ( 'NONE', *, *, #20817, .T. ) ;
#33628=CARTESIAN_POINT ( 'NONE',  ( 36.39999999453763024, 168.7903194862797420, -4.480746418436745593 ) ) ;
#33632=ORIENTED_EDGE ( 'NONE', *, *, #16386, .T. ) ;
#33643=ORIENTED_EDGE ( 'NONE', *, *, #9297, .T. ) ;
#33648=CARTESIAN_POINT ( 'NONE',  ( 84.42499999726881299, 141.7447067706911810, 9.630534252274376428 ) ) ;
#33655=CARTESIAN_POINT ( 'NONE',  ( 49.89999999999999858, 141.2096805137202580, 4.480746418436733158 ) ) ;
#33657=CARTESIAN_POINT ( 'NONE',  ( 84.01132485994281751, 167.7597621252805880, -9.270509831248443078 ) ) ;
#33660=CARTESIAN_POINT ( 'NONE',  ( 54.02499999726880020, 160.0630714827496206, 15.58253174999999402 ) ) ;
#33663=CARTESIAN_POINT ( 'NONE',  ( 56.22499999726882436, 149.9369285172503510, 15.58253174999999580 ) ) ;
#33664=CARTESIAN_POINT ( 'NONE',  ( 72.87499999726881583, 138.6155565068815463, -3.929120461958505118E-15 ) ) ;
#33682=CARTESIAN_POINT ( 'NONE',  ( 79.37499999726881583, 155.0000000000000000, -15.58253175000000823 ) ) ;
#33686=CARTESIAN_POINT ( 'NONE',  ( 71.22499999726879594, 160.0630714827496206, -15.58253175000000823 ) ) ;
#33687=ORIENTED_EDGE ( 'NONE', *, *, #32425, .F. ) ;
ENDSEC;
END-ISO-10303-21;
